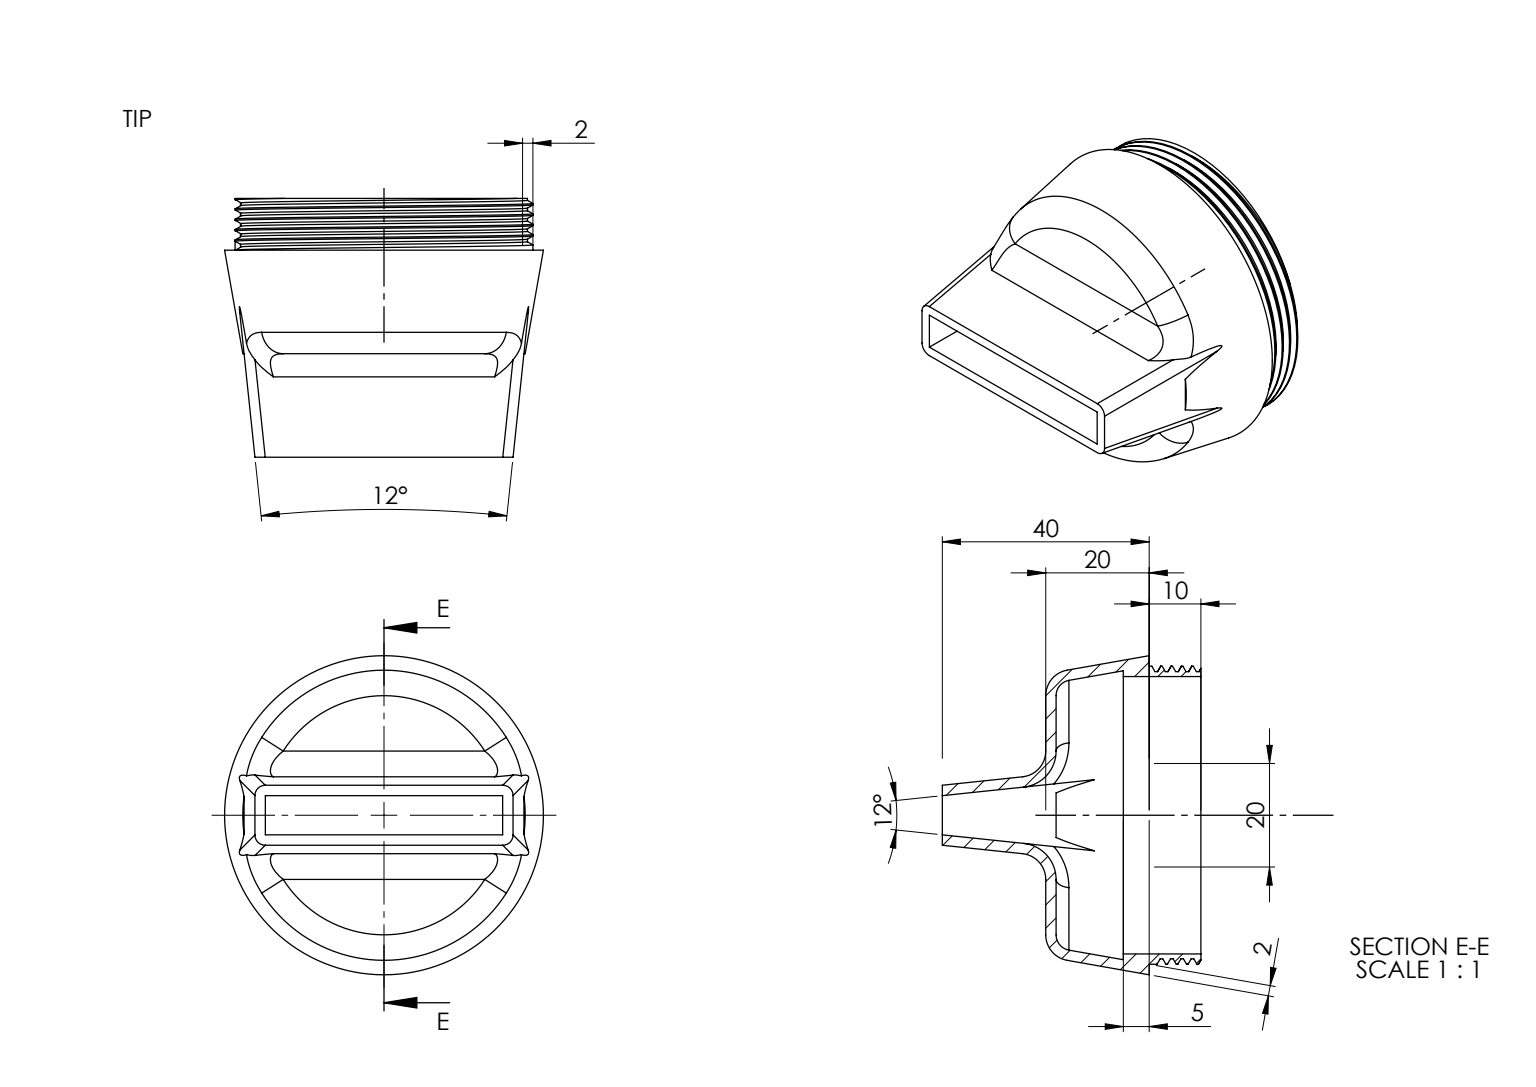
ISO-10303-21;
HEADER;
FILE_DESCRIPTION (('STEP AP214'),
    '1' );
FILE_NAME ('tip.step',
    '2026-10-04T13:31:42',
    ( '' ),
    ( '' ),
    'SwSTEP 2.0',
    'SolidWorks 2026',
    '' );
FILE_SCHEMA (( 'AUTOMOTIVE_DESIGN' ));
ENDSEC;

DATA;
#60=CARTESIAN_POINT ( 'NONE',  ( -8.571926809382608425, 26.38167802310805854, 144.4750000027312069 ) ) ;
#72=( BOUNDED_CURVE ( )  B_SPLINE_CURVE ( 2, ( #135553, #193227, #149715, #197225, #132546, #194235, #55701, #58687, #117374, #179071, #182049 ),
 .UNSPECIFIED., .F., .T. ) 
 B_SPLINE_CURVE_WITH_KNOTS ( ( 3, 2, 2, 2, 2, 3 ),
 ( 0.1000000000000000888, 0.1200000000000001343, 0.1400000000000001799, 0.1600000000000001976, 0.1800000000000002431, 0.2000000000000001776 ),
 .UNSPECIFIED. ) 
 CURVE ( )  GEOMETRIC_REPRESENTATION_ITEM ( )  RATIONAL_B_SPLINE_CURVE ( ( 0.9999999999999997780, 0.9510565162951537532, 1.000000000000000000, 0.9510565162951535312, 1.000000000000000000, 0.9510565162951535312, 1.000000000000000000, 0.9510565162951535312, 1.000000000000000000, 0.9510565162951529761, 1.000000000000000444 ) ) 
 REPRESENTATION_ITEM ( '' )  );
#75=CARTESIAN_POINT ( 'NONE',  ( 27.73933785331498569, 2.768321779492822058E-14, 140.3750000027311842 ) ) ;
#93=CARTESIAN_POINT ( 'NONE',  ( 25.38276140623240096, 4.833717845876353891, 166.7901960806512136 ) ) ;
#101=CARTESIAN_POINT ( 'NONE',  ( 28.79475375365586132, 2.781246896534039337E-14, 145.2656553485623760 ) ) ;
#142=CARTESIAN_POINT ( 'NONE',  ( 1.955436445514509014, -27.87083070116242567, 139.9999999999999716 ) ) ;
#200=CARTESIAN_POINT ( 'NONE',  ( -23.31738231874055245, -16.94106989632524574, 144.1999999999999886 ) ) ;
#216=CARTESIAN_POINT ( 'NONE',  ( 23.29544513554940011, 16.92513159979228021, 143.4656553485623647 ) ) ;
#218=CARTESIAN_POINT ( 'NONE',  ( 19.76513836702801186, -12.18681594171306237, 170.0000000000000000 ) ) ;
#300=ORIENTED_EDGE ( 'NONE', *, *, #146255, .F. ) ;
#338=CARTESIAN_POINT ( 'NONE',  ( -30.82560697742735911, 2.051108057200722688E-14, 150.0000000000000000 ) ) ;
#460=CARTESIAN_POINT ( 'NONE',  ( 27.74036206688027661, 1.797278685356906491, 140.0000000000000000 ) ) ;
#486=CARTESIAN_POINT ( 'NONE',  ( 21.65431292632186100, -8.856125861401146437, 168.9593721673316793 ) ) ;
#544=CARTESIAN_POINT ( 'NONE',  ( -17.14385361876520619, 23.59649016807275856, 143.0750000027311444 ) ) ;
#548=CARTESIAN_POINT ( 'NONE',  ( -17.14385361876520264, -23.59649016807271593, 143.6750000027311671 ) ) ;
#553=DIRECTION ( 'NONE',  ( -0.000000000000000000, -0.000000000000000000, -1.000000000000000000 ) ) ;
#581=CARTESIAN_POINT ( 'NONE',  ( -24.42783677680811749, -12.30119602009749613, 169.8172178118632587 ) ) ;
#601=CARTESIAN_POINT ( 'NONE',  ( -17.79613651744293890, -24.49428055684528260, 140.5656553485623022 ) ) ;
#766=CARTESIAN_POINT ( 'NONE',  ( -24.20533859822809220, -9.236745700548658178, 166.4300890397318540 ) ) ;
#827=CARTESIAN_POINT ( 'NONE',  ( -23.91168844458654164, 8.792376985861425354, 168.9858545422794975 ) ) ;
#852=ORIENTED_EDGE ( 'NONE', *, *, #79706, .T. ) ;
#865=DIRECTION ( 'NONE',  ( -1.000000000000000000, 0.000000000000000000, 0.000000000000000000 ) ) ;
#891=CARTESIAN_POINT ( 'NONE',  ( 1.784210473542230573E-15, -29.16686587814331588, 147.3750000027311842 ) ) ;
#978=CARTESIAN_POINT ( 'NONE',  ( -25.28179187713397269, -11.97099003546684415, 166.1915553108511290 ) ) ;
#1014=CARTESIAN_POINT ( 'NONE',  ( -3.573655867282028392E-15, 2.428612866367529932E-14, 139.9999999999999716 ) ) ;
#1025=( NAMED_UNIT ( * ) PLANE_ANGLE_UNIT ( ) SI_UNIT ( $, .RADIAN. ) );
#1054=CARTESIAN_POINT ( 'NONE',  ( 27.73933785331498214, 9.013057229001095294, 145.9750000027311785 ) ) ;
#1061=CARTESIAN_POINT ( 'NONE',  ( 20.69372460268722236, -10.84650605405300539, 168.1714143675833668 ) ) ;
#1191=CARTESIAN_POINT ( 'NONE',  ( -17.81289503416611808, 24.51734667627700404, 143.7000000000000171 ) ) ;
#1204=CARTESIAN_POINT ( 'NONE',  ( 24.18299921989822820, -12.77492350451709235, 169.7822198539309966 ) ) ;
#1210=CARTESIAN_POINT ( 'NONE',  ( 21.34799762026584702, -10.44447989802409893, 170.3878604776606096 ) ) ;
#1214=CARTESIAN_POINT ( 'NONE',  ( -24.74823625077143774, 6.005039613785521091, 168.8763313249075964 ) ) ;
#1293=ORIENTED_EDGE ( 'NONE', *, *, #171007, .T. ) ;
#1305=CARTESIAN_POINT ( 'NONE',  ( 1.784210473542230573E-15, -29.16686587814331588, 147.8750000027311273 ) ) ;
#1326=CARTESIAN_POINT ( 'NONE',  ( -25.66012929990208136, -7.783344152590475851, 170.2244316400881701 ) ) ;
#1457=CARTESIAN_POINT ( 'NONE',  ( 27.38287604894768634, -4.524378969001820572, 139.9999999999999716 ) ) ;
#1479=AXIS2_PLACEMENT_3D ( 'NONE', #153769, #105284, #28475 ) ;
#1535=EDGE_CURVE ( 'NONE', #136214, #11685, #2227, .T. ) ;
#1547=CARTESIAN_POINT ( 'NONE',  ( 22.44159573604009239, 16.30477369853692693, 148.5750000027312012 ) ) ;
#1657=VECTOR ( 'NONE', #198444, 1000.000000000000000 ) ;
#1779=ADVANCED_FACE ( 'NONE', ( #62900 ), #3223, .T. ) ;
#1806=CARTESIAN_POINT ( 'NONE',  ( -8.898068258721474777, 27.38543819252877043, 145.5843446569000150 ) ) ;
#1831=CARTESIAN_POINT ( 'NONE',  ( -21.70479006154311108, 8.695791278452229989, 169.0563666577074287 ) ) ;
#1897=CARTESIAN_POINT ( 'NONE',  ( 8.571926809382603096, -26.38167802310801235, 139.4750000027311785 ) ) ;
#2037=PLANE ( 'NONE',  #40540 ) ;
#2061=CARTESIAN_POINT ( 'NONE',  ( -27.73933785331498925, 2.428612866367529932E-14, 140.8750000027311842 ) ) ;
#2068=FACE_OUTER_BOUND ( 'NONE', #96703, .T. ) ;
#2128=EDGE_CURVE ( 'NONE', #35378, #51307, #33569, .T. ) ;
#2143=EDGE_CURVE ( 'NONE', #18425, #66087, #76032, .T. ) ;
#2198=CARTESIAN_POINT ( 'NONE',  ( -5.429308488886486681E-15, 30.30510711980690175, 143.4999999999999432 ) ) ;
#2211=CARTESIAN_POINT ( 'NONE',  ( 25.86526910843990379, -7.630673861715740358, 173.3900163844746771 ) ) ;
#2227=LINE ( 'NONE', #170091, #198734 ) ;
#2291=CARTESIAN_POINT ( 'NONE',  ( -5.429308488886486681E-15, 30.30510711980690175, 147.7500000054623683 ) ) ;
#2429=AXIS2_PLACEMENT_3D ( 'NONE', #118960, #58273, #120921 ) ;
#2459=CARTESIAN_POINT ( 'NONE',  ( 18.35237201590196676, -20.87933371662905202, 140.0000000000000284 ) ) ;
#2548=CARTESIAN_POINT ( 'NONE',  ( -28.79475375365586842, 2.428612866367529932E-14, 155.0000000000000000 ) ) ;
#2631=B_SPLINE_CURVE_WITH_KNOTS ( 'NONE', 3,
 ( #184968, #62602, #138458, #91937, #183979, #170795, #107119, #153630 ),
 .UNSPECIFIED., .F., .F.,
 ( 4, 2, 2, 4 ),
 ( 2.244678719545345876E-07, 0.002115167047690978165, 0.004230109627510002419, 0.008459994787147971998 ),
 .UNSPECIFIED. ) ;
#2717=CARTESIAN_POINT ( 'NONE',  ( -24.81835880841865816, 6.052260367207988878, 168.4265213779230521 ) ) ;
#2738=CARTESIAN_POINT ( 'NONE',  ( 3.796749449783271668, 28.08088322626615607, 140.0000000000000000 ) ) ;
#2773=VERTEX_POINT ( 'NONE', #175067 ) ;
#2802=CARTESIAN_POINT ( 'NONE',  ( -28.79475375365603185, 9.355982642739006039, 145.8843446568999980 ) ) ;
#2828=CARTESIAN_POINT ( 'NONE',  ( -23.14613071126281341, 10.96668486446900381, 168.1016194467972014 ) ) ;
#2848=ORIENTED_EDGE ( 'NONE', *, *, #192109, .F. ) ;
#2894=CARTESIAN_POINT ( 'NONE',  ( 22.44159573604009239, 16.30477369853692693, 142.0750000027311728 ) ) ;
#3058=CARTESIAN_POINT ( 'NONE',  ( -27.60098488412532802, 5.861468761074982936, 164.8187539380761564 ) ) ;
#3206=CARTESIAN_POINT ( 'NONE',  ( 21.35462415990438245, -10.43496131973849117, 170.3924512066481043 ) ) ;
#3212=CARTESIAN_POINT ( 'NONE',  ( 21.97181142354051531, -8.379174292515184419, 172.0076905927031419 ) ) ;
#3223=CYLINDRICAL_SURFACE ( 'NONE', #72438, 28.79475375365586487 ) ;
#3266=( BOUNDED_CURVE ( )  B_SPLINE_CURVE ( 2, ( #65961, #49812, #125658, #82104, #110478, #172161, #127632, #112467, #5279, #66961, #128622, #190315, #32661, #3301, #175144, #1305, #62984, #124663, #18490, #64973, #94315, #155993, #17489, #140818, #95307, #156991, #102301, #85114, #83118, #38634, #84113, #176152, #39622, #146798, #178157, #101282, #37622, #115472, #36612, #8291, #192317, #6278, #161969, #7275, #116468, #163990, #162972, #193319, #145792, #25487, #68959, #130621, #147818, #194326, #55794, #179164, #40632, #24477, #99284, #23465, #86127, #117466, #9304, #195326, #70970, #132638, #21457, #53797, #118480, #87129, #148814, #131635, #10304, #71961, #133635, #177161, #100291, #54793, #56806, #69969, #67956, #98268, #191306, #22465, #144795, #129611, #159970, #52782, #114451, #160971, #75, #166972, #13284, #137606, #72980 ),
 .UNSPECIFIED., .F., .F. ) 
 B_SPLINE_CURVE_WITH_KNOTS ( ( 3, 2, 2, 2, 2, 2, 2, 2, 2, 2, 2, 2, 2, 2, 2, 2, 2, 2, 2, 2, 2, 2, 2, 2, 2, 2, 2, 2, 2, 2, 2, 2, 2, 2, 2, 2, 2, 2, 2, 2, 2, 2, 2, 2, 2, 2, 2, 3 ),
 ( 0.000000000000000000, 0.02000000000000000042, 0.04000000000000000083, 0.05999999999999999778, 0.08000000000000000167, 0.1000000000000000056, 0.1199999999999999956, 0.1400000000000000133, 0.1600000000000000033, 0.1799999999999999933, 0.2000000000000000111, 0.2200000000000000011, 0.2399999999999999911, 0.2600000000000000089, 0.2800000000000000266, 0.2999999999999999889, 0.3200000000000000067, 0.3400000000000000244, 0.3599999999999999867, 0.3800000000000000044, 0.4000000000000000222, 0.4199999999999999845, 0.4400000000000000022, 0.4599999999999999645, 0.4799999999999999822, 0.5000000000000000000, 0.5200000000000000178, 0.5400000000000000355, 0.5600000000000000533, 0.5800000000000000711, 0.5999999999999999778, 0.6199999999999999956, 0.6400000000000000133, 0.6600000000000000311, 0.6800000000000000488, 0.6999999999999999556, 0.7199999999999999734, 0.7399999999999999911, 0.7600000000000000089, 0.7800000000000000266, 0.8000000000000000444, 0.8199999999999999512, 0.8399999999999999689, 0.8599999999999999867, 0.8800000000000000044, 0.9000000000000000222, 0.9199999999999999289, 0.9374174419963630100 ),
 .UNSPECIFIED. ) 
 CURVE ( )  GEOMETRIC_REPRESENTATION_ITEM ( )  RATIONAL_B_SPLINE_CURVE ( ( 1.000000000000000000, 0.9510565162951535312, 1.000000000000000000, 0.9510565162951535312, 1.000000000000000000, 0.9510565162951535312, 1.000000000000000000, 0.9510565162951535312, 1.000000000000000000, 0.9510565162951535312, 1.000000000000000000, 0.9510565162951535312, 1.000000000000000000, 0.9510565162951535312, 1.000000000000000000, 0.9510565162951535312, 1.000000000000000000, 0.9510565162951535312, 1.000000000000000000, 0.9510565162951535312, 1.000000000000000000, 0.9510565162951535312, 1.000000000000000000, 0.9510565162951535312, 1.000000000000000000, 0.9510565162951535312, 1.000000000000000000, 0.9510565162951535312, 1.000000000000000000, 0.9510565162951535312, 1.000000000000000000, 0.9510565162951535312, 1.000000000000000000, 0.9510565162951535312, 1.000000000000000000, 0.9510565162951535312, 1.000000000000000000, 0.9510565162951535312, 1.000000000000000000, 0.9510565162951535312, 1.000000000000000000, 0.9510565162951535312, 1.000000000000000000, 0.9510565162951535312, 1.000000000000000000, 0.9510565162951535312, 1.000000000000000000, 0.9510565162951535312, 1.000000000000000000, 0.9510565162951535312, 1.000000000000000000, 0.9510565162951535312, 1.000000000000000000, 0.9510565162951535312, 1.000000000000000000, 0.9510565162951535312, 1.000000000000000000, 0.9510565162951535312, 1.000000000000000000, 0.9510565162951535312, 1.000000000000000000, 0.9510565162951535312, 1.000000000000000000, 0.9510565162951535312, 1.000000000000000000, 0.9510565162951535312, 1.000000000000000000, 0.9510565162951535312, 1.000000000000000000, 0.9510565162951535312, 1.000000000000000000, 0.9510565162951535312, 1.000000000000000000, 0.9510565162951535312, 1.000000000000000000, 0.9510565162951535312, 1.000000000000000000, 0.9510565162951535312, 1.000000000000000000, 0.9510565162951535312, 1.000000000000000000, 0.9510565162951535312, 1.000000000000000000, 0.9510565162951535312, 1.000000000000000000, 0.9510565162951535312, 1.000000000000000000, 0.9510565162951535312, 1.000000000000000000, 0.9510565162951535312, 1.000000000000000000, 0.9510565162951535312, 1.000000000000000000, 0.9573764855735448220, 0.9889922301674822780 ) ) 
 REPRESENTATION_ITEM ( '' )  );
#3280=AXIS2_PLACEMENT_3D ( 'NONE', #188040, #19180, #186051 ) ;
#3301=CARTESIAN_POINT ( 'NONE',  ( 17.14385361876520264, -23.59649016807270883, 148.0750000027312012 ) ) ;
#3499=ORIENTED_EDGE ( 'NONE', *, *, #136656, .T. ) ;
#3562=DIRECTION ( 'NONE',  ( 0.000000000000000000, 0.000000000000000000, 1.000000000000000000 ) ) ;
#3644=ORIENTED_EDGE ( 'NONE', *, *, #152669, .F. ) ;
#3723=CARTESIAN_POINT ( 'NONE',  ( 27.89898386898346772, 7.496946767014385671, 160.9847407629968359 ) ) ;
#3810=CARTESIAN_POINT ( 'NONE',  ( -21.92083080610932910, 6.374575339255513562, 171.4095429173270020 ) ) ;
#3876=CARTESIAN_POINT ( 'NONE',  ( -22.44159573604010305, 16.30477369853692338, 149.1750000027311671 ) ) ;
#3915=FACE_OUTER_BOUND ( 'NONE', #114573, .T. ) ;
#4005=CARTESIAN_POINT ( 'NONE',  ( -5.427562675786936573E-15, 30.27659582821221207, 149.4843446568999923 ) ) ;
#4018=ORIENTED_EDGE ( 'NONE', *, *, #130470, .T. ) ;
#4039=EDGE_CURVE ( 'NONE', #135144, #122542, #15177, .T. ) ;
#4040=CARTESIAN_POINT ( 'NONE',  ( -27.18966431762778058, 4.276553394869404556, 168.7322077152510928 ) ) ;
#4069=EDGE_CURVE ( 'NONE', #163981, #33758, #46734, .T. ) ;
#4102=CARTESIAN_POINT ( 'NONE',  ( 24.06756124613832171, 8.142616467494580235, 169.4332804344653312 ) ) ;
#4186=CARTESIAN_POINT ( 'NONE',  ( 24.05407591190871130, -13.01182159662947413, 169.7785964492052244 ) ) ;
#4193=CARTESIAN_POINT ( 'NONE',  ( 21.96405779611664855, -8.831116573701658368, 171.4809137887048962 ) ) ;
#4268=CARTESIAN_POINT ( 'NONE',  ( -28.82186960331499392, 9.364793116373565596, 148.1500000054624024 ) ) ;
#4511=FACE_OUTER_BOUND ( 'NONE', #127744, .T. ) ;
#4514=CARTESIAN_POINT ( 'NONE',  ( -24.43796699203916845, 7.704306453272268485, 171.8420650787743966 ) ) ;
#4536=CARTESIAN_POINT ( 'NONE',  ( 25.90244409532897762, -6.509810826857640897, 161.8457455760359949 ) ) ;
#4658=FACE_OUTER_BOUND ( 'NONE', #43791, .T. ) ;
#4707=CARTESIAN_POINT ( 'NONE',  ( 27.96890437653522099, 7.184031643483238305, 161.0522725792803556 ) ) ;
#4734=CARTESIAN_POINT ( 'NONE',  ( -22.77340942535178314, 12.66915129224426906, 165.5704402759699008 ) ) ;
#4840=AXIS2_PLACEMENT_3D ( 'NONE', #167237, #77188, #47861 ) ;
#4847=VECTOR ( 'NONE', #61893, 1000.000000000000000 ) ;
#4861=CARTESIAN_POINT ( 'NONE',  ( 21.96329795405619834, 8.386426352705248277, 172.0132153625898468 ) ) ;
#4881=CARTESIAN_POINT ( 'NONE',  ( 27.77694149905228471, -7.633451960439483486, 161.4496143021105183 ) ) ;
#4950=CARTESIAN_POINT ( 'NONE',  ( -26.58496454516998853, -7.626754437231455519, 167.9682100371138915 ) ) ;
#4962=CARTESIAN_POINT ( 'NONE',  ( -3.573655867282028392E-15, 2.428612866367529932E-14, 155.0000000000000000 ) ) ;
#5031=CARTESIAN_POINT ( 'NONE',  ( -27.39399371936807270, 5.109217719441145000, 166.7881433183807189 ) ) ;
#5095=CARTESIAN_POINT ( 'NONE',  ( 24.29042230868054020, 8.936166115089967832, 166.5611006352800132 ) ) ;
#5182=CARTESIAN_POINT ( 'NONE',  ( 25.11239783071230747, -12.35465959874983533, 166.1131185557732124 ) ) ;
#5202=CARTESIAN_POINT ( 'NONE',  ( -23.22614267028769319, -5.670187745555518077, 172.0618673401326646 ) ) ;
#5206=CARTESIAN_POINT ( 'NONE',  ( 22.44159573604009239, 16.30477369853692693, 140.0750000027311728 ) ) ;
#5263=CARTESIAN_POINT ( 'NONE',  ( 1.784210473542230573E-15, -29.16686587814331588, 141.8750000027311842 ) ) ;
#5264=CARTESIAN_POINT ( 'NONE',  ( 17.81289503416611453, -24.51734667627695785, 146.9500000054623570 ) ) ;
#5279=CARTESIAN_POINT ( 'NONE',  ( 22.44159573604009239, 16.30477369853692693, 148.5750000027312012 ) ) ;
#5325=CARTESIAN_POINT ( 'NONE',  ( -23.29544513554941076, 16.92513159979227666, 148.0656553485623590 ) ) ;
#5436=DIRECTION ( 'NONE',  ( 1.000000000000000000, 0.000000000000000000, 0.000000000000000000 ) ) ;
#5520=CARTESIAN_POINT ( 'NONE',  ( -23.58955696227030074, 7.613471476246056469, 172.7063021553927911 ) ) ;
#5700=CARTESIAN_POINT ( 'NONE',  ( 28.79475375365586132, 2.781246896534039337E-14, 146.9843446568999923 ) ) ;
#5712=CARTESIAN_POINT ( 'NONE',  ( 22.12969251635687229, 16.97230210225939118, 139.9999999999999432 ) ) ;
#5739=EDGE_CURVE ( 'NONE', #109599, #48040, #198809, .T. ) ;
#5767=SHAPE_DEFINITION_REPRESENTATION ( #167934, #112845 ) ;
#5840=CARTESIAN_POINT ( 'NONE',  ( -21.98685479826777112, -13.98560643873833875, 165.5209445330007441 ) ) ;
#5903=CARTESIAN_POINT ( 'NONE',  ( 8.898068258721473001, -27.38543819252872069, 146.8656553485623704 ) ) ;
#6085=CARTESIAN_POINT ( 'NONE',  ( -27.91252812235343228, -7.473505457753331527, 160.9450913315372986 ) ) ;
#6149=B_SPLINE_CURVE_WITH_KNOTS ( 'NONE', 3,
 ( #55086, #194613, #23762, #131931, #118773, #56085, #85411, #180461, #11605, #71262, #10597, #8588, #165274, #26768 ),
 .UNSPECIFIED., .F., .F.,
 ( 4, 2, 2, 2, 2, 2, 4 ),
 ( 0.000000000000000000, 0.002096066633256107002, 0.003144099949884150962, 0.004192133266512195790, 0.006288199899768283710, 0.007336233216396328971, 0.008384266533024374232 ),
 .UNSPECIFIED. ) ;
#6208=CARTESIAN_POINT ( 'NONE',  ( -22.44159573604009950, -16.30477369853688430, 141.0750000027311728 ) ) ;
#6264=CARTESIAN_POINT ( 'NONE',  ( -28.82186960331499392, -9.364793116373526516, 146.3500000054623627 ) ) ;
#6278=CARTESIAN_POINT ( 'NONE',  ( -27.73933785331498925, 9.013057229001088189, 145.2750000027311899 ) ) ;
#6348=CARTESIAN_POINT ( 'NONE',  ( -25.55222625260934066, 11.31436996698904629, 166.3494238031456405 ) ) ;
#6389=CARTESIAN_POINT ( 'NONE',  ( 23.64874990377914799, 15.04272038711346049, 165.8682408883346397 ) ) ;
#6412=VECTOR ( 'NONE', #39028, 1000.000000000000114 ) ;
#6426=CARTESIAN_POINT ( 'NONE',  ( -17.79613651744293890, -24.49428055684527550, 144.2843446568999752 ) ) ;
#6431=CARTESIAN_POINT ( 'NONE',  ( -5.427562675786936573E-15, 30.27659582821221207, 145.7656553485623192 ) ) ;
#6543=CARTESIAN_POINT ( 'NONE',  ( -3.573655867282028392E-15, 2.428612866367529932E-14, 150.0000000000000000 ) ) ;
#6732=CARTESIAN_POINT ( 'NONE',  ( -24.66673051387562410, 7.254129419879411955, 167.4978569920363611 ) ) ;
#6753=CARTESIAN_POINT ( 'NONE',  ( -19.49401214000074489, -12.39993551617566325, 167.9999999999999716 ) ) ;
#6792=CARTESIAN_POINT ( 'NONE',  ( 21.73861122199297569, -5.803778330637474170, 172.6157762304496828 ) ) ;
#6995=DIRECTION ( 'NONE',  ( 0.000000000000000000, 0.000000000000000000, -1.000000000000000000 ) ) ;
#7093=CARTESIAN_POINT ( 'NONE',  ( 23.84827716990778512, 9.022217638662837658, 168.8513102586128127 ) ) ;
#7206=CARTESIAN_POINT ( 'NONE',  ( 17.14385361876520264, -23.59649016807270883, 141.5750000027311728 ) ) ;
#7240=ORIENTED_EDGE ( 'NONE', *, *, #34091, .F. ) ;
#7259=CARTESIAN_POINT ( 'NONE',  ( 17.14385361876520264, 23.59649016807275856, 140.6750000027311387 ) ) ;
#7260=CARTESIAN_POINT ( 'NONE',  ( 17.81289503416610742, 24.51734667627700404, 141.5500000054623797 ) ) ;
#7265=B_SPLINE_CURVE_WITH_KNOTS ( 'NONE', 3,
 ( #180380, #153727, #148025, #9514, #87340, #15223, #57015, #76882 ),
 .UNSPECIFIED., .F., .F.,
 ( 4, 2, 2, 4 ),
 ( 0.01263483034531142669, 0.01686471550494896693, 0.01897965808476773791, 0.02109460066458650543 ),
 .UNSPECIFIED. ) ;
#7275=CARTESIAN_POINT ( 'NONE',  ( -17.14385361876520975, 23.59649016807275856, 145.0750000027311444 ) ) ;
#7344=CARTESIAN_POINT ( 'NONE',  ( -25.75939503182791768, 8.559839547494505041, 171.7912139782359588 ) ) ;
#7388=CARTESIAN_POINT ( 'NONE',  ( 25.66129429279843066, 9.008087060820804126, 171.3163768196993431 ) ) ;
#7423=CARTESIAN_POINT ( 'NONE',  ( -29.15849868437705439, -10.00000000000000000, 150.0000000000000000 ) ) ;
#7486=CARTESIAN_POINT ( 'NONE',  ( -24.02706313830240603, 14.44797190822832711, 165.8682408883346113 ) ) ;
#7543=DIRECTION ( 'NONE',  ( 1.000000000000000000, 0.000000000000000000, 0.000000000000000000 ) ) ;
#7551=VECTOR ( 'NONE', #58066, 1000.000000000000114 ) ;
#7692=EDGE_CURVE ( 'NONE', #11205, #144964, #15531, .T. ) ;
#7705=CARTESIAN_POINT ( 'NONE',  ( 26.82869043059737635, 7.693057566823323867, 166.5358880480721098 ) ) ;
#7746=CARTESIAN_POINT ( 'NONE',  ( 17.14385361876520264, -23.59649016807271238, 148.0750000027311728 ) ) ;
#7754=CARTESIAN_POINT ( 'NONE',  ( -23.19706360625325559, -11.80427776162532538, 165.7059442611694067 ) ) ;
#7758=EDGE_CURVE ( 'NONE', #162084, #62156, #27421, .T. ) ;
#7935=CARTESIAN_POINT ( 'NONE',  ( -19.49401214000077331, 12.39993551617566681, 167.9999999999999716 ) ) ;
#7951=DIRECTION ( 'NONE',  ( -0.000000000000000000, -0.000000000000000000, -1.000000000000000000 ) ) ;
#8045=COLOUR_RGB ( '', 0.72549020, 0.75294118, 0.79215686) ;
#8089=CARTESIAN_POINT ( 'NONE',  ( -27.96890437653549455, -7.184031643498222763, 161.0522725792576182 ) ) ;
#8109=CARTESIAN_POINT ( 'NONE',  ( -3.573655867282028392E-15, 2.428612866367529932E-14, 164.9999999999999716 ) ) ;
#8220=CARTESIAN_POINT ( 'NONE',  ( 17.14385361876520264, 23.59649016807275856, 140.1750000027311671 ) ) ;
#8271=ORIENTED_EDGE ( 'NONE', *, *, #74210, .F. ) ;
#8277=CARTESIAN_POINT ( 'NONE',  ( -27.73933785331498925, 2.428612866367529932E-14, 141.3750000027311842 ) ) ;
#8278=CARTESIAN_POINT ( 'NONE',  ( -17.14385361876520619, 23.59649016807275856, 148.5750000027311444 ) ) ;
#8291=CARTESIAN_POINT ( 'NONE',  ( -27.73933785331498925, -9.013057229001049109, 145.4750000027311785 ) ) ;
#8360=CARTESIAN_POINT ( 'NONE',  ( 24.81835718235489807, 6.052279806424484931, 168.4265042179603142 ) ) ;
#8364=CARTESIAN_POINT ( 'NONE',  ( -19.49401214000077687, 12.39993551617566681, 169.9999999999999716 ) ) ;
#8408=CARTESIAN_POINT ( 'NONE',  ( 24.18299921989880730, 12.77492350451764125, 169.7822198539310250 ) ) ;
#8421=CARTESIAN_POINT ( 'NONE',  ( 8.906447517083050158, 27.41122689804195645, 147.4000000000000057 ) ) ;
#8444=PLANE ( 'NONE',  #103538 ) ;
#8447=CARTESIAN_POINT ( 'NONE',  ( 17.79613651744294245, -24.49428055684527195, 144.6843446569000093 ) ) ;
#8452=CARTESIAN_POINT ( 'NONE',  ( 17.79613651744293534, 24.49428055684532524, 145.5656553485623590 ) ) ;
#8485=CYLINDRICAL_SURFACE ( 'NONE', #27165, 28.79475375365586487 ) ;
#8497=ORIENTED_EDGE ( 'NONE', *, *, #57626, .F. ) ;
#8565=CARTESIAN_POINT ( 'NONE',  ( -21.93208748025632460, -6.437649280788580342, 171.3046185016227412 ) ) ;
#8588=CARTESIAN_POINT ( 'NONE',  ( 26.47570757000580954, 8.223507928023316538, 167.6031463996532409 ) ) ;
#8589=FACE_BOUND ( 'NONE', #92313, .T. ) ;
#8770=FACE_OUTER_BOUND ( 'NONE', #32591, .T. ) ;
#8776=CARTESIAN_POINT ( 'NONE',  ( -24.29042230868021690, -8.936166115090793838, 166.5611006352801553 ) ) ;
#8858=DIRECTION ( 'NONE',  ( -1.000000000000000000, 0.000000000000000000, 0.000000000000000000 ) ) ;
#8860=CARTESIAN_POINT ( 'NONE',  ( -26.03370437638687918, 6.875205692009823011, 160.5968874236874910 ) ) ;
#9066=CARTESIAN_POINT ( 'NONE',  ( 30.82560697742735201, 2.428612866367529932E-14, 150.0000000000000000 ) ) ;
#9106=CARTESIAN_POINT ( 'NONE',  ( -27.46944729266723328, -7.746537029273099506, 162.9576794167586797 ) ) ;
#9120=CARTESIAN_POINT ( 'NONE',  ( 21.56952297831559662, 5.557039098534931831, 173.4609804364286276 ) ) ;
#9229=CARTESIAN_POINT ( 'NONE',  ( -24.71161622716357087, -5.993525217005509553, 168.9855167950506427 ) ) ;
#9233=CARTESIAN_POINT ( 'NONE',  ( -27.73933785331498925, 2.428612866367529932E-14, 142.8750000027311842 ) ) ;
#9289=CARTESIAN_POINT ( 'NONE',  ( -8.571926809382608425, 26.38167802310805854, 140.9750000027312069 ) ) ;
#9290=CARTESIAN_POINT ( 'NONE',  ( -28.82186960331499392, 9.364793116373565596, 140.1500000054623740 ) ) ;
#9294=VERTEX_POINT ( 'NONE', #179708 ) ;
#9304=CARTESIAN_POINT ( 'NONE',  ( -22.44159573604010305, 16.30477369853692338, 143.1750000027311671 ) ) ;
#9375=CARTESIAN_POINT ( 'NONE',  ( -21.51693143705273670, 10.15780255052816550, 170.5200780514257133 ) ) ;
#9426=CARTESIAN_POINT ( 'NONE',  ( -8.906447517083060816, 27.41122689804195645, 145.5999999999999943 ) ) ;
#9514=CARTESIAN_POINT ( 'NONE',  ( 27.39399371936806560, -5.109217719441128125, 166.7881433183806905 ) ) ;
#9585=CARTESIAN_POINT ( 'NONE',  ( 1.784210473542230573E-15, -29.16686587814331588, 145.3750000027311842 ) ) ;
#9710=ORIENTED_EDGE ( 'NONE', *, *, #103264, .F. ) ;
#9775=CARTESIAN_POINT ( 'NONE',  ( -8.571926809382608425, 26.38167802310805854, 146.9750000027311785 ) ) ;
#9818=CARTESIAN_POINT ( 'NONE',  ( 21.95653654802608301, -6.613221094984325532, 171.0358100525039902 ) ) ;
#9826=B_SPLINE_CURVE_WITH_KNOTS ( 'NONE', 3,
 ( #156724, #141542, #84833, #116192 ),
 .UNSPECIFIED., .F., .F.,
 ( 4, 4 ),
 ( 0.000000000000000000, 0.007966019813519142206 ),
 .UNSPECIFIED. ) ;
#9833=EDGE_CURVE ( 'NONE', #181866, #51216, #142632, .T. ) ;
#9922=CARTESIAN_POINT ( 'NONE',  ( 20.85011945226400698, 10.59319688750118083, 168.2343749380337954 ) ) ;
#9953=ORIENTED_EDGE ( 'NONE', *, *, #58299, .T. ) ;
#9956=CARTESIAN_POINT ( 'NONE',  ( -21.27520710526540526, 9.818903669220862440, 168.4804316999487241 ) ) ;
#9999=CARTESIAN_POINT ( 'NONE',  ( 24.95432927374997689, 4.974562764236792667, 190.0000000000000000 ) ) ;
#10034=EDGE_LOOP ( 'NONE', ( #88413, #29183, #24215, #173664, #173536, #22454 ) ) ;
#10107=CARTESIAN_POINT ( 'NONE',  ( -27.96784714409843886, -7.240004476342272177, 160.9788157999716702 ) ) ;
#10121=CARTESIAN_POINT ( 'NONE',  ( 24.10884208241212079, 5.471882726980997980, 173.8287385965645058 ) ) ;
#10230=DIRECTION ( 'NONE',  ( 0.000000000000000000, 0.000000000000000000, 1.000000000000000000 ) ) ;
#10291=CARTESIAN_POINT ( 'NONE',  ( 27.73933785331498569, 2.768321779492822058E-14, 147.8750000027311842 ) ) ;
#10294=DIRECTION ( 'NONE',  ( 0.000000000000000000, 0.000000000000000000, 1.000000000000000000 ) ) ;
#10304=CARTESIAN_POINT ( 'NONE',  ( 22.44159573604009594, -16.30477369853687364, 142.1750000027311671 ) ) ;
#10375=CARTESIAN_POINT ( 'NONE',  ( -25.34721418589319342, 10.09305078451843940, 170.5222919391071912 ) ) ;
#10429=CARTESIAN_POINT ( 'NONE',  ( -17.81289503416611808, 24.51734667627700404, 149.6999999999999602 ) ) ;
#10453=CARTESIAN_POINT ( 'NONE',  ( -21.38418241377624085, 5.438282248597754887, 174.2683007571264113 ) ) ;
#10508=EDGE_LOOP ( 'NONE', ( #119645, #128968, #130150, #120844, #135238 ) ) ;
#10586=CARTESIAN_POINT ( 'NONE',  ( 1.784210473542230573E-15, -29.16686587814331588, 147.3750000027311842 ) ) ;
#10597=CARTESIAN_POINT ( 'NONE',  ( 26.33867313280597600, 8.832717389288090359, 167.2809140985657450 ) ) ;
#10783=DIRECTION ( 'NONE',  ( -0.9945218953682734009, 0.000000000000000000, 0.1045284632676537068 ) ) ;
#10816=CARTESIAN_POINT ( 'NONE',  ( 24.85114155361846144, -5.582993631601040896, 168.8590791472286412 ) ) ;
#10845=VERTEX_POINT ( 'NONE', #35693 ) ;
#10990=VECTOR ( 'NONE', #185421, 1000.000000000000000 ) ;
#10997=CARTESIAN_POINT ( 'NONE',  ( 22.96528548301342809, 5.795830589372932273, 190.0000000000000000 ) ) ;
#11077=VECTOR ( 'NONE', #116212, 1000.000000000000000 ) ;
#11122=CARTESIAN_POINT ( 'NONE',  ( 21.96844466259091533, 7.174710485416647465, 170.3366942299255413 ) ) ;
#11203=AXIS2_PLACEMENT_3D ( 'NONE', #132403, #129381, #147580 ) ;
#11205=VERTEX_POINT ( 'NONE', #147882 ) ;
#11296=CARTESIAN_POINT ( 'NONE',  ( 1.993301997531345292E-15, -30.30510711980685912, 142.7500000054623683 ) ) ;
#11300=EDGE_LOOP ( 'NONE', ( #151816, #141478, #142273, #185841, #12704, #153179, #88489, #18190, #109187, #89708, #190461, #153880 ) ) ;
#11378=CARTESIAN_POINT ( 'NONE',  ( -25.80209238092448842, 7.370998251475262997, 174.5109820657625619 ) ) ;
#11435=CARTESIAN_POINT ( 'NONE',  ( 23.31738231874054890, -16.94106989632523508, 146.7999999999999829 ) ) ;
#11524=CARTESIAN_POINT ( 'NONE',  ( -3.573655867282028392E-15, 2.428612866367529932E-14, 150.0000000000000000 ) ) ;
#11581=PLANE ( 'NONE',  #81712 ) ;
#11594=CARTESIAN_POINT ( 'NONE',  ( 17.14385361876520264, -23.59649016807270883, 147.5750000027311728 ) ) ;
#11605=CARTESIAN_POINT ( 'NONE',  ( 26.00062938246248478, 10.06977165081871384, 166.7331697587469250 ) ) ;
#11685=VERTEX_POINT ( 'NONE', #105343 ) ;
#11764=AXIS2_PLACEMENT_3D ( 'NONE', #8109, #143619, #190143 ) ;
#11827=CARTESIAN_POINT ( 'NONE',  ( -19.83801684532646803, -12.12952959760830041, 169.9999999999999716 ) ) ;
#11963=CARTESIAN_POINT ( 'NONE',  ( -21.71408805923171315, 8.664832797227232319, 169.0754946983649916 ) ) ;
#11993=CARTESIAN_POINT ( 'NONE',  ( 1.988064558232696151E-15, -30.27659582821216588, 144.7656553485623476 ) ) ;
#12003=AXIS2_PLACEMENT_3D ( 'NONE', #72281, #70284, #134966 ) ;
#12018=AXIS2_PLACEMENT_3D ( 'NONE', #158362, #47218, #108876 ) ;
#12053=EDGE_LOOP ( 'NONE', ( #119024, #139035, #83954, #140369 ) ) ;
#12133=CARTESIAN_POINT ( 'NONE',  ( -17.14385361876520264, -23.59649016807271593, 145.1750000027311387 ) ) ;
#12145=AXIS2_PLACEMENT_3D ( 'NONE', #194799, #10783, #73458 ) ;
#12194=CARTESIAN_POINT ( 'NONE',  ( -17.79613651744294600, 24.49428055684532524, 141.9656553485623647 ) ) ;
#12211=ORIENTED_EDGE ( 'NONE', *, *, #124720, .T. ) ;
#12222=CARTESIAN_POINT ( 'NONE',  ( -27.95290315088902133, 7.353483241874900322, 160.8982923760598851 ) ) ;
#12295=CARTESIAN_POINT ( 'NONE',  ( -22.44159573604010305, 16.30477369853692338, 142.6750000027311671 ) ) ;
#12297=FACE_OUTER_BOUND ( 'NONE', #26675, .T. ) ;
#12349=ADVANCED_FACE ( 'NONE', ( #26301 ), #135008, .T. ) ;
#12377=CARTESIAN_POINT ( 'NONE',  ( -7.018946318601956058, -27.29839631544761502, 139.9999999999999716 ) ) ;
#12419=CARTESIAN_POINT ( 'NONE',  ( 21.56952297831559662, 7.512152360717371913, 173.9007003117368981 ) ) ;
#12433=CARTESIAN_POINT ( 'NONE',  ( -28.82186960331499392, -9.364793116373526516, 146.1000000000000227 ) ) ;
#12448=CARTESIAN_POINT ( 'NONE',  ( 24.44405923433062355, -13.71792739260136607, 165.9118100595188707 ) ) ;
#12530=CARTESIAN_POINT ( 'NONE',  ( -24.10884208241212079, -5.471882726981282197, 173.8287385965643637 ) ) ;
#12567=CARTESIAN_POINT ( 'NONE',  ( -20.61165082012731986, -10.97245752705834043, 168.1443239908791440 ) ) ;
#12581=CARTESIAN_POINT ( 'NONE',  ( 8.571926809382597767, 26.38167802310806209, 146.2750000027311899 ) ) ;
#12704=ORIENTED_EDGE ( 'NONE', *, *, #122987, .T. ) ;
#12716=CARTESIAN_POINT ( 'NONE',  ( 19.80295450558173442, -12.05995242899444619, 167.9999999999999716 ) ) ;
#12770=CARTESIAN_POINT ( 'NONE',  ( -5.359611314223446995E-15, 29.16686587814335496, 142.8750000027311842 ) ) ;
#12810=CARTESIAN_POINT ( 'NONE',  ( -21.96844466259036111, -8.667631922774113207, 171.6690673070920354 ) ) ;
#12945=CARTESIAN_POINT ( 'NONE',  ( -21.96434091948370337, 6.687777057363587296, 170.9277123045939106 ) ) ;
#12998=EDGE_CURVE ( 'NONE', #189536, #105726, #146730, .T. ) ;
#13032=CARTESIAN_POINT ( 'NONE',  ( -8.898068258721467672, -27.38543819252872069, 146.3843446568999980 ) ) ;
#13079=B_SPLINE_CURVE_WITH_KNOTS ( 'NONE', 3,
 ( #147619, #193121, #162772, #86933, #116269, #176967, #9106, #191119, #133437, #39427, #70773, #192116, #24281, #118282, #6085, #178964, #99088, #132442, #148616, #164787, #10107, #8089, #103106, #179973, #114253, #194133, #55596, #68760 ),
 .UNSPECIFIED., .F., .F.,
 ( 4, 2, 2, 2, 2, 2, 2, 2, 2, 2, 2, 2, 2, 4 ),
 ( 0.000000000000000000, 0.002181393419090842979, 0.004362786838181685958, 0.005453483547727107014, 0.006544180257272528070, 0.006816854434658824353, 0.007089528612045118902, 0.007225865700738303039, 0.007294034245084918960, 0.007362202789431534881, 0.007498539878124766724, 0.007634876966818000300, 0.008180225321591003129, 0.008725573676364006825 ),
 .UNSPECIFIED. ) ;
#13090=CARTESIAN_POINT ( 'NONE',  ( -28.79475375365586842, 2.428612866367529932E-14, 141.9843446568999923 ) ) ;
#13109=CARTESIAN_POINT ( 'NONE',  ( 19.49401214000076621, 12.39993551617566681, 169.9999999999999716 ) ) ;
#13115=CARTESIAN_POINT ( 'NONE',  ( -5.359611314223446995E-15, 29.16686587814335496, 146.3750000027311842 ) ) ;
#13155=PLANE ( 'NONE',  #56380 ) ;
#13158=DIRECTION ( 'NONE',  ( 1.000000000000000000, 0.000000000000000000, 0.000000000000000000 ) ) ;
#13191=EDGE_CURVE ( 'NONE', #131044, #61621, #118465, .T. ) ;
#13216=FACE_OUTER_BOUND ( 'NONE', #165968, .T. ) ;
#13273=CARTESIAN_POINT ( 'NONE',  ( 17.14385361876520264, 23.59649016807275856, 142.1750000027311671 ) ) ;
#13284=CARTESIAN_POINT ( 'NONE',  ( 22.44159573604009594, -16.30477369853687364, 140.1750000027311955 ) ) ;
#13306=CARTESIAN_POINT ( 'NONE',  ( 8.898068258721473001, -27.38543819252872069, 140.5843446569000150 ) ) ;
#13350=CARTESIAN_POINT ( 'NONE',  ( -21.56952297831560372, 7.512152360717371913, 173.9007003117368981 ) ) ;
#13405=CARTESIAN_POINT ( 'NONE',  ( -28.82186960331499037, 2.428612866367529932E-14, 142.0000000000000000 ) ) ;
#13418=FACE_OUTER_BOUND ( 'NONE', #195223, .T. ) ;
#13501=CARTESIAN_POINT ( 'NONE',  ( -24.27995301597599465, -6.552671593955007978, 171.1165850637241874 ) ) ;
#13502=ORIENTED_EDGE ( 'NONE', *, *, #84475, .T. ) ;
#13689=DIRECTION ( 'NONE',  ( -0.1039620511844979306, 0.1039620511844979306, 0.9891328443778538704 ) ) ;
#13744=CARTESIAN_POINT ( 'NONE',  ( 17.14385361876520264, 23.59649016807275856, 142.6750000027311103 ) ) ;
#13748=CARTESIAN_POINT ( 'NONE',  ( 27.73933785331498214, 9.013057229001095294, 146.4750000027311501 ) ) ;
#13777=ADVANCED_FACE ( 'NONE', ( #136598 ), #73959, .T. ) ;
#13784=CARTESIAN_POINT ( 'NONE',  ( -25.82893184621037364, -8.167111171438232731, 172.3011985515803701 ) ) ;
#13909=CARTESIAN_POINT ( 'NONE',  ( -30.82560697742735911, 2.051108057200722688E-14, 150.0000000000000000 ) ) ;
#13959=DIRECTION ( 'NONE',  ( -0.9945218953682734009, 0.000000000000000000, -0.1045284632676528741 ) ) ;
#14005=CARTESIAN_POINT ( 'NONE',  ( 24.20534277172198756, -9.236732224056902751, 166.4300944521385190 ) ) ;
#14020=CARTESIAN_POINT ( 'NONE',  ( 26.03370437638686852, 6.875205692009825675, 160.5968874236875195 ) ) ;
#14086=CARTESIAN_POINT ( 'NONE',  ( -5.359611314223446995E-15, 29.16686587814335496, 148.3750000027311842 ) ) ;
#14143=CARTESIAN_POINT ( 'NONE',  ( 28.79475375365685963, 9.355982642737862065, 141.3656553485623704 ) ) ;
#14246=CARTESIAN_POINT ( 'NONE',  ( -22.44159573604009950, -16.30477369853688430, 147.0750000027312012 ) ) ;
#14309=EDGE_CURVE ( 'NONE', #114568, #105306, #48259, .T. ) ;
#14375=CARTESIAN_POINT ( 'NONE',  ( 25.85231681326528985, 7.957828899753591756, 172.6576833274792762 ) ) ;
#14391=AXIS2_PLACEMENT_3D ( 'NONE', #152755, #167938, #196321 ) ;
#14412=LINE ( 'NONE', #123561, #1657 ) ;
#14434=ORIENTED_EDGE ( 'NONE', *, *, #137956, .F. ) ;
#14491=ORIENTED_EDGE ( 'NONE', *, *, #192849, .T. ) ;
#14510=AXIS2_PLACEMENT_3D ( 'NONE', #119522, #166026, #27526 ) ;
#14530=CARTESIAN_POINT ( 'NONE',  ( -26.11842041226232780, -7.699311778675193452, 169.4341694154020956 ) ) ;
#14659=CARTESIAN_POINT ( 'NONE',  ( 26.85241745982147421, -7.190459374138095328, 139.9999999999999716 ) ) ;
#14743=CARTESIAN_POINT ( 'NONE',  ( 22.44159573604009239, 16.30477369853692693, 144.5750000027311728 ) ) ;
#14747=CARTESIAN_POINT ( 'NONE',  ( -8.571926809382608425, 26.38167802310805854, 148.9750000027311785 ) ) ;
#14784=CARTESIAN_POINT ( 'NONE',  ( -21.35462415990328822, -10.43496131973800090, 170.3924512066482748 ) ) ;
#14909=VECTOR ( 'NONE', #140815, 1000.000000000000000 ) ;
#14936=CARTESIAN_POINT ( 'NONE',  ( -15.67939035206521936, 24.07275550605739767, 140.0000000000000000 ) ) ;
#14951=CARTESIAN_POINT ( 'NONE',  ( 8.898068258721473001, -27.38543819252872069, 144.8656553485623704 ) ) ;
#14963=CARTESIAN_POINT ( 'NONE',  ( -21.98685479826777112, -13.98560643873833875, 165.5209445330007441 ) ) ;
#14984=CARTESIAN_POINT ( 'NONE',  ( -21.92716348790883529, -9.076607822308508489, 171.2490935175190998 ) ) ;
#15010=AXIS2_PLACEMENT_3D ( 'NONE', #82346, #158217, #160210 ) ;
#15047=ORIENTED_EDGE ( 'NONE', *, *, #92009, .T. ) ;
#15061=FACE_OUTER_BOUND ( 'NONE', #145996, .T. ) ;
#15087=CARTESIAN_POINT ( 'NONE',  ( 17.14385361876520264, -23.59649016807271238, 147.5750000027311444 ) ) ;
#15125=CARTESIAN_POINT ( 'NONE',  ( -3.573655867282028392E-15, 2.428612866367529932E-14, 139.9999999999999716 ) ) ;
#15164=CIRCLE ( 'NONE', #31328, 26.79475375365586487 ) ;
#15177=LINE ( 'NONE', #154678, #56405 ) ;
#15178=CARTESIAN_POINT ( 'NONE',  ( -26.00062938246246702, -10.06977165081872094, 166.7331697587468682 ) ) ;
#15223=CARTESIAN_POINT ( 'NONE',  ( 27.18966431762777702, -4.276553394869359259, 168.7322077152510928 ) ) ;
#15251=CARTESIAN_POINT ( 'NONE',  ( 8.571926809382597767, 26.38167802310806209, 146.2750000027311899 ) ) ;
#15286=DIRECTION ( 'NONE',  ( -1.000000000000000000, 0.000000000000000000, 0.000000000000000000 ) ) ;
#15332=CARTESIAN_POINT ( 'NONE',  ( -25.85231681326420272, 7.957828899755264196, 172.6576833274792762 ) ) ;
#15336=VECTOR ( 'NONE', #128029, 1000.000000000000000 ) ;
#15391=CARTESIAN_POINT ( 'NONE',  ( 17.81289503416610742, 24.51734667627700404, 143.2999999999999829 ) ) ;
#15429=AXIS2_PLACEMENT_3D ( 'NONE', #41357, #6995, #160693 ) ;
#15498=VERTEX_POINT ( 'NONE', #157145 ) ;
#15525=CARTESIAN_POINT ( 'NONE',  ( -28.79475375365586842, 2.428612866367529932E-14, 146.2656553485623760 ) ) ;
#15531=LINE ( 'NONE', #338, #92020 ) ;
#15655=CARTESIAN_POINT ( 'NONE',  ( 26.32373036410889355, -8.933993968303854061, 140.0000000000000000 ) ) ;
#15679=CARTESIAN_POINT ( 'NONE',  ( 20.84945647820395109, -10.59429869652066891, 168.2340845703681964 ) ) ;
#15702=EDGE_CURVE ( 'NONE', #140232, #144449, #79767, .T. ) ;
#15724=DIRECTION ( 'NONE',  ( 0.000000000000000000, 0.000000000000000000, -1.000000000000000000 ) ) ;
#15737=CARTESIAN_POINT ( 'NONE',  ( 27.73933785331498925, -9.013057229001033122, 146.2750000027311899 ) ) ;
#15741=CARTESIAN_POINT ( 'NONE',  ( 8.571926809382597767, 26.38167802310806209, 148.7750000027311899 ) ) ;
#15776=CARTESIAN_POINT ( 'NONE',  ( -25.34721418589374764, -10.09305078451760274, 170.5222919391028142 ) ) ;
#15828=ADVANCED_BREP_SHAPE_REPRESENTATION ( '', ( #73950, #82054 ), #166266 ) ;
#15832=AXIS2_PLACEMENT_3D ( 'NONE', #62650, #168836, #123322 ) ;
#15959=CARTESIAN_POINT ( 'NONE',  ( -23.42531391676912378, -11.30614932247368287, 165.8025715494068777 ) ) ;
#16022=CARTESIAN_POINT ( 'NONE',  ( -23.03120525563286947, 11.22467059994864336, 168.0473679553712429 ) ) ;
#16059=CARTESIAN_POINT ( 'NONE',  ( -3.573655867282028392E-15, 2.428612866367529932E-14, 155.0000000000000000 ) ) ;
#16085=CARTESIAN_POINT ( 'NONE',  ( -22.44159573604009950, -16.30477369853688430, 145.0750000027311728 ) ) ;
#16090=ORIENTED_EDGE ( 'NONE', *, *, #19851, .F. ) ;
#16161=CARTESIAN_POINT ( 'NONE',  ( 17.79613651744293534, 24.49428055684532524, 143.2843446568999468 ) ) ;
#16196=PLANE ( 'NONE',  #3280 ) ;
#16214=CARTESIAN_POINT ( 'NONE',  ( 28.79475375365586132, 2.781246896534039337E-14, 148.9843446568999923 ) ) ;
#16216=EDGE_CURVE ( 'NONE', #83996, #61621, #196998, .T. ) ;
#16229=VERTEX_POINT ( 'NONE', #146959 ) ;
#16250=CARTESIAN_POINT ( 'NONE',  ( 8.571926809382597767, 26.38167802310806209, 142.2750000027311899 ) ) ;
#16258=CARTESIAN_POINT ( 'NONE',  ( 23.34492853952200520, -11.48509598731610737, 165.7658222004385777 ) ) ;
#16284=CARTESIAN_POINT ( 'NONE',  ( 28.79475375365586132, 2.781246896534039337E-14, 140.9843446568999923 ) ) ;
#16388=CARTESIAN_POINT ( 'NONE',  ( 23.31738231874054534, 16.94106989632529192, 145.1999999999999886 ) ) ;
#16394=EDGE_CURVE ( 'NONE', #63582, #33758, #63021, .T. ) ;
#16401=CARTESIAN_POINT ( 'NONE',  ( 26.36463166569300043, -3.076743934664109226, 174.2851114983688490 ) ) ;
#16405=CARTESIAN_POINT ( 'NONE',  ( 28.79475375365679923, 9.355982642737952659, 143.3656553485623704 ) ) ;
#16482=CARTESIAN_POINT ( 'NONE',  ( -24.68411608548712266, -7.148172978119915477, 167.5704058020797902 ) ) ;
#16483=ORIENTED_EDGE ( 'NONE', *, *, #193676, .F. ) ;
#16521=CARTESIAN_POINT ( 'NONE',  ( -26.24776304279841455, -7.664901067105981625, 169.1545021717929842 ) ) ;
#16542=CARTESIAN_POINT ( 'NONE',  ( -29.15849868437705439, 10.00000000000000000, 150.0000000000000000 ) ) ;
#16670=CARTESIAN_POINT ( 'NONE',  ( 21.27520710526538394, -9.818903669220862440, 168.4804316999487526 ) ) ;
#16698=ORIENTED_EDGE ( 'NONE', *, *, #175528, .F. ) ;
#16733=CARTESIAN_POINT ( 'NONE',  ( -27.73933785331498925, -9.013057229001049109, 145.4750000027311501 ) ) ;
#16757=CARTESIAN_POINT ( 'NONE',  ( 25.31894786019267229, -4.571304203950320222, 167.3973414147893379 ) ) ;
#16922=CARTESIAN_POINT ( 'NONE',  ( -0.1587466045633683653, 28.39722349821926528, 140.0000000000000000 ) ) ;
#16957=ORIENTED_EDGE ( 'NONE', *, *, #116692, .T. ) ;
#16973=CARTESIAN_POINT ( 'NONE',  ( -21.38418241377624085, 7.427326039334300134, 174.4773576836617224 ) ) ;
#17014=CARTESIAN_POINT ( 'NONE',  ( -21.75836449082843060, 8.509082329563685931, 169.1767350484841472 ) ) ;
#17073=CARTESIAN_POINT ( 'NONE',  ( 21.76481224609945997, 7.725237430229302760, 173.1951747752679296 ) ) ;
#17078=CARTESIAN_POINT ( 'NONE',  ( -17.14385361876520264, -23.59649016807271593, 141.1750000027311671 ) ) ;
#17092=CARTESIAN_POINT ( 'NONE',  ( -24.81835718235489097, -6.052279806424480491, 168.4265042179603427 ) ) ;
#17150=ORIENTED_EDGE ( 'NONE', *, *, #173096, .T. ) ;
#17241=CARTESIAN_POINT ( 'NONE',  ( -17.14385361876520264, -23.59649016807271593, 139.1750000027311955 ) ) ;
#17391=CARTESIAN_POINT ( 'NONE',  ( 21.88033147701266046, -9.239123595177041182, 171.1226046679831825 ) ) ;
#17404=CARTESIAN_POINT ( 'NONE',  ( 24.77450267193474787, 6.022707119490100069, 168.7078695393446424 ) ) ;
#17489=CARTESIAN_POINT ( 'NONE',  ( -22.44159573604010305, 16.30477369853692338, 147.1750000027311671 ) ) ;
#17511=CARTESIAN_POINT ( 'NONE',  ( -26.53315420742543651, -7.611574518544844459, 168.2743882774363726 ) ) ;
#17555=CARTESIAN_POINT ( 'NONE',  ( -29.15849868437705439, 7.427326039334300134, 174.4773576836617224 ) ) ;
#17581=AXIS2_PLACEMENT_3D ( 'NONE', #169847, #44528, #28389 ) ;
#17592=EDGE_CURVE ( 'NONE', #10845, #135262, #45752, .T. ) ;
#17600=EDGE_LOOP ( 'NONE', ( #161936, #80105, #14491, #79742 ) ) ;
#17642=CARTESIAN_POINT ( 'NONE',  ( 12.31437665787661295, -24.87262748924413813, 139.9999999999999716 ) ) ;
#17691=CIRCLE ( 'NONE', #88710, 4.999999999999998224 ) ;
#17787=CARTESIAN_POINT ( 'NONE',  ( 28.79475375365487366, -9.355982642740542587, 141.1656553485623817 ) ) ;
#17917=LINE ( 'NONE', #79572, #120634 ) ;
#17964=CARTESIAN_POINT ( 'NONE',  ( 26.58496454516999563, 7.626754437231445749, 167.9682100371138915 ) ) ;
#17976=CARTESIAN_POINT ( 'NONE',  ( -21.83922654085339587, 7.858455564366264134, 172.8813051029758299 ) ) ;
#17982=EDGE_CURVE ( 'NONE', #18152, #173841, #96073, .T. ) ;
#18017=CARTESIAN_POINT ( 'NONE',  ( -23.46037622756033869, 10.21219847193944474, 168.3031241911537279 ) ) ;
#18037=ORIENTED_EDGE ( 'NONE', *, *, #137185, .T. ) ;
#18060=DIRECTION ( 'NONE',  ( -1.000000000000000000, 0.000000000000000000, -0.000000000000000000 ) ) ;
#18082=CARTESIAN_POINT ( 'NONE',  ( -8.571926809382608425, 26.38167802310805854, 142.4750000027312069 ) ) ;
#18152=VERTEX_POINT ( 'NONE', #99201 ) ;
#18165=CARTESIAN_POINT ( 'NONE',  ( -24.95432927374998044, -3.806786798636382585, 190.0000000000000000 ) ) ;
#18190=ORIENTED_EDGE ( 'NONE', *, *, #93397, .F. ) ;
#18222=FACE_OUTER_BOUND ( 'NONE', #106812, .T. ) ;
#18246=CARTESIAN_POINT ( 'NONE',  ( -17.14385361876520619, 23.59649016807275856, 140.5750000027311728 ) ) ;
#18310=CARTESIAN_POINT ( 'NONE',  ( 20.93662873023604121, 10.44628751056226612, 168.2749732860604865 ) ) ;
#18374=CARTESIAN_POINT ( 'NONE',  ( -25.82634036940375921, 7.758313425001081676, 169.9660385289634519 ) ) ;
#18396=CARTESIAN_POINT ( 'NONE',  ( 25.93326183087870973, -10.28624940747355510, 166.6531433017868835 ) ) ;
#18403=SURFACE_STYLE_FILL_AREA ( #31572 ) ;
#18425=VERTEX_POINT ( 'NONE', #132554 ) ;
#18475=CARTESIAN_POINT ( 'NONE',  ( 8.906447517083050158, 27.41122689804195645, 145.6500000054623740 ) ) ;
#18490=CARTESIAN_POINT ( 'NONE',  ( -22.44159573604009950, -16.30477369853688430, 147.5750000027312012 ) ) ;
#18510=AXIS2_PLACEMENT_3D ( 'NONE', #16542, #33689, #46880 ) ;
#18727=CARTESIAN_POINT ( 'NONE',  ( -24.69864643647405344, 7.736333414721471513, 171.5373488951853460 ) ) ;
#18762=FACE_OUTER_BOUND ( 'NONE', #179582, .T. ) ;
#18918=CARTESIAN_POINT ( 'NONE',  ( 27.94727380668107131, 6.976214527048578695, 161.4607934399207920 ) ) ;
#18956=CARTESIAN_POINT ( 'NONE',  ( 25.12471020271277666, 7.795852113654127002, 170.9710663016988974 ) ) ;
#19008=CARTESIAN_POINT ( 'NONE',  ( -24.83221077041876512, 4.296110748028908688, 170.3917201292316577 ) ) ;
#19072=CARTESIAN_POINT ( 'NONE',  ( -27.73933785331498925, -9.013057229001049109, 138.9750000027311785 ) ) ;
#19155=CARTESIAN_POINT ( 'NONE',  ( -24.81835718235489097, -6.052279806424480491, 168.4265042179603427 ) ) ;
#19178=ORIENTED_EDGE ( 'NONE', *, *, #66645, .T. ) ;
#19180=DIRECTION ( 'NONE',  ( 0.000000000000000000, 0.000000000000000000, 1.000000000000000000 ) ) ;
#19201=CARTESIAN_POINT ( 'NONE',  ( 8.898068258721464119, 27.38543819252877398, 149.3843446568999980 ) ) ;
#19236=CARTESIAN_POINT ( 'NONE',  ( 1.784210473542230573E-15, -29.16686587814331588, 139.3750000027311842 ) ) ;
#19284=AXIS2_PLACEMENT_3D ( 'NONE', #173440, #34909, #51076 ) ;
#19300=CARTESIAN_POINT ( 'NONE',  ( 24.68411608548795044, 7.148172978119885279, 167.5704058020753848 ) ) ;
#19336=EDGE_CURVE ( 'NONE', #18425, #70413, #187788, .T. ) ;
#19382=CARTESIAN_POINT ( 'NONE',  ( 25.82893184620924742, -8.167111171437140271, 172.3011985515803417 ) ) ;
#19410=EDGE_LOOP ( 'NONE', ( #154661, #151131, #54818, #72338, #46622 ) ) ;
#19462=CARTESIAN_POINT ( 'NONE',  ( -17.81289503416611097, -24.51734667627696496, 144.5500000054623513 ) ) ;
#19482=EDGE_CURVE ( 'NONE', #66692, #186058, #128298, .T. ) ;
#19732=CARTESIAN_POINT ( 'NONE',  ( 26.03370437638690049, -6.875205692009868308, 160.5968874236871784 ) ) ;
#19743=CARTESIAN_POINT ( 'NONE',  ( -21.36928693577339189, -7.422813773936192128, 174.5222352431090087 ) ) ;
#19762=CARTESIAN_POINT ( 'NONE',  ( -24.95432927374998044, 0.000000000000000000, 190.0000000000000000 ) ) ;
#19851=EDGE_CURVE ( 'NONE', #45770, #75663, #191977, .T. ) ;
#19922=CARTESIAN_POINT ( 'NONE',  ( -23.84690145917539894, 10.26550538186637596, 166.0764395470883983 ) ) ;
#20062=CARTESIAN_POINT ( 'NONE',  ( 27.46925885783806720, -7.746560145625162264, 162.9586723222894875 ) ) ;
#20353=ORIENTED_EDGE ( 'NONE', *, *, #14309, .F. ) ;
#20358=CARTESIAN_POINT ( 'NONE',  ( 21.51693143705161404, -10.15780255052775161, 170.5200780514259691 ) ) ;
#20362=LINE ( 'NONE', #34549, #44992 ) ;
#20369=CARTESIAN_POINT ( 'NONE',  ( 22.03588254365928378, -7.477584490968436803, 173.9991804579097163 ) ) ;
#20379=CARTESIAN_POINT ( 'NONE',  ( -21.38418241377623374, -5.438282248597753110, 174.2683007571264113 ) ) ;
#20383=CARTESIAN_POINT ( 'NONE',  ( -27.73933785331498925, 9.013057229001088189, 142.7750000027311899 ) ) ;
#20437=CARTESIAN_POINT ( 'NONE',  ( 17.14385361876520264, 23.59649016807275856, 142.6750000027311103 ) ) ;
#20438=CARTESIAN_POINT ( 'NONE',  ( -5.429308488886486681E-15, 30.30510711980690175, 143.7500000054623399 ) ) ;
#20665=CARTESIAN_POINT ( 'NONE',  ( -26.00011078373267637, 10.07146799416499938, 166.7325096689061183 ) ) ;
#20848=CARTESIAN_POINT ( 'NONE',  ( 26.26083487095746349, -9.141127703660906434, 167.1337248662267712 ) ) ;
#20888=CARTESIAN_POINT ( 'NONE',  ( 27.07824611089273148, 7.738748529345179428, 165.1039267699882771 ) ) ;
#20942=ORIENTED_EDGE ( 'NONE', *, *, #92116, .F. ) ;
#20971=CARTESIAN_POINT ( 'NONE',  ( 21.98685479826776046, -13.98560643873834763, 165.5209445330007725 ) ) ;
#20997=ORIENTED_EDGE ( 'NONE', *, *, #134205, .T. ) ;
#21058=EDGE_CURVE ( 'NONE', #31781, #51307, #153732, .T. ) ;
#21144=DIRECTION ( 'NONE',  ( 0.000000000000000000, 0.000000000000000000, -1.000000000000000000 ) ) ;
#21167=CARTESIAN_POINT ( 'NONE',  ( 27.32543223595550330, 4.845308524271299433, 167.4404622590899407 ) ) ;
#21182=( NAMED_UNIT ( * ) SI_UNIT ( $, .STERADIAN. ) SOLID_ANGLE_UNIT ( ) );
#21279=CARTESIAN_POINT ( 'NONE',  ( 24.10180676228321062, 9.559744493757255768, 166.3058469464613154 ) ) ;
#21366=CARTESIAN_POINT ( 'NONE',  ( -25.51209292918185056, 5.276535733812623974, 165.5596888358906540 ) ) ;
#21389=CARTESIAN_POINT ( 'NONE',  ( 22.44159573604009594, -16.30477369853687364, 143.6750000027311671 ) ) ;
#21437=ORIENTED_EDGE ( 'NONE', *, *, #117196, .F. ) ;
#21443=CARTESIAN_POINT ( 'NONE',  ( 27.73933785331498214, 9.013057229001095294, 140.4750000027311785 ) ) ;
#21444=CARTESIAN_POINT ( 'NONE',  ( -23.31738231874055600, 16.94106989632528837, 146.0500000054623797 ) ) ;
#21457=CARTESIAN_POINT ( 'NONE',  ( 8.571926809382597767, 26.38167802310806209, 142.7750000027311899 ) ) ;
#21477=VECTOR ( 'NONE', #81918, 1000.000000000000000 ) ;
#21497=CARTESIAN_POINT ( 'NONE',  ( 21.98685479826775335, -13.98560643873835652, 165.5209445330007441 ) ) ;
#21532=CARTESIAN_POINT ( 'NONE',  ( 1.988064558232696151E-15, -30.27659582821216588, 142.7656553485623760 ) ) ;
#21634=ADVANCED_FACE ( 'NONE', ( #18222 ), #2037, .T. ) ;
#21732=FACE_OUTER_BOUND ( 'NONE', #93524, .T. ) ;
#21942=CARTESIAN_POINT ( 'NONE',  ( -23.75112013235312602, -10.51683317207933044, 166.0021274478077942 ) ) ;
#21980=CARTESIAN_POINT ( 'NONE',  ( 24.57691432906898044, -7.727872488963283715, 167.2019946024468595 ) ) ;
#22183=PRESENTATION_STYLE_ASSIGNMENT (( #192028 ) ) ;
#22207=ADVANCED_FACE ( 'NONE', ( #120163 ), #33228, .F. ) ;
#22282=CARTESIAN_POINT ( 'NONE',  ( 19.49401214000076976, 12.39993551617566681, 167.9999999999999716 ) ) ;
#22451=CARTESIAN_POINT ( 'NONE',  ( 8.906447517083057264, -27.41122689804191026, 138.8500000054623911 ) ) ;
#22454=ORIENTED_EDGE ( 'NONE', *, *, #193877, .F. ) ;
#22465=CARTESIAN_POINT ( 'NONE',  ( -17.14385361876520975, 23.59649016807275856, 141.0750000027311728 ) ) ;
#22578=CARTESIAN_POINT ( 'NONE',  ( 26.57611637973579732, 7.696099174151423306, 167.9177021574031983 ) ) ;
#22857=CARTESIAN_POINT ( 'NONE',  ( 26.47577687012304182, -8.223210953690971436, 167.6032987643051513 ) ) ;
#22894=CARTESIAN_POINT ( 'NONE',  ( 27.91695578976620951, 6.846979738060676723, 161.8037495850574032 ) ) ;
#22942=CARTESIAN_POINT ( 'NONE',  ( -23.14613071126279209, -10.96668486446954560, 168.1016194467971445 ) ) ;
#22979=CARTESIAN_POINT ( 'NONE',  ( 21.93180397000137205, -7.641141194974085948, 169.8616410530775909 ) ) ;
#23173=CARTESIAN_POINT ( 'NONE',  ( 27.74069374691240242, 6.311165852663350506, 163.4895129000348390 ) ) ;
#23285=CARTESIAN_POINT ( 'NONE',  ( 24.79447686064953871, 6.332871904612077607, 168.1804317516251501 ) ) ;
#23342=ORIENTED_EDGE ( 'NONE', *, *, #21058, .T. ) ;
#23451=CARTESIAN_POINT ( 'NONE',  ( 17.14385361876520264, -23.59649016807271238, 142.0750000027311444 ) ) ;
#23452=CARTESIAN_POINT ( 'NONE',  ( -23.31738231874055245, -16.94106989632524574, 138.4500000054623570 ) ) ;
#23465=CARTESIAN_POINT ( 'NONE',  ( -27.73933785331498925, -9.013057229001049109, 143.4750000027312069 ) ) ;
#23523=CARTESIAN_POINT ( 'NONE',  ( -25.51181203389340268, -5.285008086477787081, 165.5623613760384387 ) ) ;
#23580=CARTESIAN_POINT ( 'NONE',  ( 24.54404792736140095, 12.06373989673628877, 169.8487138613017180 ) ) ;
#23593=CARTESIAN_POINT ( 'NONE',  ( 8.571926809382603096, -26.38167802310801235, 139.9750000027311785 ) ) ;
#23762=CARTESIAN_POINT ( 'NONE',  ( 24.37439536253439343, 13.84063584238319322, 165.9041067986157998 ) ) ;
#23945=CARTESIAN_POINT ( 'NONE',  ( -23.63516320021014749, -9.722623904421999086, 168.4908852323012241 ) ) ;
#23960=ORIENTED_EDGE ( 'NONE', *, *, #159956, .T. ) ;
#23982=CARTESIAN_POINT ( 'NONE',  ( 21.56952297831669441, -5.557039098534934496, 173.4609804364286276 ) ) ;
#24085=LINE ( 'NONE', #114066, #138666 ) ;
#24178=EDGE_CURVE ( 'NONE', #105726, #189536, #182557, .T. ) ;
#24215=ORIENTED_EDGE ( 'NONE', *, *, #28979, .F. ) ;
#24221=CARTESIAN_POINT ( 'NONE',  ( 27.05641397906351386, 2.428612866367529932E-14, 169.9999999999999716 ) ) ;
#24281=CARTESIAN_POINT ( 'NONE',  ( -27.86188877290821964, -7.554847477551930091, 161.1024127393599201 ) ) ;
#24408=CARTESIAN_POINT ( 'NONE',  ( -17.14385361876520975, 23.59649016807275856, 142.5750000027311728 ) ) ;
#24463=CARTESIAN_POINT ( 'NONE',  ( -5.359611314223446995E-15, 29.16686587814335496, 140.8750000027311842 ) ) ;
#24464=CARTESIAN_POINT ( 'NONE',  ( -28.82186960331499037, 2.428612866367529932E-14, 138.2500000054623683 ) ) ;
#24477=CARTESIAN_POINT ( 'NONE',  ( -17.14385361876520264, -23.59649016807271238, 143.6750000027311671 ) ) ;
#24534=CARTESIAN_POINT ( 'NONE',  ( -26.03370437638690049, -6.875205692009850544, 160.5968874236872637 ) ) ;
#24549=CARTESIAN_POINT ( 'NONE',  ( -24.95262708931866769, 12.69764001896744432, 166.0532406165024497 ) ) ;
#24582=B_SPLINE_CURVE_WITH_KNOTS ( 'NONE', 3,
 ( #73885, #74864, #89032, #136526, #152682, #87040, #102213, #163902, #148725, #150723, #12222, #133542, #195233, #198207, #135555, #180082, #59678, #121350, #164896, #56716, #183043, #41551, #118388, #197227, #26390, #58689, #44526, #106182 ),
 .UNSPECIFIED., .F., .F.,
 ( 4, 2, 2, 2, 2, 2, 2, 2, 2, 2, 2, 2, 2, 4 ),
 ( 1.734723475976807094E-18, 0.0005512667261461052853, 0.001102533452292208836, 0.001240350133828699080, 0.001378166815365189542, 0.001447075156133453963, 0.001515983496901718384, 0.001653800178438247226, 0.001929433541511376684, 0.002205066904584506143, 0.003307600356876775477, 0.004410133809169045245, 0.006615200713753665446, 0.008820267618338286514 ),
 .UNSPECIFIED. ) ;
#24591=CARTESIAN_POINT ( 'NONE',  ( 25.52568752982265110, 9.519068727185217682, 170.8917780290381927 ) ) ;
#24603=CARTESIAN_POINT ( 'NONE',  ( -28.82186960331499392, 9.364793116373565596, 145.8999999999999773 ) ) ;
#24620=ORIENTED_EDGE ( 'NONE', *, *, #59575, .F. ) ;
#24657=CARTESIAN_POINT ( 'NONE',  ( 24.95432927374998400, -4.974562764236790002, 189.9999999999999716 ) ) ;
#24747=EDGE_CURVE ( 'NONE', #105726, #186058, #62031, .T. ) ;
#24749=CARTESIAN_POINT ( 'NONE',  ( -3.573655867282028392E-15, 2.428612866367529932E-14, 169.9999999999999716 ) ) ;
#24762=CARTESIAN_POINT ( 'NONE',  ( 8.571926809382603096, -26.38167802310801235, 147.4750000027311785 ) ) ;
#24864=EDGE_CURVE ( 'NONE', #86852, #56947, #90523, .T. ) ;
#24876=CARTESIAN_POINT ( 'NONE',  ( -19.49401214000077331, 12.39993551617566681, 167.9999999999999716 ) ) ;
#24918=EDGE_CURVE ( 'NONE', #135939, #11685, #137026, .T. ) ;
#24984=CIRCLE ( 'NONE', #2429, 27.29906736325805028 ) ;
#24996=CARTESIAN_POINT ( 'NONE',  ( 24.14511064691487263, -7.743397529684092007, 169.7652520481140073 ) ) ;
#25153=CARTESIAN_POINT ( 'NONE',  ( 26.12113310390727250, -7.698689789033765329, 169.4288210027979460 ) ) ;
#25231=LINE ( 'NONE', #24221, #11077 ) ;
#25238=PLANE ( 'NONE',  #78925 ) ;
#25285=CARTESIAN_POINT ( 'NONE',  ( 28.79475375365512946, -9.355982642740189092, 142.8843446568999980 ) ) ;
#25364=VERTEX_POINT ( 'NONE', #159959 ) ;
#25475=CARTESIAN_POINT ( 'NONE',  ( 17.14385361876520264, 23.59649016807275856, 148.1750000027311955 ) ) ;
#25487=CARTESIAN_POINT ( 'NONE',  ( 27.73933785331498569, 9.013057229001093518, 144.4750000027311785 ) ) ;
#25517=CARTESIAN_POINT ( 'NONE',  ( -3.573655867282028392E-15, 2.428612866367529932E-14, 167.9999999999999716 ) ) ;
#25559=CARTESIAN_POINT ( 'NONE',  ( -21.88033147701377601, 9.239123595177357373, 171.1226046679828983 ) ) ;
#25610=CARTESIAN_POINT ( 'NONE',  ( 27.73933785331498569, 2.768321779492822058E-14, 140.3750000027311842 ) ) ;
#25657=ORIENTED_EDGE ( 'NONE', *, *, #24864, .F. ) ;
#25665=CARTESIAN_POINT ( 'NONE',  ( 22.96528548301342809, -5.795830589372932273, 190.0000000000000000 ) ) ;
#25747=CARTESIAN_POINT ( 'NONE',  ( -21.47377332591982224, 5.474134792251751591, 173.8918256800988900 ) ) ;
#25765=CARTESIAN_POINT ( 'NONE',  ( 8.571926809382597767, 26.38167802310806209, 148.2750000027311899 ) ) ;
#25953=CARTESIAN_POINT ( 'NONE',  ( 17.14385361876520264, 23.59649016807275856, 146.6750000027311671 ) ) ;
#25993=CARTESIAN_POINT ( 'NONE',  ( 24.17640770809924078, -7.553848413212526758, 169.9412368235734618 ) ) ;
#26127=CARTESIAN_POINT ( 'NONE',  ( -28.09353542562696404, -5.934688857626441383, 140.0000000000000000 ) ) ;
#26137=ADVANCED_FACE ( 'NONE', ( #12297 ), #104287, .T. ) ;
#26146=CARTESIAN_POINT ( 'NONE',  ( 24.93942350307310107, -7.769968609432603479, 171.2173313942149377 ) ) ;
#26158=B_SPLINE_CURVE_WITH_KNOTS ( 'NONE', 3,
 ( #100845, #83678, #145356, #131190, #129179, #37184, #161535, #192880, #68517, #70527, #96855, #130171, #191868, #112045 ),
 .UNSPECIFIED., .F., .F.,
 ( 4, 2, 2, 2, 2, 2, 4 ),
 ( 3.469446951953614189E-18, 0.002289927113134818983, 0.003434890669702226739, 0.004579854226269634496, 0.006869781339404426590, 0.008014744895971800953, 0.009159708452539173582 ),
 .UNSPECIFIED. ) ;
#26181=ORIENTED_EDGE ( 'NONE', *, *, #24918, .T. ) ;
#26195=CARTESIAN_POINT ( 'NONE',  ( -21.96405779611666631, 8.831116573701658368, 171.4809137887048962 ) ) ;
#26276=DIRECTION ( 'NONE',  ( -0.000000000000000000, -1.000000000000000000, -0.000000000000000000 ) ) ;
#26301=FACE_OUTER_BOUND ( 'NONE', #135865, .T. ) ;
#26390=CARTESIAN_POINT ( 'NONE',  ( -27.07812102864229686, 7.738729533396094595, 165.1046384229469766 ) ) ;
#26465=CARTESIAN_POINT ( 'NONE',  ( 8.906447517083050158, 27.41122689804195645, 141.6500000054623740 ) ) ;
#26506=DIRECTION ( 'NONE',  ( 0.8437662581494456138, -0.5367108174878562066, 0.000000000000000000 ) ) ;
#26545=CARTESIAN_POINT ( 'NONE',  ( -25.76143648877210524, 7.343476467573863076, 174.8772314887147843 ) ) ;
#26600=CARTESIAN_POINT ( 'NONE',  ( 1.784210473542230573E-15, -29.16686587814331588, 139.8750000027311842 ) ) ;
#26625=CARTESIAN_POINT ( 'NONE',  ( -22.54345066063601166, 5.578190839439332471, 172.9373910537578638 ) ) ;
#26667=LINE ( 'NONE', #86320, #52948 ) ;
#26675=EDGE_LOOP ( 'NONE', ( #852, #62453, #94412, #14434 ) ) ;
#26688=DIRECTION ( 'NONE',  ( 1.000000000000000000, 0.000000000000000000, 0.000000000000000000 ) ) ;
#26744=FACE_OUTER_BOUND ( 'NONE', #180367, .T. ) ;
#26757=CARTESIAN_POINT ( 'NONE',  ( -5.359611314223446995E-15, 29.16686587814335851, 146.3750000027311842 ) ) ;
#26768=CARTESIAN_POINT ( 'NONE',  ( 26.58496454516999563, 7.626754437231445749, 167.9682100371138915 ) ) ;
#26991=CARTESIAN_POINT ( 'NONE',  ( -23.64729612845568596, -13.72274676820315342, 169.8070494178799663 ) ) ;
#27113=CARTESIAN_POINT ( 'NONE',  ( -3.573655867282028392E-15, 2.428612866367529932E-14, 139.9999999999999716 ) ) ;
#27128=CARTESIAN_POINT ( 'NONE',  ( -21.58577566615619503, 5.573877917343206256, 173.3856758005497340 ) ) ;
#27165=AXIS2_PLACEMENT_3D ( 'NONE', #192508, #117662, #179359 ) ;
#27191=CARTESIAN_POINT ( 'NONE',  ( -21.96329795405619123, -8.386426352705242948, 172.0132153625897899 ) ) ;
#27282=( BOUNDED_CURVE ( )  B_SPLINE_CURVE ( 2, ( #146964, #132792, #190477, #70125, #179325, #6431, #40789, #8452, #51950, #113610, #175304 ),
 .UNSPECIFIED., .F., .F. ) 
 B_SPLINE_CURVE_WITH_KNOTS ( ( 3, 2, 2, 2, 2, 3 ),
 ( 0.2000000000000029532, 0.2200000000000029710, 0.2400000000000029887, 0.2600000000000030065, 0.2800000000000030798, 0.3000000000000030420 ),
 .UNSPECIFIED. ) 
 CURVE ( )  GEOMETRIC_REPRESENTATION_ITEM ( )  RATIONAL_B_SPLINE_CURVE ( ( 0.9999999999999927836, 0.9510565162951607476, 1.000000000000000000, 0.9510565162951535312, 1.000000000000000000, 0.9510565162951535312, 1.000000000000000000, 0.9510565162951535312, 1.000000000000000000, 0.9510565162951460927, 1.000000000000007550 ) ) 
 REPRESENTATION_ITEM ( '' )  );
#27356=ORIENTED_EDGE ( 'NONE', *, *, #79706, .F. ) ;
#27359=CARTESIAN_POINT ( 'NONE',  ( 17.79613651744293534, 24.49428055684532524, 141.5656553485623590 ) ) ;
#27421=CIRCLE ( 'NONE', #4840, 27.29906736325805028 ) ;
#27425=DIRECTION ( 'NONE',  ( 0.000000000000000000, 0.000000000000000000, -1.000000000000000000 ) ) ;
#27445=ORIENTED_EDGE ( 'NONE', *, *, #61925, .F. ) ;
#27466=CARTESIAN_POINT ( 'NONE',  ( 28.79475375365586132, 2.781246896534039337E-14, 155.0000000000000000 ) ) ;
#27467=CARTESIAN_POINT ( 'NONE',  ( -22.44159573604010305, 16.30477369853692338, 146.6750000027311671 ) ) ;
#27503=EDGE_LOOP ( 'NONE', ( #118449, #100255, #111070, #174329, #1293, #112415, #32832, #37106 ) ) ;
#27526=DIRECTION ( 'NONE',  ( 0.000000000000000000, 0.1045284632676537068, 0.9945218953682734009 ) ) ;
#27549=CARTESIAN_POINT ( 'NONE',  ( -25.85392304583292855, 7.514126903508655531, 173.7688241862488212 ) ) ;
#27594=CARTESIAN_POINT ( 'NONE',  ( 26.77293948118378353, 6.014770499723010033, 169.2063755025576199 ) ) ;
#27607=CARTESIAN_POINT ( 'NONE',  ( 28.82186960331498327, 9.364793116373570925, 147.0999999999999943 ) ) ;
#27646=CIRCLE ( 'NONE', #30934, 26.79475375365586487 ) ;
#27705=ADVANCED_FACE ( 'NONE', ( #131387 ), #130367, .T. ) ;
#27716=CARTESIAN_POINT ( 'NONE',  ( 23.64874990377911246, -15.04272038711346937, 165.8682408883346397 ) ) ;
#27745=CARTESIAN_POINT ( 'NONE',  ( -21.58591991293347689, -5.574009794464002354, 173.3850233475172615 ) ) ;
#27758=CARTESIAN_POINT ( 'NONE',  ( -22.44159573604009950, -16.30477369853688430, 147.0750000027312012 ) ) ;
#27782=ORIENTED_EDGE ( 'NONE', *, *, #35307, .F. ) ;
#27827=EDGE_CURVE ( 'NONE', #66087, #104760, #87771, .T. ) ;
#27843=CIRCLE ( 'NONE', #53626, 25.62086810090349331 ) ;
#27898=CARTESIAN_POINT ( 'NONE',  ( 21.97154029300583389, -7.270820338085814072, 170.2141396987978226 ) ) ;
#27953=CARTESIAN_POINT ( 'NONE',  ( 17.14385361876520264, -23.59649016807271238, 142.0750000027311444 ) ) ;
#27994=CARTESIAN_POINT ( 'NONE',  ( -26.13941622279033794, -9.616497135380848604, 166.9083969906205027 ) ) ;
#28128=ORIENTED_EDGE ( 'NONE', *, *, #4069, .T. ) ;
#28149=CARTESIAN_POINT ( 'NONE',  ( 25.66098555633790923, -7.783268508282407794, 170.2231668181882185 ) ) ;
#28196=CARTESIAN_POINT ( 'NONE',  ( -19.49401214000077331, 12.39993551617566681, 169.9999999999999716 ) ) ;
#28237=CARTESIAN_POINT ( 'NONE',  ( -21.61802400803986757, 13.75099706318440340, 167.9999999999999432 ) ) ;
#28301=CARTESIAN_POINT ( 'NONE',  ( 8.571926809382603096, -26.38167802310801235, 143.4750000027312069 ) ) ;
#28389=DIRECTION ( 'NONE',  ( 1.000000000000000000, 0.000000000000000000, 0.000000000000000000 ) ) ;
#28462=CARTESIAN_POINT ( 'NONE',  ( 27.73933785331498214, 9.013057229001095294, 143.9750000027312069 ) ) ;
#28475=DIRECTION ( 'NONE',  ( -1.000000000000000000, 0.000000000000000000, 0.000000000000000000 ) ) ;
#28498=CARTESIAN_POINT ( 'NONE',  ( 1.988064558232696151E-15, -30.27659582821216588, 140.4843446568999923 ) ) ;
#28540=CARTESIAN_POINT ( 'NONE',  ( -20.19161698411414463, -19.96942110459088582, 140.0000000000000000 ) ) ;
#28583=CARTESIAN_POINT ( 'NONE',  ( 25.70602947687971707, 7.354137148287277270, 175.2376750527030538 ) ) ;
#28595=CARTESIAN_POINT ( 'NONE',  ( 8.906447517083050158, 27.41122689804195645, 143.4000000000000057 ) ) ;
#28619=CARTESIAN_POINT ( 'NONE',  ( -21.50819313649950359, 5.452397343345392500, 174.1340046013915241 ) ) ;
#28694=CARTESIAN_POINT ( 'NONE',  ( -24.57691432906831963, -7.727872488968206888, 167.2019946024424257 ) ) ;
#28782=CARTESIAN_POINT ( 'NONE',  ( 26.97479053218977185, 7.816291847812730786, 151.6430507545553894 ) ) ;
#28883=CARTESIAN_POINT ( 'NONE',  ( 21.82762259161258811, -6.010869995788711506, 172.1044450858201742 ) ) ;
#28937=CARTESIAN_POINT ( 'NONE',  ( -8.571926809382608425, 26.38167802310805854, 142.9750000027312069 ) ) ;
#28941=CARTESIAN_POINT ( 'NONE',  ( 22.44159573604009239, 16.30477369853692693, 146.5750000027312012 ) ) ;
#28976=CARTESIAN_POINT ( 'NONE',  ( -25.86526910843991445, -7.630673861715466799, 173.3900163844746203 ) ) ;
#28979=EDGE_CURVE ( 'NONE', #86852, #122599, #199576, .T. ) ;
#29183=ORIENTED_EDGE ( 'NONE', *, *, #92116, .T. ) ;
#29278=CARTESIAN_POINT ( 'NONE',  ( 27.73933785331498569, 2.768321779492822058E-14, 147.8750000027311842 ) ) ;
#29355=CARTESIAN_POINT ( 'NONE',  ( 23.29544513554940011, 16.92513159979228021, 143.1843446569000093 ) ) ;
#29419=ORIENTED_EDGE ( 'NONE', *, *, #160927, .F. ) ;
#29438=CARTESIAN_POINT ( 'NONE',  ( -5.359611314223446995E-15, 29.16686587814335496, 146.3750000027311842 ) ) ;
#29516=CARTESIAN_POINT ( 'NONE',  ( -11.82020350747949955, -25.60187801590574352, 139.9999999999999716 ) ) ;
#29844=ORIENTED_EDGE ( 'NONE', *, *, #125821, .T. ) ;
#29868=DIRECTION ( 'NONE',  ( 0.8437662581494463909, 0.5367108174878553184, 0.000000000000000000 ) ) ;
#29906=ORIENTED_EDGE ( 'NONE', *, *, #99562, .F. ) ;
#29913=CARTESIAN_POINT ( 'NONE',  ( -27.73933785331498925, 2.428612866367529932E-14, 141.3750000027311842 ) ) ;
#29917=CARTESIAN_POINT ( 'NONE',  ( 17.14385361876520264, 23.59649016807275856, 148.6750000027311387 ) ) ;
#29955=CARTESIAN_POINT ( 'NONE',  ( -25.62062145120300372, -9.171473787273981770, 171.1688781158170798 ) ) ;
#30152=CARTESIAN_POINT ( 'NONE',  ( -21.49230439284897543, -7.461675232480832420, 174.1505469413571063 ) ) ;
#30184=EDGE_CURVE ( 'NONE', #31781, #144449, #3266, .T. ) ;
#30255=CARTESIAN_POINT ( 'NONE',  ( -27.73933785331498925, 2.428612866367529932E-14, 142.8750000027311842 ) ) ;
#30330=ADVANCED_FACE ( 'NONE', ( #60756 ), #184121, .T. ) ;
#30419=CARTESIAN_POINT ( 'NONE',  ( -27.73933785331498925, 2.428612866367529932E-14, 142.8750000027311842 ) ) ;
#30455=CARTESIAN_POINT ( 'NONE',  ( -23.29544513554940721, -16.92513159979223403, 140.1843446569000093 ) ) ;
#30498=CARTESIAN_POINT ( 'NONE',  ( -25.70602947687972417, 7.354137148287277270, 175.2376750527030538 ) ) ;
#30558=CARTESIAN_POINT ( 'NONE',  ( -28.82186960331499392, 9.364793116373565596, 143.9000000000000057 ) ) ;
#30560=AXIS2_PLACEMENT_3D ( 'NONE', #197298, #198278, #199274 ) ;
#30571=CARTESIAN_POINT ( 'NONE',  ( 23.64874990377911246, -15.04272038711346937, 165.8682408883346397 ) ) ;
#30629=ORIENTED_EDGE ( 'NONE', *, *, #162141, .T. ) ;
#30658=CARTESIAN_POINT ( 'NONE',  ( -24.30454888808800362, -2.781629622375087152, 174.5654150192188183 ) ) ;
#30844=CIRCLE ( 'NONE', #56696, 5.000000000000001776 ) ;
#30850=ORIENTED_EDGE ( 'NONE', *, *, #99562, .T. ) ;
#30865=DIRECTION ( 'NONE',  ( 1.000000000000000000, 0.000000000000000000, -0.000000000000000000 ) ) ;
#30910=CARTESIAN_POINT ( 'NONE',  ( -17.14385361876520619, 23.59649016807275856, 145.0750000027311728 ) ) ;
#30914=CARTESIAN_POINT ( 'NONE',  ( -17.14385361876520264, -23.59649016807271593, 147.6750000027311671 ) ) ;
#30934=AXIS2_PLACEMENT_3D ( 'NONE', #67312, #82464, #99644 ) ;
#30949=CARTESIAN_POINT ( 'NONE',  ( -26.45594755429640799, -8.318738267476385673, 167.5492909577823752 ) ) ;
#31021=ORIENTED_EDGE ( 'NONE', *, *, #105010, .F. ) ;
#31087=VERTEX_POINT ( 'NONE', #88120 ) ;
#31101=CARTESIAN_POINT ( 'NONE',  ( 17.07321893155272363, 22.25586454244016110, 139.9999999999999432 ) ) ;
#31188=CARTESIAN_POINT ( 'NONE',  ( -21.96844466259092243, 7.174710485416647465, 170.3366942299255413 ) ) ;
#31212=ORIENTED_EDGE ( 'NONE', *, *, #27827, .T. ) ;
#31253=CARTESIAN_POINT ( 'NONE',  ( -22.44159573604010305, 16.30477369853692338, 142.6750000027311671 ) ) ;
#31266=CARTESIAN_POINT ( 'NONE',  ( 27.96892006433830247, -7.184979517970438323, 161.0508495487522680 ) ) ;
#31324=ORIENTED_EDGE ( 'NONE', *, *, #9833, .T. ) ;
#31328=AXIS2_PLACEMENT_3D ( 'NONE', #49205, #110863, #157379 ) ;
#31415=CARTESIAN_POINT ( 'NONE',  ( -17.14385361876520264, -23.59649016807271593, 143.1750000027311671 ) ) ;
#31423=CARTESIAN_POINT ( 'NONE',  ( 22.72581825106559350, -12.75361973299573926, 165.5645137041833550 ) ) ;
#31553=CARTESIAN_POINT ( 'NONE',  ( 8.906447517083050158, 27.41122689804195645, 141.4000000000000057 ) ) ;
#31566=CARTESIAN_POINT ( 'NONE',  ( 21.93180397000137205, -9.000796715316949914, 171.3297436093415058 ) ) ;
#31570=CARTESIAN_POINT ( 'NONE',  ( 8.898068258721465895, 27.38543819252877398, 143.6656553485623817 ) ) ;
#31572=FILL_AREA_STYLE ('',( #81037 ) ) ;
#31576=CARTESIAN_POINT ( 'NONE',  ( -24.81835880841865816, 6.052260367207988878, 168.4265213779230521 ) ) ;
#31605=CYLINDRICAL_SURFACE ( 'NONE', #160230, 5.000000000000004441 ) ;
#31651=CARTESIAN_POINT ( 'NONE',  ( -24.85114155361886290, -5.582993631595906336, 168.8590791472331034 ) ) ;
#31673=EDGE_CURVE ( 'NONE', #122542, #87433, #43521, .T. ) ;
#31781=VERTEX_POINT ( 'NONE', #194096 ) ;
#31842=DIRECTION ( 'NONE',  ( -1.000000000000000000, -0.000000000000000000, 0.000000000000000000 ) ) ;
#31870=ORIENTED_EDGE ( 'NONE', *, *, #16216, .T. ) ;
#31904=CARTESIAN_POINT ( 'NONE',  ( -22.44159573604010305, 16.30477369853692338, 143.1750000027311671 ) ) ;
#31938=CARTESIAN_POINT ( 'NONE',  ( -26.26139018963107929, -3.005588016160666953, 174.9127113745526572 ) ) ;
#31966=VERTEX_POINT ( 'NONE', #51560 ) ;
#32058=EDGE_CURVE ( 'NONE', #162084, #199519, #53553, .T. ) ;
#32094=CARTESIAN_POINT ( 'NONE',  ( -18.87309089550571883, 21.74014469927720228, 140.0000000000000284 ) ) ;
#32183=CARTESIAN_POINT ( 'NONE',  ( -22.24685556490158689, 12.75834802357609910, 167.9013491530738520 ) ) ;
#32247=CARTESIAN_POINT ( 'NONE',  ( -22.44159573604010305, 16.30477369853692338, 146.6750000027311671 ) ) ;
#32287=DIRECTION ( 'NONE',  ( -1.000000000000000000, 0.000000000000000000, -0.000000000000000000 ) ) ;
#32377=CARTESIAN_POINT ( 'NONE',  ( -28.79475375365586842, 9.355982642739222754, 149.8843446568999980 ) ) ;
#32409=CARTESIAN_POINT ( 'NONE',  ( 22.44159573604009239, 16.30477369853692693, 140.0750000027311728 ) ) ;
#32424=EDGE_CURVE ( 'NONE', #172658, #119499, #182368, .T. ) ;
#32538=CARTESIAN_POINT ( 'NONE',  ( -23.58953014017658489, -7.613468834709958166, 172.7063272879299234 ) ) ;
#32547=CARTESIAN_POINT ( 'NONE',  ( 1.993301997531345292E-15, -30.30510711980685912, 140.5000000000000000 ) ) ;
#32560=CARTESIAN_POINT ( 'NONE',  ( 21.36928693577338478, -7.422813773936193016, 174.5222352431090087 ) ) ;
#32564=CARTESIAN_POINT ( 'NONE',  ( -28.79475375365497314, 9.355982642740462651, 144.1656553485623533 ) ) ;
#32591=EDGE_LOOP ( 'NONE', ( #2848, #92953, #23342, #132518, #55758, #177128, #84991, #51494, #34137, #91301, #50189, #138708, #21437 ) ) ;
#32643=CARTESIAN_POINT ( 'NONE',  ( -24.14511064691488329, -7.743397529681040226, 169.7652520481184126 ) ) ;
#32661=CARTESIAN_POINT ( 'NONE',  ( 22.44159573604009594, -16.30477369853687364, 148.1750000027311671 ) ) ;
#32732=FACE_OUTER_BOUND ( 'NONE', #161272, .T. ) ;
#32812=CARTESIAN_POINT ( 'NONE',  ( 27.73881904903412021, -0.9222476559034787913, 140.0000000000000000 ) ) ;
#32832=ORIENTED_EDGE ( 'NONE', *, *, #1535, .T. ) ;
#32884=FACE_OUTER_BOUND ( 'NONE', #143534, .T. ) ;
#33066=CARTESIAN_POINT ( 'NONE',  ( 10.65970682939788716, -25.60940286011448919, 139.9999999999999716 ) ) ;
#33138=CARTESIAN_POINT ( 'NONE',  ( -21.49230329115315996, 7.461674882483885440, 174.1505502713556837 ) ) ;
#33178=CARTESIAN_POINT ( 'NONE',  ( -23.34492853952160019, 11.48509598731696890, 165.7658222004386914 ) ) ;
#33228=CONICAL_SURFACE ( 'NONE', #65539, 28.85599147140294107, 0.1745329251994333364 ) ;
#33245=CARTESIAN_POINT ( 'NONE',  ( -17.14385361876520264, -23.59649016807271593, 139.1750000027311955 ) ) ;
#33280=CARTESIAN_POINT ( 'NONE',  ( 23.29544513554940366, -16.92513159979222337, 147.0656553485623590 ) ) ;
#33329=CARTESIAN_POINT ( 'NONE',  ( -26.33867313280595468, -8.832717389288097465, 167.2809140985657450 ) ) ;
#33365=ORIENTED_EDGE ( 'NONE', *, *, #13191, .F. ) ;
#33382=( BOUNDED_CURVE ( )  B_SPLINE_CURVE ( 2, ( #75955, #61766, #30455, #92103, #184145, #28498, #13306, #93102, #170953, #121462, #16284 ),
 .UNSPECIFIED., .F., .T. ) 
 B_SPLINE_CURVE_WITH_KNOTS ( ( 3, 2, 2, 2, 2, 3 ),
 ( 0.001627243422692786377, 0.02000000000000003858, 0.04000000000000008410, 0.06000000000000012268, 0.08000000000000004330, 0.1000000000000000888 ),
 .UNSPECIFIED. ) 
 CURVE ( )  GEOMETRIC_REPRESENTATION_ITEM ( )  RATIONAL_B_SPLINE_CURVE ( ( 0.9926836962356841987, 0.9550386643922726959, 1.000000000000000000, 0.9510565162951535312, 1.000000000000000000, 0.9510565162951535312, 1.000000000000000000, 0.9510565162951535312, 1.000000000000000000, 0.9510565162951533091, 1.000000000000000222 ) ) 
 REPRESENTATION_ITEM ( '' )  );
#33383=VERTEX_POINT ( 'NONE', #187645 ) ;
#33439=CARTESIAN_POINT ( 'NONE',  ( 23.14225647005876851, -5.657937718899350266, 172.1775255543084882 ) ) ;
#33529=CARTESIAN_POINT ( 'NONE',  ( -24.69864206457980771, -7.736332803992566731, 171.5373547058827626 ) ) ;
#33552=CARTESIAN_POINT ( 'NONE',  ( 25.47140278216198439, -9.703455644538477642, 170.7619267275323409 ) ) ;
#33569=LINE ( 'NONE', #123570, #163225 ) ;
#33689=DIRECTION ( 'NONE',  ( 0.000000000000000000, 0.9945218953682734009, 0.1045284632676537068 ) ) ;
#33712=DIRECTION ( 'NONE',  ( 0.1039620511844979445, -0.1039620511844979445, -0.9891328443778539814 ) ) ;
#33729=EDGE_CURVE ( 'NONE', #31966, #101974, #82363, .T. ) ;
#33758=VERTEX_POINT ( 'NONE', #174448 ) ;
#33772=ORIENTED_EDGE ( 'NONE', *, *, #175018, .T. ) ;
#34080=CARTESIAN_POINT ( 'NONE',  ( -17.07606455188742345, 23.12338299651413820, 140.0000000000000284 ) ) ;
#34091=EDGE_CURVE ( 'NONE', #88085, #139693, #6149, .T. ) ;
#34137=ORIENTED_EDGE ( 'NONE', *, *, #16216, .F. ) ;
#34168=CARTESIAN_POINT ( 'NONE',  ( -24.72709851008508863, 6.869189314505790733, 167.7661538690215650 ) ) ;
#34234=CARTESIAN_POINT ( 'NONE',  ( 22.44159573604009594, -16.30477369853687364, 139.6750000027311955 ) ) ;
#34392=CIRCLE ( 'NONE', #50560, 27.29906736325805028 ) ;
#34462=LINE ( 'NONE', #66778, #21477 ) ;
#34545=CARTESIAN_POINT ( 'NONE',  ( 25.73063820182080264, -8.702599028576591067, 171.6270364942811284 ) ) ;
#34549=CARTESIAN_POINT ( 'NONE',  ( -28.85599147140294463, 2.075228890450760606E-14, 149.6527036446661327 ) ) ;
#34551=PRESENTATION_STYLE_ASSIGNMENT (( #188247 ) ) ;
#34558=CARTESIAN_POINT ( 'NONE',  ( 24.81835718235489807, 6.052279806424484931, 168.4265042179603142 ) ) ;
#34596=CARTESIAN_POINT ( 'NONE',  ( -26.03370437638687918, 6.875205692009823011, 160.5968874236874910 ) ) ;
#34624=CARTESIAN_POINT ( 'NONE',  ( -23.31738231874055245, -16.94106989632524574, 144.4500000054623854 ) ) ;
#34840=VERTEX_POINT ( 'NONE', #184405 ) ;
#34909=DIRECTION ( 'NONE',  ( 0.000000000000000000, 0.000000000000000000, -1.000000000000000000 ) ) ;
#34941=VERTEX_POINT ( 'NONE', #190364 ) ;
#35037=LINE ( 'NONE', #130005, #15336 ) ;
#35155=CARTESIAN_POINT ( 'NONE',  ( -21.93180397000138626, 7.641141194970188621, 169.8616410530809731 ) ) ;
#35161=CIRCLE ( 'NONE', #180547, 25.62086810090349331 ) ;
#35192=EDGE_CURVE ( 'NONE', #35378, #90049, #62896, .T. ) ;
#35222=CARTESIAN_POINT ( 'NONE',  ( 27.73933785331498214, 9.013057229001095294, 139.9750000027311501 ) ) ;
#35236=CARTESIAN_POINT ( 'NONE',  ( 27.96619922901622246, -7.272069078172575196, 160.9422763814157804 ) ) ;
#35301=CIRCLE ( 'NONE', #41821, 2.999999999999999556 ) ;
#35307=EDGE_CURVE ( 'NONE', #119499, #172658, #159009, .T. ) ;
#35330=ORIENTED_EDGE ( 'NONE', *, *, #19482, .F. ) ;
#35332=DIRECTION ( 'NONE',  ( 0.000000000000000000, 0.000000000000000000, -1.000000000000000000 ) ) ;
#35346=DIRECTION ( 'NONE',  ( -0.1045284632676537068, 0.000000000000000000, 0.9945218953682734009 ) ) ;
#35378=VERTEX_POINT ( 'NONE', #84159 ) ;
#35387=CARTESIAN_POINT ( 'NONE',  ( -27.73933785331498925, 9.013057229001089965, 140.7750000027311899 ) ) ;
#35448=CARTESIAN_POINT ( 'NONE',  ( 22.37486833544152631, 13.37560805684319121, 165.5209445320979569 ) ) ;
#35467=B_SPLINE_CURVE_WITH_KNOTS ( 'NONE', 3,
 ( #75598, #32094, #77590, #93751, #34080, #14936, #198959, #155432, #46263, #62409, #186792, #94744, #122100, #124079, #79580, #16922, #78575, #184777, #171600, #2738, #95738, #64415, #187780, #49250, #92749, #183790, #169603, #45277, #31101, #76596, #96720, #146217, #37052, #97702, #5712, #111908, #50252, #83544 ),
 .UNSPECIFIED., .F., .F.,
 ( 4, 2, 2, 2, 2, 2, 2, 2, 2, 2, 2, 2, 2, 2, 2, 2, 2, 2, 4 ),
 ( 0.001405631271041209943, 0.003109748753336292505, 0.004813866235631374633, 0.008222101200221529349, 0.01163033616481168493, 0.01333445364710676533, 0.01503857112940184398, 0.02185504105858216903, 0.02355915854087725289, 0.02526327602317233675, 0.02867151098776249754, 0.03548798091694280871, 0.03719209839923789257, 0.03889621588153296255, 0.04230445084612311640, 0.04571268581071328413, 0.04741680329300836799, 0.04912092077530345186, 0.05593739070448378037 ),
 .UNSPECIFIED. ) ;
#35512=ORIENTED_EDGE ( 'NONE', *, *, #178481, .F. ) ;
#35515=CARTESIAN_POINT ( 'NONE',  ( -26.12113310390730092, 7.698689789033755559, 169.4288210027979460 ) ) ;
#35536=CARTESIAN_POINT ( 'NONE',  ( 26.61723430050320616, -3.645106422947246738, 172.4622069319862590 ) ) ;
#35540=CARTESIAN_POINT ( 'NONE',  ( 28.96383432292632065, 7.816291847812730786, 151.8521076810907005 ) ) ;
#35559=CARTESIAN_POINT ( 'NONE',  ( -27.73933785331498925, 9.013057229001088189, 140.7750000027311899 ) ) ;
#35595=VERTEX_POINT ( 'NONE', #161018 ) ;
#35615=CARTESIAN_POINT ( 'NONE',  ( 17.14385361876520264, -23.59649016807271238, 144.0750000027311444 ) ) ;
#35616=CARTESIAN_POINT ( 'NONE',  ( -8.906447517083060816, 27.41122689804195645, 143.8500000054623911 ) ) ;
#35693=CARTESIAN_POINT ( 'NONE',  ( -22.96528548301343520, -5.795830589372932273, 190.0000000000000000 ) ) ;
#35798=UNCERTAINTY_MEASURE_WITH_UNIT (LENGTH_MEASURE( 1.000000000000000082E-05 ), #127353, 'distance_accuracy_value', 'NONE');
#35838=CARTESIAN_POINT ( 'NONE',  ( -28.79475375365586842, 2.428612866367529932E-14, 140.2656553485623760 ) ) ;
#35859=FACE_OUTER_BOUND ( 'NONE', #168887, .T. ) ;
#35888=CARTESIAN_POINT ( 'NONE',  ( 25.51209292918185412, -5.276535733812600881, 165.5596888358905687 ) ) ;
#35900=CARTESIAN_POINT ( 'NONE',  ( -25.80209238092669821, -7.370998251473047880, 174.5109820657624766 ) ) ;
#36099=CARTESIAN_POINT ( 'NONE',  ( -21.61802400803983559, -13.75099706318440340, 167.9999999999999432 ) ) ;
#36141=CARTESIAN_POINT ( 'NONE',  ( -24.04614410382104595, 5.408324479811685848, 174.2944578187875209 ) ) ;
#36198=CARTESIAN_POINT ( 'NONE',  ( 21.83923006935332012, 7.858462611068595116, 172.8812894384829519 ) ) ;
#36239=CARTESIAN_POINT ( 'NONE',  ( 22.03292204642282925, 7.478118144893481478, 173.9941030799743089 ) ) ;
#36269=ORIENTED_EDGE ( 'NONE', *, *, #24747, .F. ) ;
#36312=DIRECTION ( 'NONE',  ( -1.000000000000000000, 0.000000000000000000, -0.000000000000000000 ) ) ;
#36421=ADVANCED_FACE ( 'NONE', ( #147866 ), #150859, .T. ) ;
#36529=CARTESIAN_POINT ( 'NONE',  ( 24.93942350307310107, -7.769968609432603479, 171.2173313942149377 ) ) ;
#36541=CARTESIAN_POINT ( 'NONE',  ( 8.571926809382603096, -26.38167802310801235, 143.4750000027312069 ) ) ;
#36547=EDGE_CURVE ( 'NONE', #158282, #75891, #59158, .T. ) ;
#36598=CARTESIAN_POINT ( 'NONE',  ( 28.82186960331499392, -9.364793116373510529, 143.1500000054623740 ) ) ;
#36612=CARTESIAN_POINT ( 'NONE',  ( -22.44159573604009950, -16.30477369853688430, 145.5750000027311728 ) ) ;
#36686=CARTESIAN_POINT ( 'NONE',  ( 23.29544513554940366, -16.92513159979222337, 143.0656553485623874 ) ) ;
#36723=ORIENTED_EDGE ( 'NONE', *, *, #123538, .F. ) ;
#36725=CARTESIAN_POINT ( 'NONE',  ( 23.35043118190687750, 14.19381810411953992, 169.8796877288296514 ) ) ;
#36764=CARTESIAN_POINT ( 'NONE',  ( -8.898068258721467672, -27.38543819252872069, 144.3843446568999980 ) ) ;
#36853=CARTESIAN_POINT ( 'NONE',  ( 19.49401214000073779, -12.39993551617566503, 169.9999999999999716 ) ) ;
#36961=EDGE_CURVE ( 'NONE', #34941, #114568, #105011, .T. ) ;
#37011=CARTESIAN_POINT ( 'NONE',  ( 26.58496454516998142, -7.626754437231455519, 167.9682100371138915 ) ) ;
#37044=VECTOR ( 'NONE', #183640, 1000.000000000000000 ) ;
#37052=CARTESIAN_POINT ( 'NONE',  ( 21.08520368033286729, 18.30394477064738012, 139.9999999999999716 ) ) ;
#37099=CARTESIAN_POINT ( 'NONE',  ( -23.34492853952158242, -11.48509598731697068, 165.7658222004386914 ) ) ;
#37106=ORIENTED_EDGE ( 'NONE', *, *, #99048, .T. ) ;
#37136=CARTESIAN_POINT ( 'NONE',  ( 23.19706360625304598, -11.80427776162576592, 165.7059442611692361 ) ) ;
#37184=CARTESIAN_POINT ( 'NONE',  ( 23.71437531004595911, 10.61261859643795091, 165.9743991446059965 ) ) ;
#37244=CARTESIAN_POINT ( 'NONE',  ( -23.29544513554940721, -16.92513159979223758, 146.4656553485623647 ) ) ;
#37318=CARTESIAN_POINT ( 'NONE',  ( 22.94331271462294453, 0.000000000000000000, 190.0000000000000000 ) ) ;
#37352=VERTEX_POINT ( 'NONE', #129214 ) ;
#37403=VECTOR ( 'NONE', #159029, 1000.000000000000000 ) ;
#37442=CARTESIAN_POINT ( 'NONE',  ( 21.61802400803986757, 13.75099706318440340, 167.9999999999999432 ) ) ;
#37548=CARTESIAN_POINT ( 'NONE',  ( -21.77012268027506181, -5.483007391792980911, 173.8427694444997371 ) ) ;
#37552=CARTESIAN_POINT ( 'NONE',  ( -5.359611314223446995E-15, 29.16686587814335851, 144.3750000027311842 ) ) ;
#37607=CARTESIAN_POINT ( 'NONE',  ( 8.571926809382603096, -26.38167802310801235, 139.9750000027311785 ) ) ;
#37609=CARTESIAN_POINT ( 'NONE',  ( -28.82186960331499037, 2.428612866367529932E-14, 140.2500000054623683 ) ) ;
#37622=CARTESIAN_POINT ( 'NONE',  ( -8.571926809382601320, -26.38167802310801591, 145.7750000027311899 ) ) ;
#37694=CARTESIAN_POINT ( 'NONE',  ( -25.73063820182138528, 8.702599028576308626, 171.6270364942766946 ) ) ;
#37696=CARTESIAN_POINT ( 'NONE',  ( -28.79475375365586842, 2.428612866367529932E-14, 142.2656553485623760 ) ) ;
#37739=CARTESIAN_POINT ( 'NONE',  ( 19.49401214000076976, 12.39993551617566681, 169.9999999999999716 ) ) ;
#37743=ORIENTED_EDGE ( 'NONE', *, *, #165138, .F. ) ;
#37826=EDGE_LOOP ( 'NONE', ( #149635, #77149 ) ) ;
#37829=LINE ( 'NONE', #181356, #86448 ) ;
#37840=CARTESIAN_POINT ( 'NONE',  ( -25.41560487745637076, 11.65347601360405605, 166.2639678467665476 ) ) ;
#37861=EDGE_LOOP ( 'NONE', ( #170103, #195316, #173275 ) ) ;
#37863=DIRECTION ( 'NONE',  ( 1.000000000000000000, 0.000000000000000000, 0.000000000000000000 ) ) ;
#37867=DIRECTION ( 'NONE',  ( 0.000000000000000000, 0.000000000000000000, -1.000000000000000000 ) ) ;
#38051=CARTESIAN_POINT ( 'NONE',  ( 8.898068258721464119, 27.38543819252877398, 147.3843446568999980 ) ) ;
#38062=CARTESIAN_POINT ( 'NONE',  ( 27.96784714409925243, 7.240004476324741312, 160.9788157999919918 ) ) ;
#38111=CARTESIAN_POINT ( 'NONE',  ( -19.83802472612924106, -12.02135855756094251, 167.9999999999999716 ) ) ;
#38151=CARTESIAN_POINT ( 'NONE',  ( 24.29042230868020624, -8.936166115090800943, 166.5611006352801553 ) ) ;
#38231=CARTESIAN_POINT ( 'NONE',  ( 27.93385843979449845, -7.419916809875269692, 160.9064084702648643 ) ) ;
#38251=CARTESIAN_POINT ( 'NONE',  ( 21.58591991293347689, 5.574009794464005019, 173.3850233475172615 ) ) ;
#38325=CYLINDRICAL_SURFACE ( 'NONE', #70994, 7.000000000000006217 ) ;
#38336=CARTESIAN_POINT ( 'NONE',  ( 27.39399371936739769, 5.109217719438622574, 166.7881433183870001 ) ) ;
#38387=DIRECTION ( 'NONE',  ( -1.000000000000000000, 0.000000000000000000, 0.000000000000000000 ) ) ;
#38420=EDGE_CURVE ( 'NONE', #87433, #135144, #27843, .T. ) ;
#38559=CARTESIAN_POINT ( 'NONE',  ( -22.87925077421024156, -5.621762139875928099, 172.5226062014847059 ) ) ;
#38564=CARTESIAN_POINT ( 'NONE',  ( 27.73933785331498569, 9.013057229001093518, 141.9750000027311785 ) ) ;
#38620=CARTESIAN_POINT ( 'NONE',  ( 17.81289503416611453, -24.51734667627695785, 138.9500000054623570 ) ) ;
#38634=CARTESIAN_POINT ( 'NONE',  ( 27.73933785331498569, 9.013057229001093518, 146.4750000027311501 ) ) ;
#38662=ADVANCED_FACE ( 'NONE', ( #21732 ), #72997, .T. ) ;
#38705=CARTESIAN_POINT ( 'NONE',  ( -23.03403192006594935, 14.65170476119024201, 169.9999999999999716 ) ) ;
#38787=CARTESIAN_POINT ( 'NONE',  ( 28.79475375365586132, 2.781246896534039337E-14, 144.9843446568999923 ) ) ;
#38801=AXIS2_PLACEMENT_3D ( 'NONE', #127326, #35332, #36312 ) ;
#38866=DIRECTION ( 'NONE',  ( 0.000000000000000000, 0.000000000000000000, 1.000000000000000000 ) ) ;
#39028=DIRECTION ( 'NONE',  ( -0.1039620511844979306, -0.1039620511844979306, -0.9891328443778538704 ) ) ;
#39057=CARTESIAN_POINT ( 'NONE',  ( 27.89963664982190750, 6.788868650204036292, 161.9772721943422482 ) ) ;
#39100=CARTESIAN_POINT ( 'NONE',  ( -27.73933785331498925, 9.013057229001089965, 147.2750000027311614 ) ) ;
#39106=CARTESIAN_POINT ( 'NONE',  ( -21.04946095171256104, -10.24435024061084931, 168.3368280404223754 ) ) ;
#39142=CARTESIAN_POINT ( 'NONE',  ( 24.66578506923904968, -3.377805382905422427, 172.1149105766468210 ) ) ;
#39263=DIRECTION ( 'NONE',  ( -1.000000000000000000, 0.000000000000000000, 0.000000000000000000 ) ) ;
#39278=CARTESIAN_POINT ( 'NONE',  ( -25.89282049031357857, -12.30142083841955269, 140.0000000000000000 ) ) ;
#39280=CARTESIAN_POINT ( 'NONE',  ( -20.48541513753863796, 11.15937153969632156, 168.1083253156164119 ) ) ;
#39348=SHAPE_REPRESENTATION_RELATIONSHIP ( 'NONE' , 'NONE' ,  #112845, #15828 ) ;
#39390=CARTESIAN_POINT ( 'NONE',  ( -3.573655867282028392E-15, 2.428612866367529932E-14, 167.9999999999999716 ) ) ;
#39427=CARTESIAN_POINT ( 'NONE',  ( -27.77709992218201052, -7.633332386735008690, 161.4489275245939268 ) ) ;
#39440=CARTESIAN_POINT ( 'NONE',  ( 24.30454888808800007, 2.781629622375082267, 174.5654150192188183 ) ) ;
#39497=ORIENTED_EDGE ( 'NONE', *, *, #176927, .T. ) ;
#39609=CARTESIAN_POINT ( 'NONE',  ( 28.82186960331498327, 2.781578969918950771E-14, 141.2500000054623683 ) ) ;
#39622=CARTESIAN_POINT ( 'NONE',  ( 22.44159573604009594, -16.30477369853687364, 146.1750000027311671 ) ) ;
#39691=CARTESIAN_POINT ( 'NONE',  ( -25.93326183087854275, 10.28624940747392991, 166.6531433017870540 ) ) ;
#39733=CARTESIAN_POINT ( 'NONE',  ( 25.93326183087853565, 10.28624940747392991, 166.6531433017870540 ) ) ;
#39744=CARTESIAN_POINT ( 'NONE',  ( 28.82186960331499392, -9.364793116373510529, 146.8999999999999773 ) ) ;
#39803=LINE ( 'NONE', #101469, #166765 ) ;
#39809=AXIS2_PLACEMENT_3D ( 'NONE', #50880, #82175, #112538 ) ;
#39824=EDGE_LOOP ( 'NONE', ( #172271, #61109, #183008, #105635, #98400, #82231 ) ) ;
#39888=CARTESIAN_POINT ( 'NONE',  ( -21.94566984220701755, -7.593969325705130835, 169.8906363267648771 ) ) ;
#39900=B_SPLINE_CURVE_WITH_KNOTS ( 'NONE', 3,
 ( #34558, #17404, #116133, #126554, #115133, #192985, #94227, #79061, #160638, #70637, #130276, #186271 ),
 .UNSPECIFIED., .F., .F.,
 ( 4, 2, 2, 2, 2, 4 ),
 ( -0.003994749848159050501, -0.003130422923337882173, -0.002266095998516713846, -0.0005374421488743771902, 0.001191211700767959465, 0.002919865550410296121 ),
 .UNSPECIFIED. ) ;
#39904=CARTESIAN_POINT ( 'NONE',  ( -27.73933785331498925, -9.013057229001049109, 146.9750000027311785 ) ) ;
#40037=CARTESIAN_POINT ( 'NONE',  ( 28.79475375365567302, 9.355982642739496313, 147.0843446568999866 ) ) ;
#40132=CARTESIAN_POINT ( 'NONE',  ( 21.94905633995417915, -7.481063542984161430, 170.0146117665088923 ) ) ;
#40296=CARTESIAN_POINT ( 'NONE',  ( 26.25049742697153832, -7.664248127782749442, 169.1476266185236454 ) ) ;
#40329=EDGE_LOOP ( 'NONE', ( #103946, #161702, #108610, #15047 ) ) ;
#40367=CARTESIAN_POINT ( 'NONE',  ( 23.84690145917535631, -10.26550538186640082, 166.0764395470883983 ) ) ;
#40540=AXIS2_PLACEMENT_3D ( 'NONE', #168891, #125392, #188071 ) ;
#40618=CARTESIAN_POINT ( 'NONE',  ( -27.73933785331498925, 9.013057229001089965, 141.2750000027311614 ) ) ;
#40619=CARTESIAN_POINT ( 'NONE',  ( 8.906447517083057264, -27.41122689804191026, 140.8500000054623911 ) ) ;
#40632=CARTESIAN_POINT ( 'NONE',  ( -8.571926809382601320, -26.38167802310801591, 143.7750000027311899 ) ) ;
#40701=CARTESIAN_POINT ( 'NONE',  ( -25.52568752982265821, 9.519068727184937018, 170.8917780290381927 ) ) ;
#40744=CARTESIAN_POINT ( 'NONE',  ( 19.83801684532418008, 12.12952959760495730, 169.9999999999999716 ) ) ;
#40756=CARTESIAN_POINT ( 'NONE',  ( 23.31738231874054534, 16.94106989632529192, 147.1999999999999886 ) ) ;
#40789=CARTESIAN_POINT ( 'NONE',  ( 8.898068258721465895, 27.38543819252877398, 145.6656553485624102 ) ) ;
#40849=VECTOR ( 'NONE', #101339, 1000.000000000000114 ) ;
#40913=CARTESIAN_POINT ( 'NONE',  ( -27.73933785331498925, 9.013057229001088189, 144.7750000027311614 ) ) ;
#41080=( BOUNDED_CURVE ( )  B_SPLINE_CURVE ( 2, ( #41374, #133370, #88860, #163724, #13032, #89860, #86868, #105032, #137349, #120192, #44357 ),
 .UNSPECIFIED., .F., .T. ) 
 B_SPLINE_CURVE_WITH_KNOTS ( ( 3, 2, 2, 2, 2, 3 ),
 ( 0.6000000000000005329, 0.6200000000000005507, 0.6400000000000005684, 0.6600000000000005862, 0.6800000000000006040, 0.7000000000000006217 ),
 .UNSPECIFIED. ) 
 CURVE ( )  GEOMETRIC_REPRESENTATION_ITEM ( )  RATIONAL_B_SPLINE_CURVE ( ( 0.9999999999999986677, 0.9510565162951548634, 1.000000000000000000, 0.9510565162951535312, 1.000000000000000000, 0.9510565162951535312, 1.000000000000000000, 0.9510565162951535312, 1.000000000000000000, 0.9510565162951518658, 1.000000000000001554 ) ) 
 REPRESENTATION_ITEM ( '' )  );
#41108=CARTESIAN_POINT ( 'NONE',  ( -5.359611314223446995E-15, 29.16686587814335496, 146.8750000027311273 ) ) ;
#41115=PLANE ( 'NONE',  #12145 ) ;
#41152=CARTESIAN_POINT ( 'NONE',  ( 24.10884208241212434, -5.471882726980744849, 173.8287385965643352 ) ) ;
#41189=VECTOR ( 'NONE', #168231, 1000.000000000000000 ) ;
#41286=CARTESIAN_POINT ( 'NONE',  ( -28.21656721799290324, -5.378544878440105315, 140.0000000000000568 ) ) ;
#41310=AXIS2_PLACEMENT_3D ( 'NONE', #158534, #189884, #160531 ) ;
#41332=CARTESIAN_POINT ( 'NONE',  ( -21.38418241377624085, 5.438282248597754887, 174.2683007571264113 ) ) ;
#41352=CARTESIAN_POINT ( 'NONE',  ( -21.65274598442066889, 9.891030456500295998, 170.6639841963363438 ) ) ;
#41357=CARTESIAN_POINT ( 'NONE',  ( -3.573655867282028392E-15, 2.428612866367529932E-14, 155.0000000000000000 ) ) ;
#41374=CARTESIAN_POINT ( 'NONE',  ( -28.79475375365586842, 2.428612866367530248E-14, 145.9843446568999923 ) ) ;
#41434=CARTESIAN_POINT ( 'NONE',  ( -28.79475375365581158, -9.355982642739276045, 142.0843446569000434 ) ) ;
#41455=CARTESIAN_POINT ( 'NONE',  ( 21.92083080610932200, 6.374575339256159268, 171.4095429173257514 ) ) ;
#41524=CARTESIAN_POINT ( 'NONE',  ( -28.79475375365490564, 9.355982642740551469, 142.1656553485624102 ) ) ;
#41532=CARTESIAN_POINT ( 'NONE',  ( -28.79475375365586842, 2.428612866367529932E-14, 155.0000000000000000 ) ) ;
#41551=CARTESIAN_POINT ( 'NONE',  ( -27.46925885783797838, 7.746560145625151605, 162.9586723222901981 ) ) ;
#41627=CARTESIAN_POINT ( 'NONE',  ( 1.784210473542230573E-15, -29.16686587814331588, 147.3750000027311842 ) ) ;
#41669=DIRECTION ( 'NONE',  ( 0.000000000000000000, 0.000000000000000000, 1.000000000000000000 ) ) ;
#41709=CARTESIAN_POINT ( 'NONE',  ( -21.35462415990330953, 10.43496131973800090, 170.3924512066482748 ) ) ;
#41763=CARTESIAN_POINT ( 'NONE',  ( 17.14385361876520264, -23.59649016807271238, 140.0750000027311728 ) ) ;
#41821=AXIS2_PLACEMENT_3D ( 'NONE', #91110, #88149, #26506 ) ;
#41869=EDGE_LOOP ( 'NONE', ( #151698, #146513, #85345, #78076 ) ) ;
#41909=LINE ( 'NONE', #102573, #7551 ) ;
#41922=CARTESIAN_POINT ( 'NONE',  ( -8.571926809382608425, 26.38167802310805854, 146.4750000027311785 ) ) ;
#42114=CARTESIAN_POINT ( 'NONE',  ( -17.14385361876520619, 23.59649016807275856, 149.0750000027311728 ) ) ;
#42155=CARTESIAN_POINT ( 'NONE',  ( 21.88033147701266046, -7.974798826776969385, 169.5716465351769955 ) ) ;
#42332=ADVANCED_FACE ( 'NONE', ( #123796 ), #46985, .F. ) ;
#42375=CARTESIAN_POINT ( 'NONE',  ( 24.81835880841864039, -6.052260367207979996, 168.4265213779230521 ) ) ;
#42424=ADVANCED_FACE ( 'NONE', ( #177313 ), #8444, .T. ) ;
#42451=CARTESIAN_POINT ( 'NONE',  ( 24.83221077041948988, 4.296110748034003279, 170.3917201292229322 ) ) ;
#42619=CARTESIAN_POINT ( 'NONE',  ( -17.14385361876520264, -23.59649016807271593, 145.1750000027311387 ) ) ;
#42704=CARTESIAN_POINT ( 'NONE',  ( 3.071040654511329571, -27.74725471568222801, 139.9999999999999716 ) ) ;
#42750=ORIENTED_EDGE ( 'NONE', *, *, #106636, .T. ) ;
#42759=CARTESIAN_POINT ( 'NONE',  ( 27.73933785331498214, 9.013057229001095294, 140.4750000027311785 ) ) ;
#42860=VERTEX_POINT ( 'NONE', #75092 ) ;
#42863=EDGE_CURVE ( 'NONE', #103252, #144934, #84261, .T. ) ;
#42897=CARTESIAN_POINT ( 'NONE',  ( -21.82220748998223669, -8.288476145941629625, 169.3167957967150983 ) ) ;
#42987=B_SPLINE_CURVE_WITH_KNOTS ( 'NONE', 3,
 ( #97740, #18956, #143260, #157463, #113915, #156464, #112930, #175613, #67426, #17964 ),
 .UNSPECIFIED., .F., .F.,
 ( 4, 2, 2, 2, 4 ),
 ( 3.469446951953614189E-18, 0.0009160790699533124387, 0.001832158139906621408, 0.002748237209859930377, 0.003664316279813239347 ),
 .UNSPECIFIED. ) ;
#43046=CARTESIAN_POINT ( 'NONE',  ( 21.48948823426665911, -5.485118590273156514, 173.8226827327241608 ) ) ;
#43071=ORIENTED_EDGE ( 'NONE', *, *, #155738, .T. ) ;
#43100=CARTESIAN_POINT ( 'NONE',  ( -27.73933785331498925, -9.013057229001049109, 143.4750000027311785 ) ) ;
#43138=CARTESIAN_POINT ( 'NONE',  ( -24.44405923433090067, -13.71792739260092731, 165.9118100595187286 ) ) ;
#43155=EDGE_CURVE ( 'NONE', #131752, #56947, #14412, .T. ) ;
#43339=CARTESIAN_POINT ( 'NONE',  ( -21.93653645885848746, -8.192071713419743162, 172.2938920027118002 ) ) ;
#43344=CARTESIAN_POINT ( 'NONE',  ( -3.573655867282028392E-15, 2.428612866367529932E-14, 139.9999999999999716 ) ) ;
#43361=CARTESIAN_POINT ( 'NONE',  ( 24.39441179196515463, -8.562450407400064023, 166.7298547261019053 ) ) ;
#43383=ORIENTED_EDGE ( 'NONE', *, *, #190970, .T. ) ;
#43445=CARTESIAN_POINT ( 'NONE',  ( 22.44159573604009594, -16.30477369853687364, 145.6750000027311671 ) ) ;
#43490=CARTESIAN_POINT ( 'NONE',  ( -3.573655867282028392E-15, 2.428612866367529932E-14, 164.9999999999999716 ) ) ;
#43521=CIRCLE ( 'NONE', #11203, 25.62086810090349331 ) ;
#43608=CARTESIAN_POINT ( 'NONE',  ( -8.571926809382601320, -26.38167802310801591, 145.2750000027311899 ) ) ;
#43689=CARTESIAN_POINT ( 'NONE',  ( -17.17579732620334454, -22.53935769174907122, 140.0000000000000000 ) ) ;
#43733=CARTESIAN_POINT ( 'NONE',  ( 26.36463166569312477, 3.076743934663749069, 174.2851114983683942 ) ) ;
#43747=CARTESIAN_POINT ( 'NONE',  ( -28.82186960331499392, -9.364793116373526516, 142.0999999999999659 ) ) ;
#43770=CARTESIAN_POINT ( 'NONE',  ( -22.32889156691206622, 5.550768075871975071, 173.1969276168243823 ) ) ;
#43786=DIRECTION ( 'NONE',  ( 0.000000000000000000, 0.000000000000000000, -1.000000000000000000 ) ) ;
#43791=EDGE_LOOP ( 'NONE', ( #62971, #160380, #75656, #168823 ) ) ;
#43845=CARTESIAN_POINT ( 'NONE',  ( -21.75836449082842705, -8.509082329565398339, 169.1767350484829251 ) ) ;
#43885=CARTESIAN_POINT ( 'NONE',  ( -21.75500197730213259, -5.836128546636254910, 172.5265712840238734 ) ) ;
#44036=ORIENTED_EDGE ( 'NONE', *, *, #12998, .F. ) ;
#44040=CARTESIAN_POINT ( 'NONE',  ( 21.58577566615618082, -5.573877917343201815, 173.3856758005497056 ) ) ;
#44096=CARTESIAN_POINT ( 'NONE',  ( -22.44159573604009950, -16.30477369853688430, 141.5750000027311728 ) ) ;
#44100=CARTESIAN_POINT ( 'NONE',  ( 17.14385361876520264, 23.59649016807275856, 144.6750000027311671 ) ) ;
#44136=CARTESIAN_POINT ( 'NONE',  ( -20.93662873023658122, -11.00447265502299210, 170.1964094900432372 ) ) ;
#44284=CARTESIAN_POINT ( 'NONE',  ( 22.94331271462294097, -3.784814030245898575, 190.0000000000000000 ) ) ;
#44335=CARTESIAN_POINT ( 'NONE',  ( -21.64434376887846767, -9.890319055725230513, 170.6724019390509568 ) ) ;
#44357=CARTESIAN_POINT ( 'NONE',  ( 28.79475375365586132, 2.781246896534039337E-14, 146.9843446568999923 ) ) ;
#44440=CARTESIAN_POINT ( 'NONE',  ( 27.73933785331498214, 9.013057229001095294, 145.9750000027311785 ) ) ;
#44479=DIRECTION ( 'NONE',  ( -0.8437662581494470571, 0.5367108174878540972, 0.000000000000000000 ) ) ;
#44516=CARTESIAN_POINT ( 'NONE',  ( -5.427562675786936573E-15, 30.27659582821221207, 143.4843446568999639 ) ) ;
#44526=CARTESIAN_POINT ( 'NONE',  ( -26.70613957415103101, 7.662257527287501979, 167.2521143936661474 ) ) ;
#44528=DIRECTION ( 'NONE',  ( 0.000000000000000000, 0.000000000000000000, 1.000000000000000000 ) ) ;
#44601=CARTESIAN_POINT ( 'NONE',  ( 1.784210473542230573E-15, -29.16686587814331588, 141.3750000027311557 ) ) ;
#44603=DIRECTION ( 'NONE',  ( -1.000000000000000000, 0.000000000000000000, 0.000000000000000000 ) ) ;
#44681=CARTESIAN_POINT ( 'NONE',  ( 6.377275439838900439, -27.11046330701184459, 140.0000000000000000 ) ) ;
#44723=CARTESIAN_POINT ( 'NONE',  ( 26.79623349963134871, 5.044589688426436069, 170.2051123914324080 ) ) ;
#44737=CARTESIAN_POINT ( 'NONE',  ( -8.906447517083053711, -27.41122689804191026, 140.4000000000000057 ) ) ;
#44897=FACE_OUTER_BOUND ( 'NONE', #175080, .T. ) ;
#44920=CARTESIAN_POINT ( 'NONE',  ( -28.79475375365586842, 2.428612866367529932E-14, 150.0000000000000000 ) ) ;
#44930=DIRECTION ( 'NONE',  ( 0.000000000000000000, 0.000000000000000000, -1.000000000000000000 ) ) ;
#44992=VECTOR ( 'NONE', #175058, 1000.000000000000000 ) ;
#45086=CARTESIAN_POINT ( 'NONE',  ( -27.73933785331498925, 9.013057229001089965, 143.2750000027311899 ) ) ;
#45090=CARTESIAN_POINT ( 'NONE',  ( -5.359611314223446995E-15, 29.16686587814335496, 148.8750000027311842 ) ) ;
#45125=CARTESIAN_POINT ( 'NONE',  ( -24.06609220500524415, -14.38661408136937148, 165.8682408874374232 ) ) ;
#45277=CARTESIAN_POINT ( 'NONE',  ( 16.18341559714236055, 22.93862090151660382, 139.9999999999999716 ) ) ;
#45293=CARTESIAN_POINT ( 'NONE',  ( -28.79475375365586842, 2.428612866367529932E-14, 144.2656553485623760 ) ) ;
#45306=DIRECTION ( 'NONE',  ( 0.1039620511844979445, 0.1039620511844979445, -0.9891328443778539814 ) ) ;
#45341=EDGE_LOOP ( 'NONE', ( #152192, #180986, #168348, #117968, #16483 ) ) ;
#45366=CARTESIAN_POINT ( 'NONE',  ( 27.88129983271499768, 6.733757357597986548, 162.1517353552272880 ) ) ;
#45427=CARTESIAN_POINT ( 'NONE',  ( -27.73933785331498925, 9.013057229001089965, 144.7750000027311614 ) ) ;
#45432=ORIENTED_EDGE ( 'NONE', *, *, #125504, .T. ) ;
#45518=EDGE_CURVE ( 'NONE', #68306, #155416, #61071, .T. ) ;
#45589=CARTESIAN_POINT ( 'NONE',  ( -22.44159573604009950, -16.30477369853688430, 143.0750000027311728 ) ) ;
#45643=ADVANCED_FACE ( 'NONE', ( #121753 ), #55350, .T. ) ;
#45752=LINE ( 'NONE', #78058, #4847 ) ;
#45770=VERTEX_POINT ( 'NONE', #199605 ) ;
#45825=CARTESIAN_POINT ( 'NONE',  ( -21.95653654802831412, -6.613221094984323756, 171.0358100525039902 ) ) ;
#45862=CARTESIAN_POINT ( 'NONE',  ( -25.31005825231498818, -7.802036135343648482, 170.7258689498729325 ) ) ;
#45887=DIRECTION ( 'NONE',  ( 1.000000000000000000, 0.000000000000000000, -0.000000000000000000 ) ) ;
#46062=VERTEX_POINT ( 'NONE', #123724 ) ;
#46069=CARTESIAN_POINT ( 'NONE',  ( 8.571926809382603096, -26.38167802310801235, 143.9750000027312069 ) ) ;
#46073=CARTESIAN_POINT ( 'NONE',  ( -27.73933785331498925, 9.013057229001089965, 147.2750000027311614 ) ) ;
#46108=CARTESIAN_POINT ( 'NONE',  ( -25.27727188472087505, -10.29814791481089387, 170.4127952078933106 ) ) ;
#46263=CARTESIAN_POINT ( 'NONE',  ( -11.70006521384596709, 26.14342653898853541, 139.9999999999999716 ) ) ;
#46351=CARTESIAN_POINT ( 'NONE',  ( -24.79447686064998635, 6.332871904607505265, 168.1804317516294134 ) ) ;
#46384=VECTOR ( 'NONE', #120353, 1000.000000000000000 ) ;
#46416=CARTESIAN_POINT ( 'NONE',  ( 17.14385361876520264, -23.59649016807271238, 145.5750000027312012 ) ) ;
#46429=CARTESIAN_POINT ( 'NONE',  ( 27.94727395831375460, -6.976223361892288644, 161.4607800657734344 ) ) ;
#46582=CARTESIAN_POINT ( 'NONE',  ( 17.14385361876520264, -23.59649016807271238, 141.5750000027312012 ) ) ;
#46622=ORIENTED_EDGE ( 'NONE', *, *, #19336, .F. ) ;
#46664=CARTESIAN_POINT ( 'NONE',  ( -26.77313074627685907, 4.631999166354653141, 170.7390164845645870 ) ) ;
#46723=CARTESIAN_POINT ( 'NONE',  ( -28.82186960331499392, 9.364793116373565596, 141.9000000000000057 ) ) ;
#46734=CIRCLE ( 'NONE', #17581, 23.10356920737165254 ) ;
#46745=CARTESIAN_POINT ( 'NONE',  ( 21.92644707618960709, -9.078916001213698905, 171.2473621415418847 ) ) ;
#46821=CARTESIAN_POINT ( 'NONE',  ( -24.24393946302878078, -5.863316274098051117, 172.4343578713344982 ) ) ;
#46880=DIRECTION ( 'NONE',  ( 0.000000000000000000, -0.1045284632676537068, 0.9945218953682734009 ) ) ;
#46900=CARTESIAN_POINT ( 'NONE',  ( 1.988064558232696151E-15, -30.27659582821216588, 148.4843446568999923 ) ) ;
#46910=VECTOR ( 'NONE', #84540, 1000.000000000000000 ) ;
#46985=PLANE ( 'NONE',  #129321 ) ;
#47013=CARTESIAN_POINT ( 'NONE',  ( 21.96434091948367850, -6.687777057363585520, 170.9277123045938822 ) ) ;
#47025=FACE_OUTER_BOUND ( 'NONE', #152969, .T. ) ;
#47032=ADVANCED_FACE ( 'NONE', ( #84305 ), #8485, .T. ) ;
#47075=CARTESIAN_POINT ( 'NONE',  ( -27.73933785331498925, 9.013057229001089965, 143.2750000027311899 ) ) ;
#47103=EDGE_CURVE ( 'NONE', #100170, #16229, #26667, .T. ) ;
#47110=CARTESIAN_POINT ( 'NONE',  ( -21.04946095171256104, -10.86023174791543866, 170.2405914574444239 ) ) ;
#47218=DIRECTION ( 'NONE',  ( 0.000000000000000000, 0.000000000000000000, -1.000000000000000000 ) ) ;
#47334=CARTESIAN_POINT ( 'NONE',  ( 17.79613651744293534, 24.49428055684532524, 145.2843446568999752 ) ) ;
#47360=CARTESIAN_POINT ( 'NONE',  ( -24.24385185424182154, 7.025880200331685366, 170.5073520790474504 ) ) ;
#47423=CARTESIAN_POINT ( 'NONE',  ( 27.73933785331498569, 2.768321779492822058E-14, 145.8750000027311842 ) ) ;
#47460=CARTESIAN_POINT ( 'NONE',  ( -19.49401214000077331, 12.39993551617566858, 164.9999999999999716 ) ) ;
#47553=CARTESIAN_POINT ( 'NONE',  ( 28.79475375365563750, 9.355982642739540722, 149.0843446568999866 ) ) ;
#47565=( BOUNDED_CURVE ( )  B_SPLINE_CURVE ( 2, ( #88803, #150496, #153453, #123107, #14951, #11993, #73656, #152461, #90777, #107934, #45293 ),
 .UNSPECIFIED., .F., .T. ) 
 B_SPLINE_CURVE_WITH_KNOTS ( ( 3, 2, 2, 2, 2, 3 ),
 ( 0.3000000000000030420, 0.3200000000000030598, 0.3400000000000030775, 0.3600000000000030953, 0.3800000000000031131, 0.4000000000000031308 ),
 .UNSPECIFIED. ) 
 CURVE ( )  GEOMETRIC_REPRESENTATION_ITEM ( )  RATIONAL_B_SPLINE_CURVE ( ( 0.9999999999999925615, 0.9510565162951609697, 1.000000000000000000, 0.9510565162951535312, 1.000000000000000000, 0.9510565162951535312, 1.000000000000000000, 0.9510565162951535312, 1.000000000000000000, 0.9510565162951458706, 1.000000000000007550 ) ) 
 REPRESENTATION_ITEM ( '' )  );
#47566=ORIENTED_EDGE ( 'NONE', *, *, #19851, .T. ) ;
#47585=CARTESIAN_POINT ( 'NONE',  ( -27.74069374691375955, 6.311165852667651066, 163.4895129000220209 ) ) ;
#47631=DIRECTION ( 'NONE',  ( 0.000000000000000000, 0.000000000000000000, -1.000000000000000000 ) ) ;
#47724=CARTESIAN_POINT ( 'NONE',  ( -8.906447517083053711, -27.41122689804191026, 142.4000000000000057 ) ) ;
#47737=CARTESIAN_POINT ( 'NONE',  ( 26.62494319856317304, -7.396441074661128212, 168.1134502243652094 ) ) ;
#47743=CARTESIAN_POINT ( 'NONE',  ( 21.83922654085338877, -7.858455564366274793, 172.8813051029758299 ) ) ;
#47767=ORIENTED_EDGE ( 'NONE', *, *, #133168, .T. ) ;
#47785=CIRCLE ( 'NONE', #83263, 26.05799246640827960 ) ;
#47861=DIRECTION ( 'NONE',  ( 1.000000000000000000, 0.000000000000000000, 0.000000000000000000 ) ) ;
#47884=CARTESIAN_POINT ( 'NONE',  ( -3.573655867282028392E-15, -12.39993551617566503, 175.0000000000000000 ) ) ;
#48040=VERTEX_POINT ( 'NONE', #188060 ) ;
#48101=DIRECTION ( 'NONE',  ( 1.000000000000000000, 0.000000000000000000, 0.000000000000000000 ) ) ;
#48106=CARTESIAN_POINT ( 'NONE',  ( -21.47376810973161199, -7.452933495370250405, 174.2084625793504244 ) ) ;
#48174=EDGE_CURVE ( 'NONE', #51216, #51307, #48744, .T. ) ;
#48184=ORIENTED_EDGE ( 'NONE', *, *, #146255, .T. ) ;
#48246=ORIENTED_EDGE ( 'NONE', *, *, #69903, .T. ) ;
#48259=B_SPLINE_CURVE_WITH_KNOTS ( 'NONE', 3,
 ( #37011, #86520, #22857, #189722, #20848, #131020, #53180, #159352, #99682, #115865, #148204, #82506, #70361, #116855 ),
 .UNSPECIFIED., .F., .F.,
 ( 4, 2, 2, 2, 2, 2, 4 ),
 ( -0.0006136969902427243540, 0.0004464899733162487790, 0.001506676936875221912, 0.003627050863993200487, 0.004687237827552194654, 0.005747424791111188820, 0.007867798718229178020 ),
 .UNSPECIFIED. ) ;
#48354=CARTESIAN_POINT ( 'NONE',  ( -21.88033147701267822, 7.974798826780869376, 169.5716465351736133 ) ) ;
#48415=CARTESIAN_POINT ( 'NONE',  ( 21.81018892176227908, 9.477090470496801089, 170.9397748289983099 ) ) ;
#48420=CARTESIAN_POINT ( 'NONE',  ( 27.73933785331498569, 2.768321779492822058E-14, 141.8750000027311842 ) ) ;
#48457=CARTESIAN_POINT ( 'NONE',  ( 24.43795752428853518, 7.704305290315001997, 171.8420761435737631 ) ) ;
#48504=CARTESIAN_POINT ( 'NONE',  ( -27.73933785331498925, 2.428612866367529932E-14, 149.1250000027311842 ) ) ;
#48508=CARTESIAN_POINT ( 'NONE',  ( -24.02723517065431125, -14.44770145514793036, 165.8682408883346397 ) ) ;
#48705=ORIENTED_EDGE ( 'NONE', *, *, #2143, .F. ) ;
#48707=CARTESIAN_POINT ( 'NONE',  ( -21.70980307670620846, -7.452553642297963243, 174.2373330747589932 ) ) ;
#48729=CARTESIAN_POINT ( 'NONE',  ( 20.69372460268611746, -11.29034304323151794, 170.1224388339879567 ) ) ;
#48733=CARTESIAN_POINT ( 'NONE',  ( -5.427562675786936573E-15, 30.27659582821221207, 143.7656553485623476 ) ) ;
#48744=( BOUNDED_CURVE ( )  B_SPLINE_CURVE ( 2, ( #16214, #47553, #64702, #62693, #19201, #4005, #126364, #124375, #49530, #32377, #143509 ),
 .UNSPECIFIED., .F., .F. ) 
 B_SPLINE_CURVE_WITH_KNOTS ( ( 3, 2, 2, 2, 2, 3 ),
 ( 0.9000000000000007994, 0.9200000000000007061, 0.9400000000000003908, 0.9600000000000002975, 0.9800000000000002043, 1.000000000000000000 ),
 .UNSPECIFIED. ) 
 CURVE ( )  GEOMETRIC_REPRESENTATION_ITEM ( )  RATIONAL_B_SPLINE_CURVE ( ( 0.9999999999999981126, 0.9510565162951554186, 1.000000000000000000, 0.9510565162951535312, 1.000000000000000000, 0.9510565162951535312, 1.000000000000000000, 0.9510565162951535312, 1.000000000000000000, 0.9510565162951535312, 1.000000000000000000 ) ) 
 REPRESENTATION_ITEM ( '' )  );
#48811=CARTESIAN_POINT ( 'NONE',  ( 17.81289503416611453, -24.51734667627695785, 144.9500000054623854 ) ) ;
#49116=CARTESIAN_POINT ( 'NONE',  ( 1.988064558232696151E-15, -30.27659582821216588, 140.7656553485623760 ) ) ;
#49205=CARTESIAN_POINT ( 'NONE',  ( -3.573655867282028392E-15, 2.428612866367529932E-14, 139.9999999999999716 ) ) ;
#49250=CARTESIAN_POINT ( 'NONE',  ( 12.83293741674485133, 25.03729200590208848, 139.9999999999999716 ) ) ;
#49336=CARTESIAN_POINT ( 'NONE',  ( -24.57691432906752382, 7.727872488968269948, 167.2019946024466890 ) ) ;
#49397=CARTESIAN_POINT ( 'NONE',  ( 20.74379371951214424, 11.24248911466463774, 170.1280252572803420 ) ) ;
#49402=CARTESIAN_POINT ( 'NONE',  ( 17.14385361876520264, 23.59649016807275856, 142.1750000027311671 ) ) ;
#49486=VECTOR ( 'NONE', #123722, 1000.000000000000114 ) ;
#49530=CARTESIAN_POINT ( 'NONE',  ( -23.29544513554941076, 16.92513159979227666, 149.7843446568999752 ) ) ;
#49565=CARTESIAN_POINT ( 'NONE',  ( -27.32543223595603266, 4.845308524273425732, 167.4404622590849385 ) ) ;
#49618=VECTOR ( 'NONE', #43786, 1000.000000000000000 ) ;
#49632=CARTESIAN_POINT ( 'NONE',  ( 21.94381615377240280, 13.26253372808201902, 167.9278110240112767 ) ) ;
#49707=EDGE_CURVE ( 'NONE', #146141, #66087, #71433, .T. ) ;
#49715=CARTESIAN_POINT ( 'NONE',  ( 25.85392304583073297, -7.514126903509208866, 173.7688241862487644 ) ) ;
#49721=CARTESIAN_POINT ( 'NONE',  ( 20.51334883519569985, -11.49142661404781229, 170.0774692710818101 ) ) ;
#49743=ORIENTED_EDGE ( 'NONE', *, *, #148158, .T. ) ;
#49797=EDGE_CURVE ( 'NONE', #33758, #95658, #107578, .T. ) ;
#49812=CARTESIAN_POINT ( 'NONE',  ( -27.73933785331498925, 9.013057229001088189, 149.2750000027311614 ) ) ;
#49924=( BOUNDED_SURFACE ( )  B_SPLINE_SURFACE ( 3, 2, ( 
 ( #6753, #36099, #146268 ),
 ( #38111, #97751, #68432 ),
 ( #101773, #159439, #190793 ),
 ( #52267, #113925, #7754 ),
 ( #99766, #175625, #37099 ),
 ( #161451, #98758, #160451 ),
 ( #39106, #22942, #21942 ),
 ( #69438, #131106, #100762 ),
 ( #162444, #23945, #8776 ),
 ( #85599, #147286, #70445 ),
 ( #43845, #121660, #28694 ),
 ( #199513, #182369, #16482 ),
 ( #77148, #154986, #197535 ),
 ( #137831, #32643, #92311 ),
 ( #167197, #105511, #91299 ),
 ( #123634, #122655, #31651 ),
 ( #90330, #185330, #76151 ),
 ( #45825, #13501, #152015 ),
 ( #78131, #171156, #75166 ),
 ( #186340, #46821, #109471 ),
 ( #60980, #184343, #136838 ),
 ( #107476, #12530, #198522 ),
 ( #170158, #106493, #169154 ),
 ( #59993, #183355, #30658 ) ),
 .UNSPECIFIED., .F., .F., .T. ) 
 B_SPLINE_SURFACE_WITH_KNOTS ( ( 4, 2, 2, 2, 2, 2, 2, 2, 2, 2, 2, 4 ),
 ( 3, 3 ),
 ( 0.000000000000000000, 0.001899702839891690993, 0.002849554259837536706, 0.003799405679783381985, 0.005699108519675073412, 0.006648959939620918691, 0.007598811359566763970, 0.008548662779512609250, 0.009498514199458456264, 0.01139821703935014682, 0.01329791987924183738, 0.01519762271913352794 ),
 ( 0.000000000000000000, 1.000000000000000000 ),
 .UNSPECIFIED. ) 
 GEOMETRIC_REPRESENTATION_ITEM ( )  RATIONAL_B_SPLINE_SURFACE ( (
 ( 1.000000000000000000, 0.7660444431189795678, 1.000000000000000000),
 ( 1.000000000000000000, 0.7753720600382140171, 1.000000000000000000),
 ( 1.000000000000000000, 0.7832595754286290068, 1.000000000000000000),
 ( 1.000000000000000000, 0.7928595458705313126, 1.000000000000000000),
 ( 1.000000000000000000, 0.7956872332516286006, 1.000000000000000000),
 ( 1.000000000000000000, 0.8005750596157429344, 1.000000000000000000),
 ( 1.000000000000000000, 0.8026302056541707586, 1.000000000000000000),
 ( 1.000000000000000000, 0.8075080643848452366, 1.000000000000000000),
 ( 1.000000000000000000, 0.8091143015810108308, 1.000000000000000000),
 ( 1.000000000000000000, 0.8093067629632920701, 1.000000000000000000),
 ( 1.000000000000000000, 0.8089952915731790650, 1.000000000000000000),
 ( 1.000000000000000000, 0.8076919994862170604, 1.000000000000000000),
 ( 1.000000000000000000, 0.8067078407649250771, 1.000000000000000000),
 ( 1.000000000000000000, 0.8041786842467109064, 1.000000000000000000),
 ( 1.000000000000000000, 0.8026334674877432240, 1.000000000000000000),
 ( 1.000000000000000000, 0.7990747329468971261, 1.000000000000000000),
 ( 1.000000000000000000, 0.7970509760942148247, 1.000000000000000000),
 ( 1.000000000000000000, 0.7904793850862690263, 1.000000000000000000),
 ( 1.000000000000000000, 0.7855040224313801778, 1.000000000000000000),
 ( 1.000000000000000000, 0.7751942650507522847, 1.000000000000000000),
 ( 1.000000000000000000, 0.7698260778212435707, 1.000000000000000000),
 ( 1.000000000000000000, 0.7598259884960076871, 1.000000000000000000),
 ( 1.000000000000000000, 0.7551428682220966415, 1.000000000000000000),
 ( 1.000000000000000000, 0.7510191126010865581, 1.000000000000000000) ) ) 
 REPRESENTATION_ITEM ( '' )  SURFACE ( )  );
#50058=CARTESIAN_POINT ( 'NONE',  ( -22.03588254365376997, 7.477584490969214848, 173.9991804579021277 ) ) ;
#50092=CYLINDRICAL_SURFACE ( 'NONE', #19284, 26.79475375365586487 ) ;
#50170=ORIENTED_EDGE ( 'NONE', *, *, #5739, .T. ) ;
#50189=ORIENTED_EDGE ( 'NONE', *, *, #92009, .F. ) ;
#50236=EDGE_LOOP ( 'NONE', ( #27782, #81088 ) ) ;
#50252=CARTESIAN_POINT ( 'NONE',  ( 24.81492239413702805, 12.70475479534830043, 139.9999999999999716 ) ) ;
#50341=CARTESIAN_POINT ( 'NONE',  ( -24.81886791266634873, 6.075537473402705224, 168.3989613422507432 ) ) ;
#50406=CARTESIAN_POINT ( 'NONE',  ( -27.73933785331498925, 2.428612866367529932E-14, 140.8750000027311842 ) ) ;
#50526=CARTESIAN_POINT ( 'NONE',  ( 27.16945489364049848, -10.00000000000000000, 149.7909430734646890 ) ) ;
#50538=SURFACE_STYLE_FILL_AREA ( #97010 ) ;
#50560=AXIS2_PLACEMENT_3D ( 'NONE', #75878, #105236, #182088 ) ;
#50601=CARTESIAN_POINT ( 'NONE',  ( 21.62954880396029367, -5.465688001471229462, 174.0035134771793253 ) ) ;
#50629=CARTESIAN_POINT ( 'NONE',  ( 21.93180397000027781, 7.641141194973617878, 169.8616410530779604 ) ) ;
#50685=ADVANCED_FACE ( 'NONE', ( #174634 ), #49924, .F. ) ;
#50717=CARTESIAN_POINT ( 'NONE',  ( 26.70292545465252942, -6.820347898103277018, 168.5277281069534752 ) ) ;
#50733=DIRECTION ( 'NONE',  ( 0.000000000000000000, 0.000000000000000000, -1.000000000000000000 ) ) ;
#50795=CARTESIAN_POINT ( 'NONE',  ( -17.14385361876520619, 23.59649016807275856, 149.0750000027311728 ) ) ;
#50796=CARTESIAN_POINT ( 'NONE',  ( 1.993301997531345292E-15, -30.30510711980685912, 144.7500000054623399 ) ) ;
#50880=CARTESIAN_POINT ( 'NONE',  ( -3.573655867282028392E-15, 2.428612866367529932E-14, 155.0000000000000000 ) ) ;
#50959=CARTESIAN_POINT ( 'NONE',  ( 1.988064558232696151E-15, -30.27659582821216588, 144.4843446568999639 ) ) ;
#51076=DIRECTION ( 'NONE',  ( -1.000000000000000000, 0.000000000000000000, 0.000000000000000000 ) ) ;
#51216=VERTEX_POINT ( 'NONE', #64959 ) ;
#51269=ADVANCED_FACE ( 'NONE', ( #79130 ), #84743, .T. ) ;
#51307=VERTEX_POINT ( 'NONE', #127384 ) ;
#51319=EDGE_CURVE ( 'NONE', #16229, #25364, #52071, .T. ) ;
#51382=CARTESIAN_POINT ( 'NONE',  ( 21.76075944043963872, 9.615265036675765487, 170.8440536485302346 ) ) ;
#51392=ORIENTED_EDGE ( 'NONE', *, *, #159956, .F. ) ;
#51400=CARTESIAN_POINT ( 'NONE',  ( 27.07812102864233239, -7.738729533396120353, 165.1046384229466355 ) ) ;
#51494=ORIENTED_EDGE ( 'NONE', *, *, #171107, .F. ) ;
#51520=SURFACE_SIDE_STYLE ('',( #50538 ) ) ;
#51553=CARTESIAN_POINT ( 'NONE',  ( -3.573655867282028392E-15, 2.428612866367529932E-14, 169.9999999999999716 ) ) ;
#51560=CARTESIAN_POINT ( 'NONE',  ( 28.79475375365586132, 2.781246896534039337E-14, 141.2656553485623760 ) ) ;
#51675=ORIENTED_EDGE ( 'NONE', *, *, #79934, .T. ) ;
#51678=CARTESIAN_POINT ( 'NONE',  ( -25.31021317688466254, 7.802057701675677137, 170.7256852586636171 ) ) ;
#51709=CARTESIAN_POINT ( 'NONE',  ( 21.38418241377623019, -7.427326039334300134, 174.4773576836617224 ) ) ;
#51722=CARTESIAN_POINT ( 'NONE',  ( 22.44159573604009239, 16.30477369853692693, 142.0750000027311728 ) ) ;
#51740=AXIS2_PLACEMENT_3D ( 'NONE', #54953, #99447, #5436 ) ;
#51768=AXIS2_PLACEMENT_3D ( 'NONE', #50526, #173876, #35346 ) ;
#51777=CARTESIAN_POINT ( 'NONE',  ( -17.14385361876520264, -23.59649016807271593, 141.6750000027311103 ) ) ;
#51778=CARTESIAN_POINT ( 'NONE',  ( 23.31738231874054534, 16.94106989632529192, 145.4500000054623854 ) ) ;
#51950=CARTESIAN_POINT ( 'NONE',  ( 23.29544513554940011, 16.92513159979228021, 145.4656553485623647 ) ) ;
#51963=UNCERTAINTY_MEASURE_WITH_UNIT (LENGTH_MEASURE( 1.000000000000000082E-05 ), #93038, 'distance_accuracy_value', 'NONE');
#52071=B_SPLINE_CURVE_WITH_KNOTS ( 'NONE', 3,
 ( #143545, #47585, #3058, #5031, #49565, #4040, #124410, #78892 ),
 .UNSPECIFIED., .F., .F.,
 ( 4, 2, 2, 4 ),
 ( 0.01263483034531157588, 0.01686471550494908489, 0.01897965808476779689, 0.02109460066458651237 ),
 .UNSPECIFIED. ) ;
#52210=CARTESIAN_POINT ( 'NONE',  ( -8.898068258721474777, 27.38543819252877043, 147.5843446568999866 ) ) ;
#52221=CARTESIAN_POINT ( 'NONE',  ( 27.94130797166919322, 7.397772140654549133, 160.8977822374800155 ) ) ;
#52267=CARTESIAN_POINT ( 'NONE',  ( -20.56371838171433097, -11.04494471775294961, 168.1294998094270454 ) ) ;
#52306=CARTESIAN_POINT ( 'NONE',  ( 22.37486833544087617, -13.37560805684410070, 165.5209445320981558 ) ) ;
#52371=CARTESIAN_POINT ( 'NONE',  ( 21.38418241377623019, 7.427326039334300134, 174.4773576836617224 ) ) ;
#52411=CARTESIAN_POINT ( 'NONE',  ( 28.79475375365586132, 2.781246896534039337E-14, 147.2656553485624045 ) ) ;
#52484=CARTESIAN_POINT ( 'NONE',  ( 21.38418241377623019, 5.438282248597753110, 174.2683007571264113 ) ) ;
#52516=ORIENTED_EDGE ( 'NONE', *, *, #134775, .F. ) ;
#52575=CARTESIAN_POINT ( 'NONE',  ( 21.98831087263036110, -5.509728484239349022, 173.5901369092267430 ) ) ;
#52761=ADVANCED_FACE ( 'NONE', ( #163738 ), #25238, .F. ) ;
#52768=CARTESIAN_POINT ( 'NONE',  ( 8.571926809382597767, 26.38167802310806209, 140.7750000027311899 ) ) ;
#52782=CARTESIAN_POINT ( 'NONE',  ( 17.14385361876520264, 23.59649016807275856, 140.6750000027311387 ) ) ;
#52853=CARTESIAN_POINT ( 'NONE',  ( -24.44405923433097172, 13.71792739260091132, 165.9118100595185297 ) ) ;
#52895=CARTESIAN_POINT ( 'NONE',  ( 26.38458505201398907, 8.641005086744664609, 167.3773361139123494 ) ) ;
#52924=CIRCLE ( 'NONE', #101280, 27.91311885011353766 ) ;
#52948=VECTOR ( 'NONE', #131830, 1000.000000000000114 ) ;
#53139=CARTESIAN_POINT ( 'NONE',  ( -21.98685479826779954, 13.98560643873834408, 165.5209445330007441 ) ) ;
#53180=CARTESIAN_POINT ( 'NONE',  ( 25.78958964901895712, -10.70071173758533334, 166.5174151181484774 ) ) ;
#53216=CARTESIAN_POINT ( 'NONE',  ( 26.58496454516999563, 7.626754437231445749, 167.9682100371138915 ) ) ;
#53245=CARTESIAN_POINT ( 'NONE',  ( -24.60782464877076237, -7.576768089025921249, 167.2921030401324174 ) ) ;
#53255=FACE_OUTER_BOUND ( 'NONE', #148930, .T. ) ;
#53260=CARTESIAN_POINT ( 'NONE',  ( -28.75808110634262604, -1.452795517301058048, 139.9999999999999716 ) ) ;
#53303=CARTESIAN_POINT ( 'NONE',  ( 21.36928693577338123, -5.431965077040403322, 174.3311293403526179 ) ) ;
#53356=VECTOR ( 'NONE', #115141, 1000.000000000000000 ) ;
#53388=CARTESIAN_POINT ( 'NONE',  ( 26.82864639204112933, -7.693045595922322732, 166.5361468217299148 ) ) ;
#53497=CARTESIAN_POINT ( 'NONE',  ( 27.12243378312293274, 3.972435522077283121, 169.3718635229823235 ) ) ;
#53546=CARTESIAN_POINT ( 'NONE',  ( -3.573655867282028392E-15, 2.428612866367529932E-14, 155.0000000000000000 ) ) ;
#53553=LINE ( 'NONE', #9066, #124170 ) ;
#53612=CARTESIAN_POINT ( 'NONE',  ( 21.95653654802720212, 6.613221094984321091, 171.0358100525039902 ) ) ;
#53626=AXIS2_PLACEMENT_3D ( 'NONE', #93587, #3562, #48101 ) ;
#53724=CARTESIAN_POINT ( 'NONE',  ( -24.77450267193474076, -6.022707119490098293, 168.7078695393447560 ) ) ;
#53783=CARTESIAN_POINT ( 'NONE',  ( -5.429308488886486681E-15, 30.30510711980690175, 141.7500000054623683 ) ) ;
#53797=CARTESIAN_POINT ( 'NONE',  ( 17.14385361876520264, 23.59649016807275856, 142.6750000027311103 ) ) ;
#53819=AXIS2_PLACEMENT_3D ( 'NONE', #114699, #37867, #110716 ) ;
#53871=CARTESIAN_POINT ( 'NONE',  ( -20.93662873023604831, 11.00447265502299388, 170.1964094900432372 ) ) ;
#53913=CARTESIAN_POINT ( 'NONE',  ( 21.84611564451295962, 9.363109600221495299, 171.0247306346272751 ) ) ;
#53951=CARTESIAN_POINT ( 'NONE',  ( 23.29544513554940366, -16.92513159979222337, 144.7843446568999752 ) ) ;
#54040=CARTESIAN_POINT ( 'NONE',  ( -23.88380138457670654, 7.642903512909264840, 172.4262750319490181 ) ) ;
#54091=CARTESIAN_POINT ( 'NONE',  ( -23.29544513554940721, -16.92513159979223758, 140.4656553485623931 ) ) ;
#54252=CIRCLE ( 'NONE', #147795, 30.82560697742735556 ) ;
#54256=CARTESIAN_POINT ( 'NONE',  ( -24.39441179196517240, 8.562450407400056918, 166.7298547261019621 ) ) ;
#54313=CARTESIAN_POINT ( 'NONE',  ( 21.84611564451239119, -8.148379233839406766, 169.4346228884785148 ) ) ;
#54449=CARTESIAN_POINT ( 'NONE',  ( -23.49396498682886403, -16.15366880693413520, 140.0000000000000568 ) ) ;
#54721=CARTESIAN_POINT ( 'NONE',  ( 8.571926809382597767, 26.38167802310806209, 140.2750000027311899 ) ) ;
#54779=CARTESIAN_POINT ( 'NONE',  ( 27.73933785331498925, -9.013057229001033122, 142.2750000027311899 ) ) ;
#54780=CARTESIAN_POINT ( 'NONE',  ( -23.31738231874055600, 16.94106989632528837, 140.0500000054623513 ) ) ;
#54793=CARTESIAN_POINT ( 'NONE',  ( -17.14385361876520264, -23.59649016807271238, 141.6750000027311387 ) ) ;
#54818=ORIENTED_EDGE ( 'NONE', *, *, #159341, .F. ) ;
#54825=FACE_OUTER_BOUND ( 'NONE', #133870, .T. ) ;
#54865=CARTESIAN_POINT ( 'NONE',  ( -19.83801684532418363, 12.12952959760495908, 169.9999999999999716 ) ) ;
#54908=CARTESIAN_POINT ( 'NONE',  ( 23.64729612845681928, 13.72274676820423167, 169.8070494178799663 ) ) ;
#54920=CARTESIAN_POINT ( 'NONE',  ( 28.82186960331498327, 9.364793116373570925, 149.0999999999999943 ) ) ;
#54953=CARTESIAN_POINT ( 'NONE',  ( -3.573655867282028392E-15, 2.428612866367529932E-14, 167.9999999999999716 ) ) ;
#55006=CARTESIAN_POINT ( 'NONE',  ( -19.30190589895974185, 21.36759865781276346, 139.9999999999999716 ) ) ;
#55076=CARTESIAN_POINT ( 'NONE',  ( 27.73933785331498569, 2.768321779492822058E-14, 145.8750000027311842 ) ) ;
#55086=CARTESIAN_POINT ( 'NONE',  ( 23.64874990377914799, 15.04272038711346049, 165.8682408883346397 ) ) ;
#55305=CARTESIAN_POINT ( 'NONE',  ( 24.68411608548642988, -7.148172978124902599, 167.5704058020752996 ) ) ;
#55350=CYLINDRICAL_SURFACE ( 'NONE', #149824, 28.79475375365586487 ) ;
#55387=CARTESIAN_POINT ( 'NONE',  ( 27.40223502306392689, -7.751740014893113262, 163.3164180876353555 ) ) ;
#55596=CARTESIAN_POINT ( 'NONE',  ( -27.89963664982370872, -6.788868650209762379, 161.9772721943246552 ) ) ;
#55701=CARTESIAN_POINT ( 'NONE',  ( -8.898068258721474777, 27.38543819252877043, 141.5843446569000150 ) ) ;
#55723=CARTESIAN_POINT ( 'NONE',  ( 22.44159573604009594, -16.30477369853687364, 141.6750000027311671 ) ) ;
#55758=ORIENTED_EDGE ( 'NONE', *, *, #9833, .F. ) ;
#55778=CARTESIAN_POINT ( 'NONE',  ( -17.14385361876520264, -23.59649016807271593, 139.6750000027311955 ) ) ;
#55780=CARTESIAN_POINT ( 'NONE',  ( -23.31738231874055245, -16.94106989632524574, 140.4500000054623854 ) ) ;
#55785=EDGE_CURVE ( 'NONE', #148762, #101739, #39900, .T. ) ;
#55794=CARTESIAN_POINT ( 'NONE',  ( 8.571926809382603096, -26.38167802310801235, 143.9750000027312069 ) ) ;
#55849=CARTESIAN_POINT ( 'NONE',  ( -25.77159179889071439, -6.124174026812453597, 163.0907220140216509 ) ) ;
#55863=CARTESIAN_POINT ( 'NONE',  ( -26.57611637973580443, 7.696099174151423306, 167.9177021574031983 ) ) ;
#55906=CARTESIAN_POINT ( 'NONE',  ( 21.93180397000027781, 9.000796715316637275, 171.3297436093417900 ) ) ;
#55916=CARTESIAN_POINT ( 'NONE',  ( 28.82186960331498327, 2.781578969918950771E-14, 149.0000000000000000 ) ) ;
#55965=ORIENTED_EDGE ( 'NONE', *, *, #131623, .T. ) ;
#56055=CARTESIAN_POINT ( 'NONE',  ( -21.36928693577339544, 5.431965077040405099, 174.3311293403526179 ) ) ;
#56060=CARTESIAN_POINT ( 'NONE',  ( -21.82787714368444654, -6.011549001344956622, 172.1028946673681332 ) ) ;
#56074=CARTESIAN_POINT ( 'NONE',  ( 22.44159573604009594, -16.30477369853687364, 145.6750000027311671 ) ) ;
#56085=CARTESIAN_POINT ( 'NONE',  ( 25.28179187713399401, 11.97099003546684060, 166.1915553108511290 ) ) ;
#56185=B_SPLINE_CURVE_WITH_KNOTS ( 'NONE', 3,
 ( #171048, #33529, #81985, #186237, #32538, #124540, #175032, #93196, #94191, #48707, #154881, #78026 ),
 .UNSPECIFIED., .F., .F.,
 ( 4, 2, 2, 2, 2, 4 ),
 ( 0.003927129849554285117, 0.005134622258946382710, 0.006342114668338479436, 0.007549607077730577029, 0.008153353282426625825, 0.008757099487122674622 ),
 .UNSPECIFIED. ) ;
#56265=CARTESIAN_POINT ( 'NONE',  ( -8.571926809382608425, 26.38167802310805854, 148.9750000027311785 ) ) ;
#56286=ORIENTED_EDGE ( 'NONE', *, *, #175528, .T. ) ;
#56308=CARTESIAN_POINT ( 'NONE',  ( 24.72709851008550075, -6.869189314501102039, 167.7661538690260556 ) ) ;
#56351=CARTESIAN_POINT ( 'NONE',  ( 26.56065628307859683, -9.391201389438098346, 155.7923318601102380 ) ) ;
#56380=AXIS2_PLACEMENT_3D ( 'NONE', #15125, #185976, #32287 ) ;
#56405=VECTOR ( 'NONE', #106184, 1000.000000000000000 ) ;
#56415=CARTESIAN_POINT ( 'NONE',  ( 21.48956683882227381, 5.485153550827154945, 173.8223501052718518 ) ) ;
#56521=DIRECTION ( 'NONE',  ( 0.000000000000000000, 0.000000000000000000, -1.000000000000000000 ) ) ;
#56530=EDGE_LOOP ( 'NONE', ( #59185, #125324, #91803, #94426, #33772, #86117, #178384, #9953, #145915, #191657, #136965, #73626 ) ) ;
#56603=CARTESIAN_POINT ( 'NONE',  ( -23.29544513554940721, -16.92513159979223403, 142.1843446569000093 ) ) ;
#56622=CARTESIAN_POINT ( 'NONE',  ( 23.97133246043717847, 5.390759101651051211, 174.7603932261090733 ) ) ;
#56696=AXIS2_PLACEMENT_3D ( 'NONE', #166900, #196262, #180097 ) ;
#56704=EDGE_LOOP ( 'NONE', ( #27445, #59215 ) ) ;
#56712=VECTOR ( 'NONE', #186081, 1000.000000000000114 ) ;
#56716=CARTESIAN_POINT ( 'NONE',  ( -27.67867608143706804, 7.698234437107397632, 161.8893175680488525 ) ) ;
#56794=CARTESIAN_POINT ( 'NONE',  ( 22.44159573604009594, -16.30477369853687364, 147.6750000027311671 ) ) ;
#56806=CARTESIAN_POINT ( 'NONE',  ( -22.44159573604009950, -16.30477369853688430, 141.5750000027311728 ) ) ;
#56875=CARTESIAN_POINT ( 'NONE',  ( -25.66129429279789065, 9.008087060820807679, 171.3163768196993715 ) ) ;
#56917=CARTESIAN_POINT ( 'NONE',  ( 21.47376810973061723, 7.452933495370294814, 174.2084625793499981 ) ) ;
#56931=CARTESIAN_POINT ( 'NONE',  ( -5.359611314223446995E-15, 29.16686587814335496, 140.8750000027311842 ) ) ;
#56947=VERTEX_POINT ( 'NONE', #44284 ) ;
#56955=CARTESIAN_POINT ( 'NONE',  ( -21.87067081123533541, 5.494950430485542547, 173.7269556299028750 ) ) ;
#57015=CARTESIAN_POINT ( 'NONE',  ( 27.12243378312305708, -3.972435522077897296, 169.3718635229811014 ) ) ;
#57087=CARTESIAN_POINT ( 'NONE',  ( -22.44159573604010305, 16.30477369853692338, 148.6750000027311671 ) ) ;
#57320=CARTESIAN_POINT ( 'NONE',  ( 23.46037622755923380, -10.21219847193883368, 168.3031241911537847 ) ) ;
#57426=CARTESIAN_POINT ( 'NONE',  ( 20.48593134815244099, 11.15862823513540647, 168.1084560298344570 ) ) ;
#57450=CIRCLE ( 'NONE', #121938, 28.79475375365586487 ) ;
#57524=CARTESIAN_POINT ( 'NONE',  ( -21.96985492114659166, -8.492568044003455441, 171.8755390570805730 ) ) ;
#57626=EDGE_CURVE ( 'NONE', #15498, #140232, #35467, .T. ) ;
#57688=ORIENTED_EDGE ( 'NONE', *, *, #196970, .T. ) ;
#57717=DIRECTION ( 'NONE',  ( 0.1039620511844979306, -0.1039620511844979306, -0.9891328443778538704 ) ) ;
#57791=CARTESIAN_POINT ( 'NONE',  ( 23.31738231874054534, 16.94106989632529192, 139.4500000054623570 ) ) ;
#57861=EDGE_CURVE ( 'NONE', #104760, #66087, #191734, .T. ) ;
#57873=CARTESIAN_POINT ( 'NONE',  ( -26.68407921138448557, 3.932373394472265193, 171.8653659962753295 ) ) ;
#57928=CARTESIAN_POINT ( 'NONE',  ( 1.993301997531345292E-15, -30.30510711980685912, 148.5000000000000000 ) ) ;
#57943=CARTESIAN_POINT ( 'NONE',  ( 23.03403192006591027, -14.65170476119024912, 169.9999999999999716 ) ) ;
#58061=CARTESIAN_POINT ( 'NONE',  ( -23.97133246043719268, 5.390759101651052099, 174.7603932261090733 ) ) ;
#58066=DIRECTION ( 'NONE',  ( 0.1039620511844979306, 0.1039620511844979306, 0.9891328443778538704 ) ) ;
#58162=VECTOR ( 'NONE', #83809, 1000.000000000000000 ) ;
#58273=DIRECTION ( 'NONE',  ( 0.000000000000000000, 0.000000000000000000, 1.000000000000000000 ) ) ;
#58299=EDGE_CURVE ( 'NONE', #139693, #107790, #134342, .T. ) ;
#58495=CYLINDRICAL_SURFACE ( 'NONE', #154032, 28.79475375365586487 ) ;
#58503=CARTESIAN_POINT ( 'NONE',  ( -20.74379371951212647, -11.24248911466463596, 170.1280252572803988 ) ) ;
#58526=CARTESIAN_POINT ( 'NONE',  ( 24.66673051387559568, -7.254129419879413732, 167.4978569920363043 ) ) ;
#58582=FACE_OUTER_BOUND ( 'NONE', #27503, .T. ) ;
#58605=CARTESIAN_POINT ( 'NONE',  ( -5.359611314223446995E-15, 29.16686587814335496, 144.3750000027311842 ) ) ;
#58687=CARTESIAN_POINT ( 'NONE',  ( -17.79613651744294600, 24.49428055684532524, 141.6843446568999809 ) ) ;
#58689=CARTESIAN_POINT ( 'NONE',  ( -26.82864639204112578, 7.693045595922302304, 166.5361468217300569 ) ) ;
#58762=CARTESIAN_POINT ( 'NONE',  ( -8.571926809382601320, -26.38167802310801591, 147.2750000027311899 ) ) ;
#58832=CARTESIAN_POINT ( 'NONE',  ( -25.25560589046783733, -4.310829775027113620, 167.9999999999999716 ) ) ;
#58846=CARTESIAN_POINT ( 'NONE',  ( 0.2665833460779011288, -27.95491218073336270, 139.9999999999999716 ) ) ;
#58889=CARTESIAN_POINT ( 'NONE',  ( 21.95653654802720212, 8.266568072468359674, 172.1684357517875412 ) ) ;
#58902=CARTESIAN_POINT ( 'NONE',  ( -28.82186960331499392, 9.364793116373565596, 149.9000000000000057 ) ) ;
#58927=CARTESIAN_POINT ( 'NONE',  ( -21.62954880396024748, 5.465688001471193047, 174.0035134771795526 ) ) ;
#59129=ORIENTED_EDGE ( 'NONE', *, *, #57861, .T. ) ;
#59158=B_SPLINE_CURVE_WITH_KNOTS ( 'NONE', 3,
 ( #156602, #108088, #110090, #17092 ),
 .UNSPECIFIED., .F., .F.,
 ( 4, 4 ),
 ( 0.000000000000000000, 0.007966001190080937433 ),
 .UNSPECIFIED. ) ;
#59185=ORIENTED_EDGE ( 'NONE', *, *, #7692, .F. ) ;
#59210=EDGE_CURVE ( 'NONE', #79565, #189536, #157069, .T. ) ;
#59215=ORIENTED_EDGE ( 'NONE', *, *, #183623, .F. ) ;
#59243=CARTESIAN_POINT ( 'NONE',  ( 27.73933785331498214, 9.013057229001095294, 142.4750000027311785 ) ) ;
#59247=CARTESIAN_POINT ( 'NONE',  ( 1.784210473542230573E-15, -29.16686587814331588, 145.8750000027311273 ) ) ;
#59283=B_SPLINE_CURVE_WITH_KNOTS ( 'NONE', 3,
 ( #155025, #198563, #45862, #1326, #63006, #14530, #16521, #169191, #17511, #108519 ),
 .UNSPECIFIED., .F., .F.,
 ( 4, 2, 2, 2, 4 ),
 ( 3.469446951953613804E-18, 0.0009160790699533039819, 0.001832158139906604494, 0.002748237209859905224, 0.003664316279813205519 ),
 .UNSPECIFIED. ) ;
#59284=CARTESIAN_POINT ( 'NONE',  ( -25.55222625260941172, -11.31436996698886155, 166.3494238031455268 ) ) ;
#59345=ADVANCED_FACE ( 'NONE', ( #47025 ), #108683, .F. ) ;
#59421=CARTESIAN_POINT ( 'NONE',  ( -21.82762259161260232, 6.010869995788715059, 172.1044450858202026 ) ) ;
#59439=CARTESIAN_POINT ( 'NONE',  ( 26.53317239408746175, -7.611579847057702075, 168.2742808015845526 ) ) ;
#59522=CARTESIAN_POINT ( 'NONE',  ( 24.93942350307308686, 7.769968609432599926, 171.2173313942149946 ) ) ;
#59575=EDGE_CURVE ( 'NONE', #93307, #75663, #39803, .T. ) ;
#59589=CARTESIAN_POINT ( 'NONE',  ( -27.73933785331498925, 9.013057229001089965, 146.7750000027312183 ) ) ;
#59668=CARTESIAN_POINT ( 'NONE',  ( -23.29544513554941076, 16.92513159979227666, 143.7843446568999752 ) ) ;
#59678=CARTESIAN_POINT ( 'NONE',  ( -27.83964505791037425, 7.578386611925740368, 161.1890226338711614 ) ) ;
#59757=CARTESIAN_POINT ( 'NONE',  ( 17.14385361876520264, -23.59649016807271238, 143.5750000027312012 ) ) ;
#59789=CARTESIAN_POINT ( 'NONE',  ( 25.77159179889068596, 6.124174026812450045, 163.0907220140217930 ) ) ;
#59836=CARTESIAN_POINT ( 'NONE',  ( -21.73861122199408058, 7.688394669363296963, 173.2969830217476499 ) ) ;
#59894=CARTESIAN_POINT ( 'NONE',  ( 28.82186960331498327, 2.781578969918950771E-14, 143.0000000000000000 ) ) ;
#59909=CARTESIAN_POINT ( 'NONE',  ( -17.79613651744294600, 24.49428055684532524, 143.9656553485623647 ) ) ;
#59971=ORIENTED_EDGE ( 'NONE', *, *, #79934, .F. ) ;
#59993=CARTESIAN_POINT ( 'NONE',  ( -21.36928693577339189, -5.431965077040402434, 174.3311293403526179 ) ) ;
#60183=DIRECTION ( 'NONE',  ( 0.1039620511844979306, -0.1039620511844979306, 0.9891328443778538704 ) ) ;
#60191=DIRECTION ( 'NONE',  ( 0.000000000000000000, 0.000000000000000000, 1.000000000000000000 ) ) ;
#60238=CARTESIAN_POINT ( 'NONE',  ( -8.571926809382601320, -26.38167802310801591, 143.7750000027311899 ) ) ;
#60242=CARTESIAN_POINT ( 'NONE',  ( -5.359611314223446995E-15, 29.16686587814335496, 142.8750000027311842 ) ) ;
#60274=CARTESIAN_POINT ( 'NONE',  ( -28.79475375365586842, 2.428612866367529932E-14, 155.0000000000000000 ) ) ;
#60277=CARTESIAN_POINT ( 'NONE',  ( -25.11239783071220799, -12.35465959875006092, 166.1131185557732124 ) ) ;
#60415=CARTESIAN_POINT ( 'NONE',  ( -21.94595931813859124, 7.591279830614301893, 169.8931963588657368 ) ) ;
#60488=CARTESIAN_POINT ( 'NONE',  ( -23.29544513554941076, 16.92513159979227666, 145.7843446568999752 ) ) ;
#60576=CARTESIAN_POINT ( 'NONE',  ( 1.784210473542230573E-15, -29.16686587814331588, 143.3750000027311557 ) ) ;
#60743=CARTESIAN_POINT ( 'NONE',  ( -27.73933785331498925, 2.428612866367529932E-14, 144.8750000027311842 ) ) ;
#60756=FACE_OUTER_BOUND ( 'NONE', #17600, .T. ) ;
#60823=CARTESIAN_POINT ( 'NONE',  ( -25.86526910843991800, 7.630673861713272998, 173.3900163844835163 ) ) ;
#60864=CARTESIAN_POINT ( 'NONE',  ( 21.81230582904511550, 7.807068725604178638, 172.9985625539982550 ) ) ;
#60980=CARTESIAN_POINT ( 'NONE',  ( -21.73861122199297924, -5.803778330637474170, 172.6157762304496828 ) ) ;
#60981=VERTEX_POINT ( 'NONE', #64921 ) ;
#61071=LINE ( 'NONE', #154086, #10990 ) ;
#61109=ORIENTED_EDGE ( 'NONE', *, *, #4039, .T. ) ;
#61146=CARTESIAN_POINT ( 'NONE',  ( 14.68807091101007067, -23.54891160506147330, 139.9999999999999716 ) ) ;
#61228=CARTESIAN_POINT ( 'NONE',  ( 22.44159573604009594, -16.30477369853687364, 142.1750000027311671 ) ) ;
#61232=CARTESIAN_POINT ( 'NONE',  ( -22.44159573604009950, -16.30477369853688430, 147.5750000027312012 ) ) ;
#61269=CARTESIAN_POINT ( 'NONE',  ( -25.52568752982044842, -9.519068727187397272, 170.8917780290337873 ) ) ;
#61408=CARTESIAN_POINT ( 'NONE',  ( -19.49401214000074489, -12.39993551617566503, 167.9999999999999716 ) ) ;
#61470=CARTESIAN_POINT ( 'NONE',  ( -21.59135963187072704, 7.527667041516030721, 173.8290201207856285 ) ) ;
#61511=CARTESIAN_POINT ( 'NONE',  ( -23.84827716990724866, 9.022217638662548111, 168.8513102586128412 ) ) ;
#61571=CARTESIAN_POINT ( 'NONE',  ( 8.571926809382597767, 26.38167802310806209, 146.2750000027311899 ) ) ;
#61621=VERTEX_POINT ( 'NONE', #195273 ) ;
#61646=CARTESIAN_POINT ( 'NONE',  ( -28.79475375365596435, 9.355982642739093080, 143.8843446568999980 ) ) ;
#61659=CARTESIAN_POINT ( 'NONE',  ( -26.53515902489024825, -7.921333329385879196, 167.7790254135048826 ) ) ;
#61733=CARTESIAN_POINT ( 'NONE',  ( -5.359611314223446995E-15, 29.16686587814335496, 144.3750000027311842 ) ) ;
#61766=CARTESIAN_POINT ( 'NONE',  ( -28.32625367550113182, -10.00081768005069449, 140.0928639110588279 ) ) ;
#61869=CARTESIAN_POINT ( 'NONE',  ( -8.906447517083060816, 27.41122689804195645, 143.5999999999999943 ) ) ;
#61891=CARTESIAN_POINT ( 'NONE',  ( -24.62642639703178205, 5.957135776930584825, 169.3344962860537635 ) ) ;
#61893=DIRECTION ( 'NONE',  ( 1.000000000000000000, -0.000000000000000000, -0.000000000000000000 ) ) ;
#61909=EDGE_CURVE ( 'NONE', #11205, #31087, #34392, .T. ) ;
#61925=EDGE_CURVE ( 'NONE', #42860, #112207, #189407, .T. ) ;
#62031=B_SPLINE_CURVE_WITH_KNOTS ( 'NONE', 3,
 ( #107667, #12716, #169344, #167387, #181568, #15679, #196747, #16670, #197722, #486, #119883, #77340, #185521, #74382, #27898, #47013, #170350, #28883, #108672, #44040, #43046, #105700 ),
 .UNSPECIFIED., .F., .F.,
 ( 4, 2, 2, 2, 2, 2, 2, 2, 2, 2, 4 ),
 ( 0.000000000000000000, 0.001361773908209224556, 0.002042660862313843990, 0.002723547816418463857, 0.004085321724627701857, 0.004766208678732323893, 0.005447095632836944194, 0.006808869541046241175, 0.008170643449255537288, 0.009532417357464836871, 0.01089419126567413298 ),
 .UNSPECIFIED. ) ;
#62156=VERTEX_POINT ( 'NONE', #136563 ) ;
#62159=CARTESIAN_POINT ( 'NONE',  ( -3.573655867282028392E-15, -12.39993551617566503, 167.9999999999999716 ) ) ;
#62215=CARTESIAN_POINT ( 'NONE',  ( 8.571926809382603096, -26.38167802310801235, 145.9750000027311785 ) ) ;
#62219=CARTESIAN_POINT ( 'NONE',  ( -27.73933785331498925, -9.013057229001049109, 143.4750000027311785 ) ) ;
#62252=CARTESIAN_POINT ( 'NONE',  ( -26.62494319856254066, -7.396441074666470605, 168.1134502243608893 ) ) ;
#62409=CARTESIAN_POINT ( 'NONE',  ( -10.11138388277261946, 26.74549871207304363, 140.0000000000000000 ) ) ;
#62453=ORIENTED_EDGE ( 'NONE', *, *, #189014, .F. ) ;
#62502=CARTESIAN_POINT ( 'NONE',  ( -24.86035471869041302, 4.680034064337904809, 169.8578160361100799 ) ) ;
#62566=CARTESIAN_POINT ( 'NONE',  ( -8.571926809382608425, 26.38167802310805854, 148.4750000027311785 ) ) ;
#62579=CARTESIAN_POINT ( 'NONE',  ( 27.88129983271663903, -6.733757357602863536, 162.1517353552116560 ) ) ;
#62602=CARTESIAN_POINT ( 'NONE',  ( -27.12243378312308195, -3.972435522077939929, 169.3718635229810729 ) ) ;
#62650=CARTESIAN_POINT ( 'NONE',  ( -3.573655867282028392E-15, 2.428612866367529932E-14, 165.8682408883346397 ) ) ;
#62652=CARTESIAN_POINT ( 'NONE',  ( -3.573655867282028392E-15, 2.428612866367529932E-14, 165.8682408883346397 ) ) ;
#62654=CARTESIAN_POINT ( 'NONE',  ( -25.79025989231046623, -10.69883710965550527, 166.5180000355201742 ) ) ;
#62693=CARTESIAN_POINT ( 'NONE',  ( 17.79613651744293534, 24.49428055684532524, 149.2843446569000037 ) ) ;
#62727=CARTESIAN_POINT ( 'NONE',  ( -17.14385361876520264, -23.59649016807271593, 141.1750000027311671 ) ) ;
#62775=LINE ( 'NONE', #121474, #200166 ) ;
#62867=CARTESIAN_POINT ( 'NONE',  ( 28.82186960331499392, -9.364793116373510529, 142.9000000000000057 ) ) ;
#62881=CARTESIAN_POINT ( 'NONE',  ( 26.79623349963120660, -5.044589688426930785, 170.2051123914326070 ) ) ;
#62888=CARTESIAN_POINT ( 'NONE',  ( 21.65274598442062626, -9.891030456500306656, 170.6639841963363438 ) ) ;
#62896=( BOUNDED_CURVE ( )  B_SPLINE_CURVE ( 2, ( #99335, #69005, #5325, #80184, #141856, #65022, #98318, #126678, #128668, #174207, #188382 ),
 .UNSPECIFIED., .F., .F. ) 
 B_SPLINE_CURVE_WITH_KNOTS ( ( 3, 2, 2, 2, 2, 3 ),
 ( 0.000000000000000000, 0.02000000000000001776, 0.04000000000000003553, 0.06000000000000005329, 0.08000000000000007105, 0.1000000000000000888 ),
 .UNSPECIFIED. ) 
 CURVE ( )  GEOMETRIC_REPRESENTATION_ITEM ( )  RATIONAL_B_SPLINE_CURVE ( ( 1.000000000000000000, 0.9510565162951535312, 1.000000000000000000, 0.9510565162951535312, 1.000000000000000000, 0.9510565162951535312, 1.000000000000000000, 0.9510565162951535312, 1.000000000000000000, 0.9510565162951533091, 1.000000000000000222 ) ) 
 REPRESENTATION_ITEM ( '' )  );
#62900=FACE_OUTER_BOUND ( 'NONE', #146917, .T. ) ;
#62971=ORIENTED_EDGE ( 'NONE', *, *, #116692, .F. ) ;
#62984=CARTESIAN_POINT ( 'NONE',  ( -8.571926809382601320, -26.38167802310801591, 147.7750000027311899 ) ) ;
#63006=CARTESIAN_POINT ( 'NONE',  ( -25.82491430096448681, -7.758527484246124040, 169.9682266581730232 ) ) ;
#63021=CIRCLE ( 'NONE', #172735, 4.999999999999998224 ) ;
#63049=LINE ( 'NONE', #17555, #37403 ) ;
#63156=ORIENTED_EDGE ( 'NONE', *, *, #125997, .F. ) ;
#63223=CARTESIAN_POINT ( 'NONE',  ( 27.73933785331498569, 2.768321779492822058E-14, 148.3750000027311842 ) ) ;
#63403=EDGE_LOOP ( 'NONE', ( #100641, #65175, #20997, #81111 ) ) ;
#63459=CARTESIAN_POINT ( 'NONE',  ( -28.79475375365586842, 2.428612866367529932E-14, 143.9843446568999923 ) ) ;
#63513=CARTESIAN_POINT ( 'NONE',  ( -24.17640770809925854, 7.553848413212390867, 169.9412368235690565 ) ) ;
#63577=CARTESIAN_POINT ( 'NONE',  ( 1.784210473542230573E-15, -29.16686587814331588, 139.3750000027311842 ) ) ;
#63582=VERTEX_POINT ( 'NONE', #87825 ) ;
#63614=CARTESIAN_POINT ( 'NONE',  ( 24.69864206457978639, 7.736332803992567619, 171.5373547058828763 ) ) ;
#63663=DIRECTION ( 'NONE',  ( 0.000000000000000000, 0.000000000000000000, -1.000000000000000000 ) ) ;
#63740=CARTESIAN_POINT ( 'NONE',  ( -27.73933785331498925, -9.013057229001049109, 138.9750000027311785 ) ) ;
#63879=CARTESIAN_POINT ( 'NONE',  ( 23.31738231874054890, -16.94106989632523508, 140.7999999999999829 ) ) ;
#63898=( LENGTH_UNIT ( ) NAMED_UNIT ( * ) SI_UNIT ( .MILLI., .METRE. ) );
#63973=CARTESIAN_POINT ( 'NONE',  ( 23.31738231874054890, -16.94106989632523508, 147.0500000054623797 ) ) ;
#63978=ORIENTED_EDGE ( 'NONE', *, *, #55785, .F. ) ;
#64051=CARTESIAN_POINT ( 'NONE',  ( -17.79613651744293890, -24.49428055684527550, 148.2843446568999752 ) ) ;
#64141=CARTESIAN_POINT ( 'NONE',  ( 11.49674612099286719, -25.26099202438251723, 140.0000000000000000 ) ) ;
#64370=ADVANCED_FACE ( 'NONE', ( #32884 ), #58495, .T. ) ;
#64407=DIRECTION ( 'NONE',  ( 0.1039620511844979306, 0.1039620511844979306, -0.9891328443778538704 ) ) ;
#64415=CARTESIAN_POINT ( 'NONE',  ( 8.211251140130430670, 27.09903948220703995, 139.9999999999999147 ) ) ;
#64506=CARTESIAN_POINT ( 'NONE',  ( -24.51266705573315718, 8.027923408435372110, 167.0300397585818928 ) ) ;
#64545=CARTESIAN_POINT ( 'NONE',  ( -29.15849868437705439, 5.438282248597753110, 174.2683007571264113 ) ) ;
#64568=CARTESIAN_POINT ( 'NONE',  ( 19.49401214000076621, 12.39993551617566681, 169.9999999999999716 ) ) ;
#64573=CARTESIAN_POINT ( 'NONE',  ( -17.14385361876520619, 23.59649016807275856, 140.5750000027311728 ) ) ;
#64589=PRODUCT_DEFINITION_CONTEXT ( 'detailed design', #164372, 'design' ) ;
#64702=CARTESIAN_POINT ( 'NONE',  ( 23.29544513554940011, 16.92513159979228021, 149.1843446569000093 ) ) ;
#64800=CARTESIAN_POINT ( 'NONE',  ( 21.98685479826779599, 13.98560643873834231, 165.5209445330007725 ) ) ;
#64880=CARTESIAN_POINT ( 'NONE',  ( 26.77313074627600287, -4.631999166350020403, 170.7390164845734546 ) ) ;
#64897=CARTESIAN_POINT ( 'NONE',  ( -3.573655867282028392E-15, 2.428612866367529932E-14, 155.0000000000000000 ) ) ;
#64921=CARTESIAN_POINT ( 'NONE',  ( 21.38418241377623019, 7.427326039334300134, 174.4773576836617224 ) ) ;
#64959=CARTESIAN_POINT ( 'NONE',  ( 28.79475375365586132, 2.781246896534039337E-14, 148.9843446568999923 ) ) ;
#64973=CARTESIAN_POINT ( 'NONE',  ( -27.73933785331498925, -9.013057229001049109, 147.4750000027311785 ) ) ;
#65022=CARTESIAN_POINT ( 'NONE',  ( -5.427562675786936573E-15, 30.27659582821221207, 147.7656553485623760 ) ) ;
#65175=ORIENTED_EDGE ( 'NONE', *, *, #155178, .T. ) ;
#65245=CARTESIAN_POINT ( 'NONE',  ( -25.70602947687971351, -7.354137148287275494, 175.2376750527030822 ) ) ;
#65488=CARTESIAN_POINT ( 'NONE',  ( -24.24393946303101544, 5.863316274098875347, 172.4343578713345266 ) ) ;
#65539=AXIS2_PLACEMENT_3D ( 'NONE', #153481, #75642, #181854 ) ;
#65555=CARTESIAN_POINT ( 'NONE',  ( 27.73933785331498925, -9.013057229001033122, 139.7750000027311899 ) ) ;
#65717=CARTESIAN_POINT ( 'NONE',  ( 22.44159573604009594, -16.30477369853687364, 139.6750000027311955 ) ) ;
#65865=CARTESIAN_POINT ( 'NONE',  ( 21.97054992548899222, -8.562709642470922589, 171.7904333278019351 ) ) ;
#65907=ORIENTED_EDGE ( 'NONE', *, *, #24178, .F. ) ;
#65947=CARTESIAN_POINT ( 'NONE',  ( -28.82186960331499392, 9.364793116373565596, 144.1500000054623740 ) ) ;
#65961=CARTESIAN_POINT ( 'NONE',  ( -27.73933785331498925, 2.428612866367529932E-14, 149.3750000027311842 ) ) ;
#66087=VERTEX_POINT ( 'NONE', #82857 ) ;
#66207=( BOUNDED_CURVE ( )  B_SPLINE_CURVE ( 2, ( #89005, #41524, #75810, #12194, #152653, #181043, #150696, #27359, #183014, #14143, #73859 ),
 .UNSPECIFIED., .F., .T. ) 
 B_SPLINE_CURVE_WITH_KNOTS ( ( 3, 2, 2, 2, 2, 3 ),
 ( 0.6000000000000033085, 0.6200000000000033262, 0.6400000000000033440, 0.6600000000000034728, 0.6800000000000034905, 0.7000000000000033973 ),
 .UNSPECIFIED. ) 
 CURVE ( )  GEOMETRIC_REPRESENTATION_ITEM ( )  RATIONAL_B_SPLINE_CURVE ( ( 0.9999999999999918954, 0.9510565162951616358, 1.000000000000000000, 0.9510565162951535312, 1.000000000000000000, 0.9510565162951535312, 1.000000000000000000, 0.9510565162951535312, 1.000000000000000000, 0.9510565162951450935, 1.000000000000008438 ) ) 
 REPRESENTATION_ITEM ( '' )  );
#66229=CARTESIAN_POINT ( 'NONE',  ( 25.57682740168941748, -5.495034664247685718, 164.9437814717016408 ) ) ;
#66383=EDGE_LOOP ( 'NONE', ( #174642, #97767, #69447, #117609 ) ) ;
#66397=CARTESIAN_POINT ( 'NONE',  ( 27.95742675678724609, 7.330130391636824783, 160.9071069586348415 ) ) ;
#66415=TOROIDAL_SURFACE ( 'NONE', #11764, 23.10356920737165254, 3.000000000000000000 ) ;
#66504=EDGE_CURVE ( 'NONE', #110081, #100463, #177287, .T. ) ;
#66583=B_SPLINE_CURVE_WITH_KNOTS ( 'NONE', 3,
 ( #14963, #76623, #184804, #154467, #15959, #77619, #139289, #766, #124110, #53245, #144253, #145251, #131083, #67416 ),
 .UNSPECIFIED., .F., .F.,
 ( 4, 2, 2, 2, 2, 2, 4 ),
 ( 3.469446951953614189E-18, 0.002289927113134828090, 0.003434890669702238015, 0.004579854226269648373, 0.006869781339404439600, 0.008014744895971813096, 0.009159708452539187459 ),
 .UNSPECIFIED. ) ;
#66645=EDGE_CURVE ( 'NONE', #48040, #177604, #41080, .T. ) ;
#66692=VERTEX_POINT ( 'NONE', #117207 ) ;
#66750=CARTESIAN_POINT ( 'NONE',  ( 23.48258780958830982, -5.709364865862134764, 171.6892424014283733 ) ) ;
#66778=CARTESIAN_POINT ( 'NONE',  ( 28.79475375365586132, 2.781246896534039337E-14, 155.0000000000000000 ) ) ;
#66792=VECTOR ( 'NONE', #105181, 1000.000000000000000 ) ;
#66863=CARTESIAN_POINT ( 'NONE',  ( 24.86475712555791873, -11.37215039201027089, 169.9824823118007657 ) ) ;
#66874=CARTESIAN_POINT ( 'NONE',  ( 23.58955696227031140, -7.613471476246058245, 172.7063021553927058 ) ) ;
#66887=CARTESIAN_POINT ( 'NONE',  ( -27.73933785331498925, -9.013057229001049109, 142.9750000027312069 ) ) ;
#66945=CARTESIAN_POINT ( 'NONE',  ( 22.44159573604009594, -16.30477369853687364, 140.1750000027311955 ) ) ;
#66946=CARTESIAN_POINT ( 'NONE',  ( 17.81289503416610742, 24.51734667627700404, 143.5500000054623513 ) ) ;
#66961=CARTESIAN_POINT ( 'NONE',  ( 27.73933785331498569, 9.013057229001093518, 148.4750000027311785 ) ) ;
#66985=DIRECTION ( 'NONE',  ( 0.000000000000000000, 0.000000000000000000, 1.000000000000000000 ) ) ;
#67009=DIRECTION ( 'NONE',  ( 1.000000000000000000, 0.000000000000000000, -0.000000000000000000 ) ) ;
#67107=VECTOR ( 'NONE', #80692, 1000.000000000000000 ) ;
#67114=CARTESIAN_POINT ( 'NONE',  ( -28.79475375365577250, -9.355982642739318678, 144.0843446569000150 ) ) ;
#67200=CARTESIAN_POINT ( 'NONE',  ( -24.93942350307309752, 7.769968609432599926, 171.2173313942149946 ) ) ;
#67312=CARTESIAN_POINT ( 'NONE',  ( -3.573655867282028392E-15, 2.428612866367529932E-14, 155.0000000000000000 ) ) ;
#67377=CARTESIAN_POINT ( 'NONE',  ( -28.79475375365586842, 2.428612866367529932E-14, 147.9843446568999923 ) ) ;
#67416=CARTESIAN_POINT ( 'NONE',  ( -24.81835718235489097, -6.052279806424480491, 168.4265042179603427 ) ) ;
#67426=CARTESIAN_POINT ( 'NONE',  ( 26.53315420742544717, 7.611574518544833801, 168.2743882774363726 ) ) ;
#67491=ADVANCED_FACE ( 'NONE', ( #98920 ), #115105, .T. ) ;
#67539=CARTESIAN_POINT ( 'NONE',  ( 21.59136165864583390, 7.527668378163610896, 173.8290135686407893 ) ) ;
#67557=CARTESIAN_POINT ( 'NONE',  ( 27.60788766665615768, -7.718175339870845697, 162.2452582881560943 ) ) ;
#67580=CARTESIAN_POINT ( 'NONE',  ( 22.67087683854552083, 7.530304285672279718, 173.4975851171454622 ) ) ;
#67778=CARTESIAN_POINT ( 'NONE',  ( 21.51693143705272959, 9.260949364272169859, 168.7281092719942990 ) ) ;
#67859=VERTEX_POINT ( 'NONE', #96931 ) ;
#67888=CARTESIAN_POINT ( 'NONE',  ( -17.14385361876520975, 23.59649016807275856, 140.5750000027311444 ) ) ;
#67922=ORIENTED_EDGE ( 'NONE', *, *, #114385, .F. ) ;
#67944=CARTESIAN_POINT ( 'NONE',  ( -28.82186960331499392, 9.364793116373565596, 146.1500000054623456 ) ) ;
#67956=CARTESIAN_POINT ( 'NONE',  ( -27.73933785331498925, 2.428612866367529932E-14, 141.3750000027311842 ) ) ;
#68125=UNCERTAINTY_MEASURE_WITH_UNIT (LENGTH_MEASURE( 1.000000000000000082E-05 ), #63898, 'distance_accuracy_value', 'NONE');
#68165=CARTESIAN_POINT ( 'NONE',  ( -25.78958964901898554, 10.70071173758531557, 166.5174151181484490 ) ) ;
#68275=EDGE_CURVE ( 'NONE', #67859, #15498, #134872, .T. ) ;
#68306=VERTEX_POINT ( 'NONE', #136259 ) ;
#68383=CARTESIAN_POINT ( 'NONE',  ( 27.83962847748220781, 7.578403945688395815, 161.1890875223823514 ) ) ;
#68410=CARTESIAN_POINT ( 'NONE',  ( -22.40075113267185714, 13.33491755757043506, 165.5209445330008009 ) ) ;
#68432=CARTESIAN_POINT ( 'NONE',  ( -22.37486833544133091, -13.37560805684351450, 165.5209445320977864 ) ) ;
#68471=CARTESIAN_POINT ( 'NONE',  ( 21.47377332592399668, -5.474134792251643233, 173.8918256800999984 ) ) ;
#68495=ORIENTED_EDGE ( 'NONE', *, *, #178481, .T. ) ;
#68517=CARTESIAN_POINT ( 'NONE',  ( 24.39440776506090103, 8.562465606919662520, 166.7298475161184683 ) ) ;
#68575=( BOUNDED_SURFACE ( )  B_SPLINE_SURFACE ( 3, 2, ( 
 ( #37739, #130739, #6389 ),
 ( #40744, #36725, #191419 ),
 ( #116581, #54908, #100405 ),
 ( #176267, #192431, #132747 ),
 ( #190430, #8408, #129722 ),
 ( #69072, #193432, #178270 ),
 ( #83231, #23580, #144906 ),
 ( #179279, #70082, #39733 ),
 ( #101394, #162086, #131750 ),
 ( #194435, #128734, #52895 ),
 ( #99400, #163087, #161083 ),
 ( #53913, #85228, #22578 ),
 ( #146919, #24591, #86239 ),
 ( #55906, #117579, #84225 ),
 ( #145904, #7388, #115588 ),
 ( #180282, #152880, #27594 ),
 ( #183242, #195442, #73092 ),
 ( #58889, #75056, #44723 ),
 ( #106379, #14375, #120555 ),
 ( #60864, #76041, #137716 ),
 ( #119587, #165094, #197423 ),
 ( #12419, #182248, #148927 ),
 ( #56917, #199400, #43733 ),
 ( #72074, #28583, #89232 ) ),
 .UNSPECIFIED., .F., .F., .T. ) 
 B_SPLINE_SURFACE_WITH_KNOTS ( ( 4, 2, 2, 2, 2, 2, 2, 2, 2, 2, 2, 4 ),
 ( 3, 3 ),
 ( -8.673617379884035472E-19, 0.001899702839891689908, 0.002849554259837535405, 0.003799405679783380684, 0.005699108519675071677, 0.006648959939620916956, 0.007598811359566762236, 0.008548662779512607515, 0.009498514199458452795, 0.01139821703935014335, 0.01329791987924183391, 0.01519762271913352447 ),
 ( 0.000000000000000000, 1.000000000000000000 ),
 .UNSPECIFIED. ) 
 GEOMETRIC_REPRESENTATION_ITEM ( )  RATIONAL_B_SPLINE_SURFACE ( (
 ( 1.000000000000000000, 0.7660444431189777914, 1.000000000000000000),
 ( 1.000000000000000000, 0.7753720600381861505, 1.000000000000000000),
 ( 1.000000000000000000, 0.7832595754286625356, 1.000000000000000000),
 ( 1.000000000000000000, 0.7928595458705119947, 1.000000000000000000),
 ( 1.000000000000000000, 0.7956872332516092827, 1.000000000000000000),
 ( 1.000000000000000000, 0.8005750596157589216, 1.000000000000000000),
 ( 1.000000000000000000, 0.8026302056541690932, 1.000000000000000000),
 ( 1.000000000000000000, 0.8075080643848435713, 1.000000000000000000),
 ( 1.000000000000000000, 0.8091143015809740824, 1.000000000000000000),
 ( 1.000000000000000000, 0.8093067629633081683, 1.000000000000000000),
 ( 1.000000000000000000, 0.8089952915731970506, 1.000000000000000000),
 ( 1.000000000000000000, 0.8076919994861997409, 1.000000000000000000),
 ( 1.000000000000000000, 0.8067078407648531346, 1.000000000000000000),
 ( 1.000000000000000000, 0.8041786842467797403, 1.000000000000000000),
 ( 1.000000000000000000, 0.8026334674877259046, 1.000000000000000000),
 ( 1.000000000000000000, 0.7990747329469148896, 1.000000000000000000),
 ( 1.000000000000000000, 0.7970509760942132704, 1.000000000000000000),
 ( 1.000000000000000000, 0.7904793850862674720, 1.000000000000000000),
 ( 1.000000000000000000, 0.7855040224314492336, 1.000000000000000000),
 ( 1.000000000000000000, 0.7751942650506803423, 1.000000000000000000),
 ( 1.000000000000000000, 0.7698260778211011290, 1.000000000000000000),
 ( 1.000000000000000000, 0.7598259884961470201, 1.000000000000000000),
 ( 1.000000000000000000, 0.7551428682219897270, 1.000000000000000000),
 ( 1.000000000000000000, 0.7510191126010854479, 1.000000000000000000) ) ) 
 REPRESENTATION_ITEM ( '' )  SURFACE ( )  );
#68669=APPLICATION_CONTEXT ( 'automotive_design' ) ;
#68760=CARTESIAN_POINT ( 'NONE',  ( -27.88129983271673851, -6.733757357603135318, 162.1517353552107750 ) ) ;
#68890=CARTESIAN_POINT ( 'NONE',  ( 27.73933785331498569, 9.013057229001093518, 143.9750000027312069 ) ) ;
#68945=CARTESIAN_POINT ( 'NONE',  ( -27.73933785331498925, 9.013057229001089965, 148.7750000027311899 ) ) ;
#68959=CARTESIAN_POINT ( 'NONE',  ( 27.73933785331498569, 2.768321779492822058E-14, 144.3750000027311842 ) ) ;
#69005=CARTESIAN_POINT ( 'NONE',  ( -28.79475375365586842, 9.355982642739222754, 148.1656553485623533 ) ) ;
#69029=CARTESIAN_POINT ( 'NONE',  ( -21.94905633995364269, 8.886455535323596777, 171.4390084046502523 ) ) ;
#69072=CARTESIAN_POINT ( 'NONE',  ( 20.93662873023604121, 11.00447265502299388, 170.1964094900432372 ) ) ;
#69112=LINE ( 'NONE', #88026, #46384 ) ;
#69116=CARTESIAN_POINT ( 'NONE',  ( 28.79475375365586132, 2.781246896534039337E-14, 140.9843446568999923 ) ) ;
#69189=VERTEX_POINT ( 'NONE', #91714 ) ;
#69312=ORIENTED_EDGE ( 'NONE', *, *, #93066, .T. ) ;
#69438=CARTESIAN_POINT ( 'NONE',  ( -21.35462415990328822, -9.648971641163925028, 168.5494316893072835 ) ) ;
#69447=ORIENTED_EDGE ( 'NONE', *, *, #55785, .T. ) ;
#69478=CARTESIAN_POINT ( 'NONE',  ( 23.75112013235311892, -10.51683317207933399, 166.0021274478077942 ) ) ;
#69618=CARTESIAN_POINT ( 'NONE',  ( -19.80295450558176640, 12.05995242899444797, 167.9999999999999716 ) ) ;
#69634=DIRECTION ( 'NONE',  ( -1.000000000000000000, 0.000000000000000000, 0.000000000000000000 ) ) ;
#69766=CARTESIAN_POINT ( 'NONE',  ( -3.573655867282028392E-15, 2.428612866367529932E-14, 167.9999999999999716 ) ) ;
#69870=CARTESIAN_POINT ( 'NONE',  ( -25.25560589046783733, 4.310829775027161581, 167.9999999999999716 ) ) ;
#69896=CARTESIAN_POINT ( 'NONE',  ( -27.73933785331498925, 2.428612866367529932E-14, 140.8750000027311842 ) ) ;
#69903=EDGE_CURVE ( 'NONE', #146141, #18152, #35037, .T. ) ;
#69955=CARTESIAN_POINT ( 'NONE',  ( 27.73933785331498569, 2.768321779492822058E-14, 140.3750000027311842 ) ) ;
#69956=CARTESIAN_POINT ( 'NONE',  ( -5.359611314223446995E-15, 29.16686587814335496, 148.3750000027311842 ) ) ;
#69969=CARTESIAN_POINT ( 'NONE',  ( -27.73933785331498925, -9.013057229001049109, 141.4750000027312069 ) ) ;
#70025=CARTESIAN_POINT ( 'NONE',  ( -28.28060372831499336, 2.428612866367529932E-14, 148.5625000040967620 ) ) ;
#70082=CARTESIAN_POINT ( 'NONE',  ( 24.86475712555687423, 11.37215039201022293, 169.9824823118007657 ) ) ;
#70093=CARTESIAN_POINT ( 'NONE',  ( 8.571926809382597767, 26.38167802310806209, 140.7750000027311899 ) ) ;
#70125=CARTESIAN_POINT ( 'NONE',  ( -17.79613651744294600, 24.49428055684532524, 145.9656553485623647 ) ) ;
#70181=CARTESIAN_POINT ( 'NONE',  ( -28.79475375365484524, 9.355982642740638511, 140.1656553485623533 ) ) ;
#70240=CARTESIAN_POINT ( 'NONE',  ( -21.96449396329681392, -6.689387493872139601, 170.9254202302468855 ) ) ;
#70267=ORIENTED_EDGE ( 'NONE', *, *, #151508, .F. ) ;
#70284=DIRECTION ( 'NONE',  ( 0.000000000000000000, 0.000000000000000000, 1.000000000000000000 ) ) ;
#70361=CARTESIAN_POINT ( 'NONE',  ( 24.02706313830236695, -14.44797190822832889, 165.8682408883346397 ) ) ;
#70413=VERTEX_POINT ( 'NONE', #154054 ) ;
#70422=AXIS2_PLACEMENT_3D ( 'NONE', #43490, #183983, #13158 ) ;
#70445=CARTESIAN_POINT ( 'NONE',  ( -24.51266705573320692, -8.027923408435210462, 167.0300397585817791 ) ) ;
#70482=FACE_OUTER_BOUND ( 'NONE', #19410, .T. ) ;
#70527=CARTESIAN_POINT ( 'NONE',  ( 24.60782464877076947, 7.576768089025934572, 167.2921030401324742 ) ) ;
#70540=EDGE_CURVE ( 'NONE', #34840, #42860, #80181, .T. ) ;
#70622=CARTESIAN_POINT ( 'NONE',  ( -27.81654016797119766, -7.031644252044944920, 140.0000000000000284 ) ) ;
#70637=CARTESIAN_POINT ( 'NONE',  ( 22.15208335914313409, 5.528296758471276107, 173.4118699040215006 ) ) ;
#70694=DIRECTION ( 'NONE',  ( 1.000000000000000000, -0.000000000000000000, -0.000000000000000000 ) ) ;
#70773=CARTESIAN_POINT ( 'NONE',  ( -27.79720911487485324, -7.618197028333625553, 161.3616953378478343 ) ) ;
#70787=CARTESIAN_POINT ( 'NONE',  ( 24.40828949532285819, 2.848420800298366196, 173.9378174459544937 ) ) ;
#70806=ADVANCED_FACE ( 'NONE', ( #44897 ), #172204, .T. ) ;
#70826=VECTOR ( 'NONE', #141720, 1000.000000000000114 ) ;
#70875=CARTESIAN_POINT ( 'NONE',  ( -25.31894786019269361, 4.571304203950368183, 167.3973414147895085 ) ) ;
#70900=CARTESIAN_POINT ( 'NONE',  ( 8.571926809382597767, 26.38167802310806209, 142.2750000027311899 ) ) ;
#70954=CARTESIAN_POINT ( 'NONE',  ( 17.14385361876520264, -23.59649016807271238, 140.0750000027311728 ) ) ;
#70956=CARTESIAN_POINT ( 'NONE',  ( 8.906447517083050158, 27.41122689804195645, 139.6500000054623740 ) ) ;
#70970=CARTESIAN_POINT ( 'NONE',  ( -8.571926809382608425, 26.38167802310805854, 142.9750000027312069 ) ) ;
#70994=AXIS2_PLACEMENT_3D ( 'NONE', #130305, #85822, #147510 ) ;
#71040=CARTESIAN_POINT ( 'NONE',  ( -26.38458505201399618, 8.641005086744664609, 167.3773361139123494 ) ) ;
#71091=CARTESIAN_POINT ( 'NONE',  ( -27.73933785331498925, -9.013057229001049109, 139.4750000027311785 ) ) ;
#71251=CARTESIAN_POINT ( 'NONE',  ( 17.14385361876520264, -23.59649016807270883, 145.5750000027311728 ) ) ;
#71262=CARTESIAN_POINT ( 'NONE',  ( 26.26106931734003425, 9.140213825779245127, 167.1341548181404164 ) ) ;
#71325=ORIENTED_EDGE ( 'NONE', *, *, #104490, .T. ) ;
#71374=ORIENTED_EDGE ( 'NONE', *, *, #121851, .F. ) ;
#71433=B_SPLINE_CURVE_WITH_KNOTS ( 'NONE', 3,
 ( #196049, #30152, #149520, #91794, #136341, #181860, #43339, #27191, #57524, #121159, #14984, #135365, #166693, #44335, #197036, #118193, #89838, #58503, #105007, #137326, #105992, #88838 ),
 .UNSPECIFIED., .F., .F.,
 ( 4, 2, 2, 2, 2, 2, 2, 2, 2, 2, 4 ),
 ( 0.000000000000000000, 0.001027542925581684209, 0.002055085851163368418, 0.002568857313954213666, 0.003082628776745058915, 0.004110171702326815765, 0.004623943165117716525, 0.005137714627908618152, 0.006165257553490454366, 0.007192800479072292315, 0.008220343404654129396 ),
 .UNSPECIFIED. ) ;
#71479=CARTESIAN_POINT ( 'NONE',  ( 23.63516320021125594, -9.722623904421409335, 168.4908852323012809 ) ) ;
#71581=CARTESIAN_POINT ( 'NONE',  ( 19.80313217313587870, 12.05975691044382181, 167.9999999999999147 ) ) ;
#71714=DIRECTION ( 'NONE',  ( 0.000000000000000000, -0.000000000000000000, -1.000000000000000000 ) ) ;
#71781=CARTESIAN_POINT ( 'NONE',  ( 24.04614410382215084, 5.408324479805897589, 174.2944578187874072 ) ) ;
#71949=CARTESIAN_POINT ( 'NONE',  ( 27.73933785331498925, -9.013057229001033122, 147.7750000027311899 ) ) ;
#71961=CARTESIAN_POINT ( 'NONE',  ( 17.14385361876520264, -23.59649016807270883, 142.0750000027311444 ) ) ;
#72032=CARTESIAN_POINT ( 'NONE',  ( -20.14845677604832375, 11.85354687992394496, 170.0217845860066745 ) ) ;
#72064=VECTOR ( 'NONE', #13689, 1000.000000000000114 ) ;
#72074=CARTESIAN_POINT ( 'NONE',  ( 21.36928693577338834, 7.422813773936193016, 174.5222352431090087 ) ) ;
#72087=CARTESIAN_POINT ( 'NONE',  ( 23.31738231874054890, -16.94106989632523508, 148.7999999999999829 ) ) ;
#72105=ORIENTED_EDGE ( 'NONE', *, *, #141591, .T. ) ;
#72247=CARTESIAN_POINT ( 'NONE',  ( -27.73933785331498925, -9.013057229001049109, 144.9750000027312069 ) ) ;
#72281=CARTESIAN_POINT ( 'NONE',  ( -3.573655867282028392E-15, 2.428612866367529932E-14, 169.9999999999999716 ) ) ;
#72338=ORIENTED_EDGE ( 'NONE', *, *, #114385, .T. ) ;
#72438=AXIS2_PLACEMENT_3D ( 'NONE', #64897, #50733, #186276 ) ;
#72450=FACE_OUTER_BOUND ( 'NONE', #39824, .T. ) ;
#72486=CARTESIAN_POINT ( 'NONE',  ( 21.92083080610821355, -6.374575339255582840, 171.4095429173268599 ) ) ;
#72592=CARTESIAN_POINT ( 'NONE',  ( 21.97143472835163891, 7.273127645264538366, 170.2116391040482313 ) ) ;
#72623=ORIENTED_EDGE ( 'NONE', *, *, #43155, .T. ) ;
#72626=CARTESIAN_POINT ( 'NONE',  ( -21.38418241377624085, 5.438282248597754887, 174.2683007571264113 ) ) ;
#72690=CARTESIAN_POINT ( 'NONE',  ( -20.02432819973542877, 11.96332215053014636, 170.0134113894037000 ) ) ;
#72797=CARTESIAN_POINT ( 'NONE',  ( 24.66578506923905323, 3.377805382905409104, 172.1149105766468494 ) ) ;
#72892=LINE ( 'NONE', #196248, #108979 ) ;
#72968=CARTESIAN_POINT ( 'NONE',  ( -23.31738231874055245, -16.94106989632524574, 142.4500000054623854 ) ) ;
#72980=CARTESIAN_POINT ( 'NONE',  ( 10.65970682939788716, -25.60940286011448919, 139.9999999999999716 ) ) ;
#72997=CONICAL_SURFACE ( 'NONE', #131132, 30.82560697742735556, 0.1745329251994333364 ) ;
#73009=PLANE ( 'NONE',  #145128 ) ;
#73048=CARTESIAN_POINT ( 'NONE',  ( -21.36928693577339544, 7.422813773936193016, 174.5222352431090087 ) ) ;
#73092=CARTESIAN_POINT ( 'NONE',  ( 26.78465914369782297, 5.761000505272440897, 169.4491075441771670 ) ) ;
#73104=AXIS2_PLACEMENT_3D ( 'NONE', #94498, #155192, #29868 ) ;
#73106=CARTESIAN_POINT ( 'NONE',  ( 8.906447517083057264, -27.41122689804191026, 146.5999999999999943 ) ) ;
#73262=CARTESIAN_POINT ( 'NONE',  ( 17.14385361876520264, 23.59649016807275856, 146.1750000027311387 ) ) ;
#73274=PLANE ( 'NONE',  #151956 ) ;
#73397=ORIENTED_EDGE ( 'NONE', *, *, #136828, .F. ) ;
#73458=DIRECTION ( 'NONE',  ( 0.1045284632676537068, 0.000000000000000000, 0.9945218953682734009 ) ) ;
#73492=CARTESIAN_POINT ( 'NONE',  ( -24.95262708931866058, -12.69764001896745143, 166.0532406165023360 ) ) ;
#73626=ORIENTED_EDGE ( 'NONE', *, *, #104106, .T. ) ;
#73628=CARTESIAN_POINT ( 'NONE',  ( -21.81399809961444802, 8.291606000631404072, 169.3279294801716617 ) ) ;
#73656=CARTESIAN_POINT ( 'NONE',  ( -8.898068258721469448, -27.38543819252872069, 144.6656553485624102 ) ) ;
#73716=CARTESIAN_POINT ( 'NONE',  ( 23.71437922609630178, -10.61260870832703773, 165.9744018657352456 ) ) ;
#73773=CARTESIAN_POINT ( 'NONE',  ( 17.79613651744294245, -24.49428055684527195, 142.6843446568999809 ) ) ;
#73797=CARTESIAN_POINT ( 'NONE',  ( -27.73933785331498925, -9.013057229001049109, 144.9750000027312069 ) ) ;
#73856=ORIENTED_EDGE ( 'NONE', *, *, #160998, .T. ) ;
#73859=CARTESIAN_POINT ( 'NONE',  ( 28.79475375365586132, 2.781246896534039337E-14, 141.2656553485623760 ) ) ;
#73885=CARTESIAN_POINT ( 'NONE',  ( -27.88129983271662837, 6.733757357602863536, 162.1517353552117982 ) ) ;
#73950=MANIFOLD_SOLID_BREP ( 'Cavity1', #117602 ) ;
#73959=CYLINDRICAL_SURFACE ( 'NONE', #30560, 28.79475375365586487 ) ;
#73960=CARTESIAN_POINT ( 'NONE',  ( 17.14385361876520264, -23.59649016807271238, 145.5750000027312012 ) ) ;
#74025=CARTESIAN_POINT ( 'NONE',  ( -3.573655867282028392E-15, 2.428612866367529932E-14, 149.6527036446661327 ) ) ;
#74039=CARTESIAN_POINT ( 'NONE',  ( -9.708182408413708941, -26.42831169063299157, 139.9999999999999716 ) ) ;
#74095=CARTESIAN_POINT ( 'NONE',  ( 28.82186960331498327, 2.781578969918950771E-14, 147.0000000000000000 ) ) ;
#74110=CARTESIAN_POINT ( 'NONE',  ( 23.64729612845458817, -13.72274676820368633, 169.8070494178799663 ) ) ;
#74126=CARTESIAN_POINT ( 'NONE',  ( 25.25560589046783022, -4.310829775027113620, 167.9999999999999716 ) ) ;
#74210=EDGE_CURVE ( 'NONE', #104760, #18152, #173885, .T. ) ;
#74246=CARTESIAN_POINT ( 'NONE',  ( 22.44159573604009239, 16.30477369853692693, 146.0750000027311728 ) ) ;
#74382=CARTESIAN_POINT ( 'NONE',  ( 21.94595931813856637, -7.591279830614304558, 169.8931963588656231 ) ) ;
#74390=DIRECTION ( 'NONE',  ( 1.000000000000000000, 0.000000000000000000, 0.000000000000000000 ) ) ;
#74434=CARTESIAN_POINT ( 'NONE',  ( 17.14385361876520264, -23.59649016807271238, 146.0750000027311728 ) ) ;
#74438=CARTESIAN_POINT ( 'NONE',  ( 22.44159573604009594, -16.30477369853687364, 148.1750000027311671 ) ) ;
#74477=CARTESIAN_POINT ( 'NONE',  ( -25.85231681326418851, -7.957828899753048191, 172.6576833274880869 ) ) ;
#74779=CARTESIAN_POINT ( 'NONE',  ( -17.14385361876520264, -23.59649016807271593, 143.1750000027311671 ) ) ;
#74862=LINE ( 'NONE', #125336, #157975 ) ;
#74864=CARTESIAN_POINT ( 'NONE',  ( -27.89965394715913760, 6.788920637341050224, 161.9771076211713137 ) ) ;
#74936=CARTESIAN_POINT ( 'NONE',  ( -27.73933785331498925, -9.013057229001049109, 146.9750000027311785 ) ) ;
#74976=FACE_OUTER_BOUND ( 'NONE', #128348, .T. ) ;
#75014=CARTESIAN_POINT ( 'NONE',  ( -21.95653654802720922, 8.266568072468359674, 172.1684357517875412 ) ) ;
#75056=CARTESIAN_POINT ( 'NONE',  ( 25.82893184620815319, 8.167111171437667849, 172.3011985515803701 ) ) ;
#75069=CARTESIAN_POINT ( 'NONE',  ( 28.82186960331499392, -9.364793116373510529, 144.9000000000000057 ) ) ;
#75092=CARTESIAN_POINT ( 'NONE',  ( -26.79475375365586842, 2.428612866367529932E-14, 139.9999999999999716 ) ) ;
#75107=CARTESIAN_POINT ( 'NONE',  ( 28.79475375365586132, 2.781246896534039337E-14, 155.0000000000000000 ) ) ;
#75166=CARTESIAN_POINT ( 'NONE',  ( -24.83221077041872960, -4.296110748029300375, 170.3917201292314303 ) ) ;
#75246=CARTESIAN_POINT ( 'NONE',  ( 28.79475375365609935, -9.355982642738862154, 148.8843446569000264 ) ) ;
#75405=AXIS2_PLACEMENT_3D ( 'NONE', #99311, #66985, #127655 ) ;
#75412=CARTESIAN_POINT ( 'NONE',  ( -27.73933785331498925, -9.013057229001049109, 141.4750000027311785 ) ) ;
#75416=CARTESIAN_POINT ( 'NONE',  ( 8.571926809382603096, -26.38167802310801235, 145.9750000027311785 ) ) ;
#75451=CARTESIAN_POINT ( 'NONE',  ( -21.73861122199297924, -7.688394669363364464, 173.2969830217473941 ) ) ;
#75553=EDGE_CURVE ( 'NONE', #16229, #2773, #24582, .T. ) ;
#75598=CARTESIAN_POINT ( 'NONE',  ( -19.30190589895974185, 21.36759865781276346, 139.9999999999999716 ) ) ;
#75626=FACE_OUTER_BOUND ( 'NONE', #45341, .T. ) ;
#75642=DIRECTION ( 'NONE',  ( -0.000000000000000000, -0.000000000000000000, -1.000000000000000000 ) ) ;
#75656=ORIENTED_EDGE ( 'NONE', *, *, #183623, .T. ) ;
#75662=CARTESIAN_POINT ( 'NONE',  ( 23.29544513554940011, 16.92513159979228021, 145.1843446569000093 ) ) ;
#75663=VERTEX_POINT ( 'NONE', #75839 ) ;
#75729=CARTESIAN_POINT ( 'NONE',  ( 1.988064558232696151E-15, -30.27659582821216588, 142.4843446568999923 ) ) ;
#75752=CARTESIAN_POINT ( 'NONE',  ( 17.14385361876520264, -23.59649016807271238, 143.5750000027312012 ) ) ;
#75810=CARTESIAN_POINT ( 'NONE',  ( -23.29544513554941076, 16.92513159979227666, 142.0656553485623590 ) ) ;
#75822=EDGE_CURVE ( 'NONE', #9294, #34941, #72892, .T. ) ;
#75839=CARTESIAN_POINT ( 'NONE',  ( -22.94331271462294808, 3.784814030245898575, 190.0000000000000000 ) ) ;
#75878=CARTESIAN_POINT ( 'NONE',  ( -3.573655867282028392E-15, 2.428612866367529932E-14, 169.9999999999999716 ) ) ;
#75881=PRODUCT_DEFINITION_FORMATION_WITH_SPECIFIED_SOURCE ( 'ANY', '', #95384, .NOT_KNOWN. ) ;
#75891=VERTEX_POINT ( 'NONE', #19155 ) ;
#75918=CARTESIAN_POINT ( 'NONE',  ( 27.73933785331498925, -9.013057229001033122, 145.7750000027311899 ) ) ;
#75954=ORIENTED_EDGE ( 'NONE', *, *, #74210, .T. ) ;
#75955=CARTESIAN_POINT ( 'NONE',  ( -28.75808110634262604, -1.452795517301058048, 139.9999999999999716 ) ) ;
#76032=CIRCLE ( 'NONE', #189064, 5.000000000000001776 ) ;
#76041=CARTESIAN_POINT ( 'NONE',  ( 25.86526910843881311, 7.630673861714906359, 173.3900163844835731 ) ) ;
#76055=CARTESIAN_POINT ( 'NONE',  ( 28.82186960331498327, 2.781578969918950771E-14, 145.0000000000000000 ) ) ;
#76057=EDGE_CURVE ( 'NONE', #105306, #18425, #163852, .T. ) ;
#76151=CARTESIAN_POINT ( 'NONE',  ( -24.85901545656360767, -5.346793810781480083, 169.1018111888377291 ) ) ;
#76153=ORIENTED_EDGE ( 'NONE', *, *, #193676, .T. ) ;
#76230=CARTESIAN_POINT ( 'NONE',  ( 8.898068258721473001, -27.38543819252872069, 148.5843446568999866 ) ) ;
#76266=( BOUNDED_CURVE ( )  B_SPLINE_CURVE ( 3, ( #88409, #132927, #149108, #178449 ),
 .UNSPECIFIED., .F., .F. ) 
 B_SPLINE_CURVE_WITH_KNOTS ( ( 4, 4 ),
 ( 5.503250352303675541, 7.063120262055496923 ),
 .UNSPECIFIED. ) 
 CURVE ( )  GEOMETRIC_REPRESENTATION_ITEM ( )  RATIONAL_B_SPLINE_CURVE ( ( 1.000000000000000000, 0.8073061876036304874, 0.8073061876036304874, 1.000000000000000000 ) ) 
 REPRESENTATION_ITEM ( '' )  );
#76404=CARTESIAN_POINT ( 'NONE',  ( 8.571926809382597767, 26.38167802310806209, 144.7750000027311899 ) ) ;
#76408=CARTESIAN_POINT ( 'NONE',  ( 8.571926809382603096, -26.38167802310801235, 147.9750000027311785 ) ) ;
#76444=CARTESIAN_POINT ( 'NONE',  ( -23.64874990377911601, -15.04272038711346582, 165.8682408883346397 ) ) ;
#76596=CARTESIAN_POINT ( 'NONE',  ( 18.76835711872175594, 20.78600286866540969, 140.0000000000000000 ) ) ;
#76623=CARTESIAN_POINT ( 'NONE',  ( -22.40074995931641055, -13.33491940220945793, 165.5209445330007725 ) ) ;
#76685=CARTESIAN_POINT ( 'NONE',  ( -21.94381615377086447, 13.26253372808103848, 167.9278110240108788 ) ) ;
#76748=CARTESIAN_POINT ( 'NONE',  ( -17.14385361876520619, 23.59649016807275856, 146.5750000027311444 ) ) ;
#76834=DIRECTION ( 'NONE',  ( -1.000000000000000000, 0.000000000000000000, 0.000000000000000000 ) ) ;
#76837=CARTESIAN_POINT ( 'NONE',  ( -26.26106931734002004, -9.140213825779254009, 167.1341548181403596 ) ) ;
#76882=CARTESIAN_POINT ( 'NONE',  ( 27.05641397906351386, -3.631740835637518927, 169.9999999999999716 ) ) ;
#76909=CARTESIAN_POINT ( 'NONE',  ( -22.44159573604009950, -16.30477369853688430, 145.0750000027311728 ) ) ;
#77048=CARTESIAN_POINT ( 'NONE',  ( 8.906447517083050158, 27.41122689804195645, 145.4000000000000057 ) ) ;
#77066=CARTESIAN_POINT ( 'NONE',  ( 21.76480897080536181, -7.725232727579773417, 173.1951875983967852 ) ) ;
#77093=EDGE_CURVE ( 'NONE', #100463, #79565, #47785, .T. ) ;
#77148=CARTESIAN_POINT ( 'NONE',  ( -21.88033147701211689, -7.974798826780787664, 169.5716465351736986 ) ) ;
#77149=ORIENTED_EDGE ( 'NONE', *, *, #176999, .F. ) ;
#77188=DIRECTION ( 'NONE',  ( 0.000000000000000000, 0.000000000000000000, 1.000000000000000000 ) ) ;
#77207=CARTESIAN_POINT ( 'NONE',  ( -26.79475375365586842, 2.428612866367529932E-14, 155.0000000000000000 ) ) ;
#77275=ORIENTED_EDGE ( 'NONE', *, *, #167369, .T. ) ;
#77314=CARTESIAN_POINT ( 'NONE',  ( 16.94467121224478134, -22.03697309902838697, 139.9999999999999432 ) ) ;
#77330=CIRCLE ( 'NONE', #90181, 26.05799246640827960 ) ;
#77340=CARTESIAN_POINT ( 'NONE',  ( 21.81399809961443381, -8.291606000631404072, 169.3279294801716048 ) ) ;
#77396=CARTESIAN_POINT ( 'NONE',  ( -8.571926809382608425, 26.38167802310805854, 144.9750000027312069 ) ) ;
#77400=CARTESIAN_POINT ( 'NONE',  ( -8.571926809382601320, -26.38167802310801591, 145.7750000027311899 ) ) ;
#77435=CARTESIAN_POINT ( 'NONE',  ( -21.51693143705271893, -10.15780255052857406, 170.5200780514254859 ) ) ;
#77453=CARTESIAN_POINT ( 'NONE',  ( 8.898068258721473001, -27.38543819252872069, 140.8656553485623704 ) ) ;
#77590=CARTESIAN_POINT ( 'NONE',  ( -18.43223033536927957, 22.10073931973474970, 139.9999999999999716 ) ) ;
#77619=CARTESIAN_POINT ( 'NONE',  ( -23.71437531004594135, -10.61261859643794558, 165.9743991446059113 ) ) ;
#77626=ORIENTED_EDGE ( 'NONE', *, *, #175018, .F. ) ;
#77680=CARTESIAN_POINT ( 'NONE',  ( -20.93662873023660254, 10.44628751056252725, 168.2749732860604013 ) ) ;
#77698=EDGE_CURVE ( 'NONE', #114568, #173841, #147383, .T. ) ;
#77717=CYLINDRICAL_SURFACE ( 'NONE', #130537, 28.79475375365586487 ) ;
#77743=CARTESIAN_POINT ( 'NONE',  ( -17.14385361876520619, 23.59649016807275856, 142.5750000027312012 ) ) ;
#77902=CARTESIAN_POINT ( 'NONE',  ( 27.73933785331498569, 2.768321779492822058E-14, 141.8750000027311842 ) ) ;
#77974=FACE_OUTER_BOUND ( 'NONE', #128601, .T. ) ;
#78026=CARTESIAN_POINT ( 'NONE',  ( -21.38418241377623374, -7.427326039334300134, 174.4773576836617224 ) ) ;
#78035=CARTESIAN_POINT ( 'NONE',  ( 23.31738231874054890, -16.94106989632523508, 144.7999999999999829 ) ) ;
#78047=CARTESIAN_POINT ( 'NONE',  ( 21.47376810972761163, -7.452933495370365868, 174.2084625793492307 ) ) ;
#78058=CARTESIAN_POINT ( 'NONE',  ( 0.000000000000000000, -5.795830589372932273, 190.0000000000000000 ) ) ;
#78076=ORIENTED_EDGE ( 'NONE', *, *, #49797, .T. ) ;
#78131=CARTESIAN_POINT ( 'NONE',  ( -21.92083080610932200, -6.374575339255695638, 171.4095429173266325 ) ) ;
#78132=ORIENTED_EDGE ( 'NONE', *, *, #77093, .F. ) ;
#78291=DIRECTION ( 'NONE',  ( 0.000000000000000000, 0.000000000000000000, 1.000000000000000000 ) ) ;
#78381=CARTESIAN_POINT ( 'NONE',  ( 27.73933785331498569, 2.768321779492822058E-14, 146.3750000027311842 ) ) ;
#78405=CARTESIAN_POINT ( 'NONE',  ( 25.77168321198462664, -6.124454116751252286, 163.0898522765300811 ) ) ;
#78575=CARTESIAN_POINT ( 'NONE',  ( 0.4100696261202915749, 28.38346208463798348, 140.0000000000000853 ) ) ;
#78666=CARTESIAN_POINT ( 'NONE',  ( -23.63516320021239636, 9.722623904421405783, 168.4908852323012809 ) ) ;
#78709=DIRECTION ( 'NONE',  ( 0.000000000000000000, 0.000000000000000000, -1.000000000000000000 ) ) ;
#78727=CARTESIAN_POINT ( 'NONE',  ( 20.02446474427094003, 11.96320450740734032, 170.0134183209139849 ) ) ;
#78732=CARTESIAN_POINT ( 'NONE',  ( 17.14385361876520264, -23.59649016807271238, 139.5750000027311444 ) ) ;
#78892=CARTESIAN_POINT ( 'NONE',  ( -27.05641397906351742, 3.631740835637567333, 169.9999999999999716 ) ) ;
#78925=AXIS2_PLACEMENT_3D ( 'NONE', #86879, #148564, #71714 ) ;
#79033=CARTESIAN_POINT ( 'NONE',  ( -23.31738231874055245, -16.94106989632524574, 140.1999999999999886 ) ) ;
#79061=CARTESIAN_POINT ( 'NONE',  ( 23.22614267028769675, 5.670187745555516301, 172.0618673401326646 ) ) ;
#79130=FACE_OUTER_BOUND ( 'NONE', #86431, .T. ) ;
#79212=CARTESIAN_POINT ( 'NONE',  ( -23.29544513554940721, -16.92513159979223403, 148.1843446569000093 ) ) ;
#79424=CARTESIAN_POINT ( 'NONE',  ( -25.85392304583074008, -7.514126903510844002, 173.7688241862487644 ) ) ;
#79565=VERTEX_POINT ( 'NONE', #5840 ) ;
#79572=CARTESIAN_POINT ( 'NONE',  ( 26.56065628307858262, 9.391201389438098346, 155.7923318601102380 ) ) ;
#79580=CARTESIAN_POINT ( 'NONE',  ( -2.996983800768426409, 28.38061290966174255, 139.9999999999999716 ) ) ;
#79644=CARTESIAN_POINT ( 'NONE',  ( 24.95432927374997334, 0.000000000000000000, 190.0000000000000000 ) ) ;
#79670=CARTESIAN_POINT ( 'NONE',  ( -24.10180676228322483, 9.559744493757339256, 166.3058469464611164 ) ) ;
#79706=EDGE_CURVE ( 'NONE', #101739, #103252, #111038, .T. ) ;
#79715=FACE_BOUND ( 'NONE', #82846, .T. ) ;
#79737=CARTESIAN_POINT ( 'NONE',  ( -27.73933785331498925, 9.013057229001089965, 140.7750000027311899 ) ) ;
#79742=ORIENTED_EDGE ( 'NONE', *, *, #104490, .F. ) ;
#79751=CARTESIAN_POINT ( 'NONE',  ( 27.96122637818066181, -7.045120623242188351, 161.2893955982186185 ) ) ;
#79767=B_SPLINE_CURVE_WITH_KNOTS ( 'NONE', 3,
 ( #153158, #138982, #94463, #170325, #460, #32812, #187507, #109641, #1457, #14659, #15655, #140971, #137997, #199681, #171324, #2459, #77314, #61146, #188487, #17642, #64141, #108647 ),
 .UNSPECIFIED., .F., .F.,
 ( 4, 2, 2, 2, 2, 2, 2, 2, 2, 2, 4 ),
 ( 0.000000000000000000, 0.005439051211804343464, 0.01087810242360868693, 0.01359762802951085953, 0.01631715363541303213, 0.02175620484721737039, 0.02719525605902171211, 0.03263430727082605037, 0.03807335848263039557, 0.04079288408853257164, 0.04351240969443474077 ),
 .UNSPECIFIED. ) ;
#79774=CARTESIAN_POINT ( 'NONE',  ( 21.54612633733962568, 7.439814990119595350, 174.3585332542395463 ) ) ;
#79934=EDGE_CURVE ( 'NONE', #148543, #147212, #131784, .T. ) ;
#80026=CARTESIAN_POINT ( 'NONE',  ( -25.12473289294612755, 7.795855283352524090, 170.9710361440363613 ) ) ;
#80047=CARTESIAN_POINT ( 'NONE',  ( 26.45594755429551626, -8.318738267476710746, 167.5492909577866101 ) ) ;
#80051=LINE ( 'NONE', #35540, #70826 ) ;
#80105=ORIENTED_EDGE ( 'NONE', *, *, #163400, .T. ) ;
#80125=CARTESIAN_POINT ( 'NONE',  ( 8.906447517083050158, 27.41122689804195645, 143.6500000054623740 ) ) ;
#80181=LINE ( 'NONE', #77207, #41189 ) ;
#80184=CARTESIAN_POINT ( 'NONE',  ( -17.79613651744294600, 24.49428055684532524, 147.9656553485623647 ) ) ;
#80204=DIRECTION ( 'NONE',  ( -0.9945218953682734009, 0.000000000000000000, -0.1045284632676528741 ) ) ;
#80211=CARTESIAN_POINT ( 'NONE',  ( -23.29544513554940721, -16.92513159979223758, 142.4656553485623647 ) ) ;
#80437=ORIENTED_EDGE ( 'NONE', *, *, #160998, .F. ) ;
#80550=ORIENTED_EDGE ( 'NONE', *, *, #99297, .T. ) ;
#80601=DIRECTION ( 'NONE',  ( 1.000000000000000000, 0.000000000000000000, -0.000000000000000000 ) ) ;
#80654=CARTESIAN_POINT ( 'NONE',  ( -24.29042230868038388, 8.936166115090465212, 166.5611006352799848 ) ) ;
#80692=DIRECTION ( 'NONE',  ( -1.000000000000000000, -0.000000000000000000, 0.000000000000000000 ) ) ;
#80714=CARTESIAN_POINT ( 'NONE',  ( 21.64434376887848899, 9.890319055725232289, 170.6724019390510421 ) ) ;
#80719=CARTESIAN_POINT ( 'NONE',  ( 17.14385361876520264, -23.59649016807271238, 141.5750000027312012 ) ) ;
#80826=ORIENTED_EDGE ( 'NONE', *, *, #199141, .T. ) ;
#80842=CARTESIAN_POINT ( 'NONE',  ( 23.64874990377914799, 15.04272038711346049, 165.8682408883346397 ) ) ;
#80948=CARTESIAN_POINT ( 'NONE',  ( 22.65770943308888263, 11.99324031494455589, 167.9410816520763206 ) ) ;
#81031=CARTESIAN_POINT ( 'NONE',  ( 25.34721418589261432, -10.09305078451928317, 170.5222919391072764 ) ) ;
#81037=FILL_AREA_STYLE_COLOUR ( '', #170318 ) ;
#81042=CARTESIAN_POINT ( 'NONE',  ( 23.88380138457669588, -7.642903512909267505, 172.4262750319489612 ) ) ;
#81048=DIRECTION ( 'NONE',  ( -0.8437662581494459468, -0.5367108174878556515, 0.000000000000000000 ) ) ;
#81088=ORIENTED_EDGE ( 'NONE', *, *, #32424, .F. ) ;
#81111=ORIENTED_EDGE ( 'NONE', *, *, #114259, .T. ) ;
#81166=CARTESIAN_POINT ( 'NONE',  ( -3.573655867282028392E-15, 12.39993551617566681, 167.9999999999999716 ) ) ;
#81227=ORIENTED_EDGE ( 'NONE', *, *, #51319, .T. ) ;
#81231=EDGE_LOOP ( 'NONE', ( #3644, #102177, #173337, #161852, #116906 ) ) ;
#81285=ORIENTED_EDGE ( 'NONE', *, *, #47103, .F. ) ;
#81344=CARTESIAN_POINT ( 'NONE',  ( -25.62086810090349687, 2.114847725256050184E-14, 167.9999999999999716 ) ) ;
#81524=ORIENTED_EDGE ( 'NONE', *, *, #137185, .F. ) ;
#81564=CARTESIAN_POINT ( 'NONE',  ( -23.71437922609632665, 10.61260870832700931, 165.9744018657351887 ) ) ;
#81602=ORIENTED_EDGE ( 'NONE', *, *, #28979, .T. ) ;
#81667=CARTESIAN_POINT ( 'NONE',  ( 19.49401214000076976, 12.39993551617566681, 164.9999999999999716 ) ) ;
#81687=CARTESIAN_POINT ( 'NONE',  ( 21.96985492114658811, 8.492568044003455441, 171.8755390570805730 ) ) ;
#81712=AXIS2_PLACEMENT_3D ( 'NONE', #24749, #134918, #119736 ) ;
#81798=FACE_OUTER_BOUND ( 'NONE', #41869, .T. ) ;
#81857=CARTESIAN_POINT ( 'NONE',  ( -8.571926809382601320, -26.38167802310801591, 139.2750000027311899 ) ) ;
#81918=DIRECTION ( 'NONE',  ( 0.000000000000000000, 0.000000000000000000, -1.000000000000000000 ) ) ;
#81985=CARTESIAN_POINT ( 'NONE',  ( -24.43795752428855650, -7.704305290315005550, 171.8420761435737916 ) ) ;
#82001=EDGE_LOOP ( 'NONE', ( #144397, #36269, #115118, #138705 ) ) ;
#82006=CARTESIAN_POINT ( 'NONE',  ( 21.94905633995417915, -8.886455535323333876, 171.4390084046505365 ) ) ;
#82030=CARTESIAN_POINT ( 'NONE',  ( -8.571926809382608425, 26.38167802310805854, 142.4750000027312069 ) ) ;
#82054=AXIS2_PLACEMENT_3D ( 'NONE', #82060, #99242, #83075 ) ;
#82060=CARTESIAN_POINT ( 'NONE',  ( 0.000000000000000000, 0.000000000000000000, 0.000000000000000000 ) ) ;
#82088=CARTESIAN_POINT ( 'NONE',  ( 27.73933785331498214, 9.013057229001095294, 142.4750000027311785 ) ) ;
#82090=CARTESIAN_POINT ( 'NONE',  ( -28.82186960331499037, 2.428612866367529932E-14, 148.2500000054623683 ) ) ;
#82091=ORIENTED_EDGE ( 'NONE', *, *, #14309, .T. ) ;
#82102=LINE ( 'NONE', #97273, #14909 ) ;
#82104=CARTESIAN_POINT ( 'NONE',  ( -17.14385361876520975, 23.59649016807275856, 149.0750000027312012 ) ) ;
#82175=DIRECTION ( 'NONE',  ( 0.000000000000000000, 0.000000000000000000, -1.000000000000000000 ) ) ;
#82184=VECTOR ( 'NONE', #150798, 1000.000000000000000 ) ;
#82231=ORIENTED_EDGE ( 'NONE', *, *, #114246, .F. ) ;
#82258=DIRECTION ( 'NONE',  ( -0.8437662581494472791, 0.5367108174878539861, 0.000000000000000000 ) ) ;
#82312=VERTEX_POINT ( 'NONE', #53260 ) ;
#82346=CARTESIAN_POINT ( 'NONE',  ( -3.573655867282028392E-15, 2.428612866367529932E-14, 150.0000000000000000 ) ) ;
#82363=( BOUNDED_CURVE ( )  B_SPLINE_CURVE ( 2, ( #172455, #17787, #141113, #125947, #77453, #49116, #139124, #601, #54091, #111770, #113742 ),
 .UNSPECIFIED., .F., .F. ) 
 B_SPLINE_CURVE_WITH_KNOTS ( ( 3, 2, 2, 2, 2, 3 ),
 ( 0.7000000000000033973, 0.7200000000000034150, 0.7400000000000034328, 0.7600000000000035616, 0.7800000000000035794, 0.8000000000000035971 ),
 .UNSPECIFIED. ) 
 CURVE ( )  GEOMETRIC_REPRESENTATION_ITEM ( )  RATIONAL_B_SPLINE_CURVE ( ( 0.9999999999999915623, 0.9510565162951619689, 1.000000000000000000, 0.9510565162951535312, 1.000000000000000000, 0.9510565162951535312, 1.000000000000000000, 0.9510565162951535312, 1.000000000000000000, 0.9510565162951448714, 1.000000000000008660 ) ) 
 REPRESENTATION_ITEM ( '' )  );
#82380=DIRECTION ( 'NONE',  ( -0.000000000000000000, -0.000000000000000000, -1.000000000000000000 ) ) ;
#82464=DIRECTION ( 'NONE',  ( 0.000000000000000000, 0.000000000000000000, -1.000000000000000000 ) ) ;
#82506=CARTESIAN_POINT ( 'NONE',  ( 24.37407968765134569, -13.84118768211351735, 165.9040744261181430 ) ) ;
#82572=CARTESIAN_POINT ( 'NONE',  ( -21.98685479826779954, 13.98560643873834408, 165.5209445330007441 ) ) ;
#82736=CARTESIAN_POINT ( 'NONE',  ( 21.38418241377623019, 7.427326039334300134, 174.4773576836617224 ) ) ;
#82755=DIRECTION ( 'NONE',  ( 0.000000000000000000, 0.000000000000000000, -1.000000000000000000 ) ) ;
#82799=DIRECTION ( 'NONE',  ( -1.000000000000000000, 0.000000000000000000, 0.000000000000000000 ) ) ;
#82846=EDGE_LOOP ( 'NONE', ( #9710, #16090, #190668, #133038 ) ) ;
#82857=CARTESIAN_POINT ( 'NONE',  ( -19.49401214000074489, -12.39993551617566503, 169.9999999999999716 ) ) ;
#83017=ADVANCED_FACE ( 'NONE', ( #8770 ), #103077, .T. ) ;
#83048=CARTESIAN_POINT ( 'NONE',  ( -22.44159573604009950, -16.30477369853688430, 143.0750000027311728 ) ) ;
#83075=DIRECTION ( 'NONE',  ( 1.000000000000000000, 0.000000000000000000, 0.000000000000000000 ) ) ;
#83105=CARTESIAN_POINT ( 'NONE',  ( 23.31738231874054890, -16.94106989632523508, 145.0500000054623513 ) ) ;
#83118=CARTESIAN_POINT ( 'NONE',  ( 22.44159573604009239, 16.30477369853692693, 146.5750000027312012 ) ) ;
#83186=CARTESIAN_POINT ( 'NONE',  ( 28.79475375365586132, 2.781246896534039337E-14, 150.0000000000000000 ) ) ;
#83191=CARTESIAN_POINT ( 'NONE',  ( -21.75836449082843060, 9.620754668593672676, 170.8405250346329467 ) ) ;
#83193=CARTESIAN_POINT ( 'NONE',  ( -17.79613651744293890, -24.49428055684528260, 142.5656553485623590 ) ) ;
#83231=CARTESIAN_POINT ( 'NONE',  ( 21.04946095171257525, 10.86023174791543866, 170.2405914574444239 ) ) ;
#83239=CIRCLE ( 'NONE', #15429, 27.91311885011353766 ) ;
#83263=AXIS2_PLACEMENT_3D ( 'NONE', #146458, #7951, #69634 ) ;
#83533=CARTESIAN_POINT ( 'NONE',  ( -28.79475375365606737, 9.355982642738961630, 147.8843446568999980 ) ) ;
#83544=CARTESIAN_POINT ( 'NONE',  ( 25.64061671795035124, 10.58440545630783269, 139.9999999999999716 ) ) ;
#83582=CARTESIAN_POINT ( 'NONE',  ( 21.98685479826779243, 13.98560643873834231, 165.5209445330007441 ) ) ;
#83632=CARTESIAN_POINT ( 'NONE',  ( 24.79447686064953160, -6.332871904612202840, 168.1804317516249512 ) ) ;
#83678=CARTESIAN_POINT ( 'NONE',  ( 22.40074995931641766, 13.33491940220945793, 165.5209445330007441 ) ) ;
#83766=CARTESIAN_POINT ( 'NONE',  ( -28.53458682541353042, -3.706052286928735562, 140.0000000000000568 ) ) ;
#83803=VECTOR ( 'NONE', #106833, 1000.000000000000114 ) ;
#83809=DIRECTION ( 'NONE',  ( -0.000000000000000000, 1.000000000000000000, -0.000000000000000000 ) ) ;
#83875=DIRECTION ( 'NONE',  ( 1.000000000000000000, 0.000000000000000000, 0.000000000000000000 ) ) ;
#83899=CARTESIAN_POINT ( 'NONE',  ( 22.54345066063599035, -5.578190839439335136, 172.9373910537578354 ) ) ;
#83933=CARTESIAN_POINT ( 'NONE',  ( 19.83802472612599743, 12.02135855755798133, 167.9999999999999716 ) ) ;
#83954=ORIENTED_EDGE ( 'NONE', *, *, #59210, .T. ) ;
#83992=ORIENTED_EDGE ( 'NONE', *, *, #141591, .F. ) ;
#83996=VERTEX_POINT ( 'NONE', #63459 ) ;
#84046=CARTESIAN_POINT ( 'NONE',  ( 22.44159573604009239, 16.30477369853692693, 144.0750000027311728 ) ) ;
#84099=CARTESIAN_POINT ( 'NONE',  ( -17.14385361876520619, 23.59649016807275856, 141.0750000027311728 ) ) ;
#84100=CARTESIAN_POINT ( 'NONE',  ( 1.993301997531345292E-15, -30.30510711980685912, 138.7500000054623683 ) ) ;
#84113=CARTESIAN_POINT ( 'NONE',  ( 27.73933785331498569, 2.768321779492822058E-14, 146.3750000027311842 ) ) ;
#84159=CARTESIAN_POINT ( 'NONE',  ( -28.79475375365585066, 2.428612866367529932E-14, 148.2656553485623760 ) ) ;
#84182=FACE_OUTER_BOUND ( 'NONE', #113390, .T. ) ;
#84225=CARTESIAN_POINT ( 'NONE',  ( 26.70292545465260048, 6.820347898102890660, 168.5277281069536741 ) ) ;
#84261=B_SPLINE_CURVE_WITH_KNOTS ( 'NONE', 3,
 ( #10453, #28619, #58927, #56955, #182290, #43770, #26625, #105434, #88268, #167119, #109400, #61891, #1214, #31576 ),
 .UNSPECIFIED., .F., .F.,
 ( 4, 2, 2, 2, 2, 2, 4 ),
 ( 0.000000000000000000, 0.05072380597786840806, 0.1014476119557368161, 0.2028952239114668876, 0.4057904478229276135, 0.6086856717343883671, 0.8115808956458491208 ),
 .UNSPECIFIED. ) ;
#84284=ORIENTED_EDGE ( 'NONE', *, *, #117196, .T. ) ;
#84305=FACE_OUTER_BOUND ( 'NONE', #174388, .T. ) ;
#84475=EDGE_CURVE ( 'NONE', #107664, #139693, #42987, .T. ) ;
#84481=ORIENTED_EDGE ( 'NONE', *, *, #171107, .T. ) ;
#84540=DIRECTION ( 'NONE',  ( -1.000000000000000000, -0.000000000000000000, 0.000000000000000000 ) ) ;
#84628=CARTESIAN_POINT ( 'NONE',  ( 23.03120525563227972, -11.22467059994892935, 168.0473679553712429 ) ) ;
#84653=VERTEX_POINT ( 'NONE', #83582 ) ;
#84730=CARTESIAN_POINT ( 'NONE',  ( 21.38418241377623019, 5.438282248597753110, 174.2683007571264113 ) ) ;
#84743=( BOUNDED_SURFACE ( )  B_SPLINE_SURFACE ( 1, 2, ( 
 ( #82090, #4268, #140802, #126619, #157969, #2291, #114438, #188320, #141794, #111464, #112455, #158949, #63973, #5264, #187340, #94298, #143782, #175131, #142786, #6264, #155976, #67944, #21444, #173149, #129597, #156978, #18475, #125643, #51778, #159957, #174144, #110464, #83105, #48811, #144781, #50796, #96283, #19462, #34624, #172146, #95294, #65947, #127619, #189319, #35616, #20438, #80125, #66946, #128608, #190301, #113438, #36598, #98254, #149792, #119461, #11296, #164971, #193306, #72968, #100277, #161956, #196323, #195313, #103291, #117452, #53783, #26465, #7260, #88108, #194313, #39609, #101268, #85099, #177148, #40619, #134637, #131621, #86114, #55780, #116455, #37609, #9290, #54780, #178143, #133620, #102289, #70956, #115459, #57791, #160958, #162958, #99271, #87115, #38620, #22451, #84100, #145779, #163978, #23452, #179151, #24464 ),
 ( #146785, #68945, #130608, #8278, #147805, #69956, #192304, #25475, #132625, #148802, #10291, #71949, #56794, #118466, #180158, #41627, #58762, #92067, #14246, #74936, #182124, #169923, #27467, #165965, #89109, #29438, #15251, #185094, #122416, #1054, #167939, #75918, #138580, #73960, #151780, #120432, #43608, #42619, #76909, #105273, #60743, #137593, #104285, #166960, #60, #61733, #136599, #91070, #152757, #28462, #197299, #199275, #150799, #59757, #184108, #153755, #108244, #31415, #45589, #93067, #30419, #168914, #12295, #121425, #90098, #154753, #16250, #13273, #107243, #198279, #77902, #123401, #135628, #46582, #183118, #44601, #139569, #62727, #106256, #181145, #2061, #35387, #157745, #18246, #125414, #113214, #170917, #109238, #32409, #172920, #158719, #128378, #65717, #144548, #111228, #19236, #81857, #17241, #95063, #63740, #187111 ) ),
 .UNSPECIFIED., .F., .F., .T. ) 
 B_SPLINE_SURFACE_WITH_KNOTS ( ( 2, 2 ),
 ( 3, 2, 2, 2, 2, 2, 2, 2, 2, 2, 2, 2, 2, 2, 2, 2, 2, 2, 2, 2, 2, 2, 2, 2, 2, 2, 2, 2, 2, 2, 2, 2, 2, 2, 2, 2, 2, 2, 2, 2, 2, 2, 2, 2, 2, 2, 2, 2, 2, 2, 3 ),
 ( 0.000000000000000000, 1.000000000000000000 ),
 ( 0.000000000000000000, 0.02000000000000000042, 0.04000000000000000083, 0.05999999999999999778, 0.08000000000000000167, 0.1000000000000000056, 0.1199999999999999956, 0.1400000000000000133, 0.1600000000000000033, 0.1799999999999999933, 0.2000000000000000111, 0.2200000000000000011, 0.2399999999999999911, 0.2600000000000000089, 0.2800000000000000266, 0.2999999999999999889, 0.3200000000000000067, 0.3400000000000000244, 0.3599999999999999867, 0.3800000000000000044, 0.4000000000000000222, 0.4199999999999999845, 0.4400000000000000022, 0.4600000000000000200, 0.4799999999999999822, 0.5000000000000000000, 0.5200000000000000178, 0.5400000000000000355, 0.5600000000000000533, 0.5799999999999999600, 0.5999999999999999778, 0.6199999999999999956, 0.6400000000000000133, 0.6600000000000000311, 0.6800000000000000488, 0.6999999999999999556, 0.7199999999999999734, 0.7399999999999999911, 0.7600000000000000089, 0.7800000000000000266, 0.8000000000000000444, 0.8199999999999999512, 0.8399999999999999689, 0.8599999999999999867, 0.8800000000000000044, 0.9000000000000000222, 0.9200000000000000400, 0.9399999999999999467, 0.9599999999999999645, 0.9799999999999999822, 1.000000000000000000 ),
 .UNSPECIFIED. ) 
 GEOMETRIC_REPRESENTATION_ITEM ( )  RATIONAL_B_SPLINE_SURFACE ( (
 ( 1.000000000000000000, 0.9510565162951535312, 1.000000000000000000, 0.9510565162951535312, 1.000000000000000000, 0.9510565162951535312, 1.000000000000000000, 0.9510565162951535312, 1.000000000000000000, 0.9510565162951535312, 1.000000000000000000, 0.9510565162951535312, 1.000000000000000000, 0.9510565162951535312, 1.000000000000000000, 0.9510565162951535312, 1.000000000000000000, 0.9510565162951535312, 1.000000000000000000, 0.9510565162951535312, 1.000000000000000000, 0.9510565162951535312, 1.000000000000000000, 0.9510565162951535312, 1.000000000000000000, 0.9510565162951535312, 1.000000000000000000, 0.9510565162951535312, 1.000000000000000000, 0.9510565162951535312, 1.000000000000000000, 0.9510565162951535312, 1.000000000000000000, 0.9510565162951535312, 1.000000000000000000, 0.9510565162951535312, 1.000000000000000000, 0.9510565162951535312, 1.000000000000000000, 0.9510565162951535312, 1.000000000000000000, 0.9510565162951535312, 1.000000000000000000, 0.9510565162951535312, 1.000000000000000000, 0.9510565162951535312, 1.000000000000000000, 0.9510565162951535312, 1.000000000000000000, 0.9510565162951535312, 1.000000000000000000, 0.9510565162951535312, 1.000000000000000000, 0.9510565162951535312, 1.000000000000000000, 0.9510565162951535312, 1.000000000000000000, 0.9510565162951535312, 1.000000000000000000, 0.9510565162951535312, 1.000000000000000000, 0.9510565162951535312, 1.000000000000000000, 0.9510565162951535312, 1.000000000000000000, 0.9510565162951535312, 1.000000000000000000, 0.9510565162951535312, 1.000000000000000000, 0.9510565162951535312, 1.000000000000000000, 0.9510565162951535312, 1.000000000000000000, 0.9510565162951535312, 1.000000000000000000, 0.9510565162951535312, 1.000000000000000000, 0.9510565162951535312, 1.000000000000000000, 0.9510565162951535312, 1.000000000000000000, 0.9510565162951535312, 1.000000000000000000, 0.9510565162951535312, 1.000000000000000000, 0.9510565162951535312, 1.000000000000000000, 0.9510565162951535312, 1.000000000000000000, 0.9510565162951535312, 1.000000000000000000, 0.9510565162951535312, 1.000000000000000000, 0.9510565162951535312, 1.000000000000000000, 0.9510565162951535312, 1.000000000000000000, 0.9510565162951535312, 1.000000000000000000, 0.9510565162951535312, 1.000000000000000000),
 ( 1.000000000000000000, 0.9510565162951535312, 1.000000000000000000, 0.9510565162951535312, 1.000000000000000000, 0.9510565162951535312, 1.000000000000000000, 0.9510565162951535312, 1.000000000000000000, 0.9510565162951535312, 1.000000000000000000, 0.9510565162951535312, 1.000000000000000000, 0.9510565162951535312, 1.000000000000000000, 0.9510565162951535312, 1.000000000000000000, 0.9510565162951535312, 1.000000000000000000, 0.9510565162951535312, 1.000000000000000000, 0.9510565162951535312, 1.000000000000000000, 0.9510565162951535312, 1.000000000000000000, 0.9510565162951535312, 1.000000000000000000, 0.9510565162951535312, 1.000000000000000000, 0.9510565162951535312, 1.000000000000000000, 0.9510565162951535312, 1.000000000000000000, 0.9510565162951535312, 1.000000000000000000, 0.9510565162951535312, 1.000000000000000000, 0.9510565162951535312, 1.000000000000000000, 0.9510565162951535312, 1.000000000000000000, 0.9510565162951535312, 1.000000000000000000, 0.9510565162951535312, 1.000000000000000000, 0.9510565162951535312, 1.000000000000000000, 0.9510565162951535312, 1.000000000000000000, 0.9510565162951535312, 1.000000000000000000, 0.9510565162951535312, 1.000000000000000000, 0.9510565162951535312, 1.000000000000000000, 0.9510565162951535312, 1.000000000000000000, 0.9510565162951535312, 1.000000000000000000, 0.9510565162951535312, 1.000000000000000000, 0.9510565162951535312, 1.000000000000000000, 0.9510565162951535312, 1.000000000000000000, 0.9510565162951535312, 1.000000000000000000, 0.9510565162951535312, 1.000000000000000000, 0.9510565162951535312, 1.000000000000000000, 0.9510565162951535312, 1.000000000000000000, 0.9510565162951535312, 1.000000000000000000, 0.9510565162951535312, 1.000000000000000000, 0.9510565162951535312, 1.000000000000000000, 0.9510565162951535312, 1.000000000000000000, 0.9510565162951535312, 1.000000000000000000, 0.9510565162951535312, 1.000000000000000000, 0.9510565162951535312, 1.000000000000000000, 0.9510565162951535312, 1.000000000000000000, 0.9510565162951535312, 1.000000000000000000, 0.9510565162951535312, 1.000000000000000000, 0.9510565162951535312, 1.000000000000000000, 0.9510565162951535312, 1.000000000000000000, 0.9510565162951535312, 1.000000000000000000, 0.9510565162951535312, 1.000000000000000000) ) ) 
 REPRESENTATION_ITEM ( '' )  SURFACE ( )  );
#84763=CARTESIAN_POINT ( 'NONE',  ( -27.66235494655239791, -7.573861383418037718, 139.9999999999999716 ) ) ;
#84832=FILL_AREA_STYLE_COLOUR ( '', #8045 ) ;
#84833=CARTESIAN_POINT ( 'NONE',  ( 25.22509938781154304, -6.326560822155840924, 165.8168946714177991 ) ) ;
#84929=CARTESIAN_POINT ( 'NONE',  ( 24.24393946303100122, 5.863316274095517144, 172.4343578713345551 ) ) ;
#84984=ADVANCED_FACE ( 'NONE', ( #53255 ), #145261, .F. ) ;
#84991=ORIENTED_EDGE ( 'NONE', *, *, #66645, .F. ) ;
#85017=CARTESIAN_POINT ( 'NONE',  ( -26.03370437638687918, 6.875205692009823011, 160.5968874236874910 ) ) ;
#85042=CARTESIAN_POINT ( 'NONE',  ( 27.73933785331498569, 2.768321779492822058E-14, 141.8750000027311842 ) ) ;
#85098=CARTESIAN_POINT ( 'NONE',  ( 8.571926809382603096, -26.38167802310801235, 141.9750000027312069 ) ) ;
#85099=CARTESIAN_POINT ( 'NONE',  ( 23.31738231874054890, -16.94106989632523508, 141.0500000054623513 ) ) ;
#85114=CARTESIAN_POINT ( 'NONE',  ( 17.14385361876520264, 23.59649016807275856, 146.6750000027311671 ) ) ;
#85169=CARTESIAN_POINT ( 'NONE',  ( -25.90238458237723052, -6.509645158105411333, 161.8463118039487085 ) ) ;
#85183=CARTESIAN_POINT ( 'NONE',  ( -23.64874990377915509, 15.04272038711346049, 165.8682408883346397 ) ) ;
#85228=CARTESIAN_POINT ( 'NONE',  ( 25.47140278216034304, 9.703455644539843661, 170.7619267275324262 ) ) ;
#85240=CARTESIAN_POINT ( 'NONE',  ( -17.14385361876520264, -23.59649016807271593, 139.6750000027311955 ) ) ;
#85345=ORIENTED_EDGE ( 'NONE', *, *, #177190, .F. ) ;
#85411=CARTESIAN_POINT ( 'NONE',  ( 25.41627434887081805, 11.65185368830120893, 166.2643564577823270 ) ) ;
#85599=CARTESIAN_POINT ( 'NONE',  ( -21.70479006154309687, -8.695791278452020379, 169.0563666577075423 ) ) ;
#85638=CARTESIAN_POINT ( 'NONE',  ( 24.10180676228338825, -9.559744493756877404, 166.3058469464611449 ) ) ;
#85776=ORIENTED_EDGE ( 'NONE', *, *, #117794, .F. ) ;
#85822=DIRECTION ( 'NONE',  ( 1.000000000000000000, 0.000000000000000000, -0.000000000000000000 ) ) ;
#86114=CARTESIAN_POINT ( 'NONE',  ( -17.81289503416611097, -24.51734667627696496, 140.5500000054623513 ) ) ;
#86117=ORIENTED_EDGE ( 'NONE', *, *, #125997, .T. ) ;
#86127=CARTESIAN_POINT ( 'NONE',  ( -27.73933785331498925, 2.428612866367529932E-14, 143.3750000027311842 ) ) ;
#86199=CARTESIAN_POINT ( 'NONE',  ( -25.11239783071224707, 12.35465959875007336, 166.1131185557730987 ) ) ;
#86239=CARTESIAN_POINT ( 'NONE',  ( 26.62494319856311975, 7.396441074661496806, 168.1134502243650104 ) ) ;
#86243=ORIENTED_EDGE ( 'NONE', *, *, #175605, .T. ) ;
#86250=CARTESIAN_POINT ( 'NONE',  ( -23.31738231874055600, 16.94106989632528837, 145.7999999999999829 ) ) ;
#86298=ORIENTED_EDGE ( 'NONE', *, *, #176519, .T. ) ;
#86306=CARTESIAN_POINT ( 'NONE',  ( 24.95432927374997334, -3.806786798636382141, 190.0000000000000000 ) ) ;
#86320=CARTESIAN_POINT ( 'NONE',  ( -28.96383432292632776, 7.816291847812730786, 151.8521076810907005 ) ) ;
#86409=CARTESIAN_POINT ( 'NONE',  ( -17.14385361876520975, 23.59649016807275856, 148.5750000027311728 ) ) ;
#86431=EDGE_LOOP ( 'NONE', ( #30629, #42750, #8497, #149741, #116878, #80437, #102238, #36723, #129348, #143098, #81524, #162174 ) ) ;
#86448=VECTOR ( 'NONE', #117671, 1000.000000000000000 ) ;
#86520=CARTESIAN_POINT ( 'NONE',  ( 26.53518950525897679, -7.921153050709833998, 167.7791411921787699 ) ) ;
#86599=CARTESIAN_POINT ( 'NONE',  ( -17.14385361876520264, -23.59649016807271593, 147.6750000027311671 ) ) ;
#86640=CARTESIAN_POINT ( 'NONE',  ( 24.85901545656367873, -5.346793810781269585, 169.1018111888375870 ) ) ;
#86742=CARTESIAN_POINT ( 'NONE',  ( 21.72193145969975703, 8.667250440200810147, 169.0624054586918987 ) ) ;
#86852=VERTEX_POINT ( 'NONE', #128851 ) ;
#86868=CARTESIAN_POINT ( 'NONE',  ( 8.898068258721473001, -27.38543819252872069, 146.5843446569000150 ) ) ;
#86879=CARTESIAN_POINT ( 'NONE',  ( -28.28060372831499336, 2.428612866367529932E-14, 149.6875000013656063 ) ) ;
#86933=CARTESIAN_POINT ( 'NONE',  ( -27.07824611089070999, -7.738748529344896987, 165.1039267699996458 ) ) ;
#86947=CARTESIAN_POINT ( 'NONE',  ( 24.50238749460113752, 2.981321037229033521, 173.3223451563238200 ) ) ;
#87040=CARTESIAN_POINT ( 'NONE',  ( -27.96813078753325144, 7.160245613316167379, 161.0900052257269692 ) ) ;
#87115=CARTESIAN_POINT ( 'NONE',  ( 23.31738231874054890, -16.94106989632523508, 139.0500000054623513 ) ) ;
#87129=CARTESIAN_POINT ( 'NONE',  ( 27.73933785331498569, 9.013057229001093518, 142.4750000027312069 ) ) ;
#87203=CARTESIAN_POINT ( 'NONE',  ( -24.54404792736085739, 12.06373989673656943, 169.8487138613016896 ) ) ;
#87254=CARTESIAN_POINT ( 'NONE',  ( 27.73933785331498925, -9.013057229001033122, 140.2750000027311330 ) ) ;
#87272=ORIENTED_EDGE ( 'NONE', *, *, #155178, .F. ) ;
#87340=CARTESIAN_POINT ( 'NONE',  ( 27.32543223595603266, -4.845308524273388429, 167.4404622590848817 ) ) ;
#87360=CARTESIAN_POINT ( 'NONE',  ( -3.573655867282028392E-15, 2.428612866367529932E-14, 164.9999999999999716 ) ) ;
#87411=CARTESIAN_POINT ( 'NONE',  ( -27.73933785331498925, 9.013057229001088189, 148.7750000027311899 ) ) ;
#87433=VERTEX_POINT ( 'NONE', #81344 ) ;
#87596=CARTESIAN_POINT ( 'NONE',  ( 22.44159573604009239, 16.30477369853692693, 148.5750000027312012 ) ) ;
#87636=CARTESIAN_POINT ( 'NONE',  ( 23.97133246043717136, -5.390759101651049434, 174.7603932261090733 ) ) ;
#87717=ADVANCED_FACE ( 'NONE', ( #35859 ), #173931, .T. ) ;
#87771=CIRCLE ( 'NONE', #123261, 23.10356920737165254 ) ;
#87825=CARTESIAN_POINT ( 'NONE',  ( -23.64874990377915509, 15.04272038711346049, 165.8682408883346397 ) ) ;
#87839=CARTESIAN_POINT ( 'NONE',  ( -3.573655867282028392E-15, 12.39993551617566681, 169.9999999999999716 ) ) ;
#87918=LINE ( 'NONE', #179968, #132615 ) ;
#88026=CARTESIAN_POINT ( 'NONE',  ( -22.94331271462295163, 0.000000000000000000, 190.0000000000000000 ) ) ;
#88085=VERTEX_POINT ( 'NONE', #80842 ) ;
#88108=CARTESIAN_POINT ( 'NONE',  ( 23.31738231874054534, 16.94106989632529192, 141.4500000054623854 ) ) ;
#88120=CARTESIAN_POINT ( 'NONE',  ( -27.05641397906351742, -3.631740835637518927, 169.9999999999999716 ) ) ;
#88149=DIRECTION ( 'NONE',  ( -0.5367108174878562066, -0.8437662581494459468, 0.000000000000000000 ) ) ;
#88243=CARTESIAN_POINT ( 'NONE',  ( 17.81289503416610742, 24.51734667627700404, 147.2999999999999545 ) ) ;
#88268=CARTESIAN_POINT ( 'NONE',  ( -23.48258780958832048, 5.709364865862125882, 171.6892424014284018 ) ) ;
#88289=EDGE_CURVE ( 'NONE', #62156, #107790, #143910, .T. ) ;
#88397=CARTESIAN_POINT ( 'NONE',  ( -17.14385361876520975, 23.59649016807275856, 146.5750000027311728 ) ) ;
#88409=CARTESIAN_POINT ( 'NONE',  ( -24.95432927374998044, -3.806786798636382585, 190.0000000000000000 ) ) ;
#88413=ORIENTED_EDGE ( 'NONE', *, *, #110272, .F. ) ;
#88416=ADVANCED_FACE ( 'NONE', ( #128335 ), #189051, .F. ) ;
#88489=ORIENTED_EDGE ( 'NONE', *, *, #160927, .T. ) ;
#88594=CARTESIAN_POINT ( 'NONE',  ( 22.44159573604009594, -16.30477369853687364, 148.1750000027311671 ) ) ;
#88636=CARTESIAN_POINT ( 'NONE',  ( -26.70292545465317247, -6.820347898097931072, 168.5277281069577953 ) ) ;
#88686=LINE ( 'NONE', #154335, #83803 ) ;
#88710=AXIS2_PLACEMENT_3D ( 'NONE', #81667, #112041, #143350 ) ;
#88742=CARTESIAN_POINT ( 'NONE',  ( 19.49401214000076621, 12.39993551617566681, 167.9999999999999716 ) ) ;
#88743=STYLED_ITEM ( 'NONE', ( #22183 ), #15828 ) ;
#88803=CARTESIAN_POINT ( 'NONE',  ( 28.79475375365586132, 2.781246896534039337E-14, 145.2656553485623760 ) ) ;
#88838=CARTESIAN_POINT ( 'NONE',  ( -19.49401214000074489, -12.39993551617566503, 169.9999999999999716 ) ) ;
#88860=CARTESIAN_POINT ( 'NONE',  ( -23.29544513554940721, -16.92513159979223403, 146.1843446569000093 ) ) ;
#88941=CARTESIAN_POINT ( 'NONE',  ( 24.22576942085165896, 7.195495839727253262, 170.3116806589316354 ) ) ;
#89005=CARTESIAN_POINT ( 'NONE',  ( -28.79475375365586842, 2.428612866367529932E-14, 142.2656553485623760 ) ) ;
#89032=CARTESIAN_POINT ( 'NONE',  ( -27.91697786073761023, 6.847065636290214918, 161.8035115693297712 ) ) ;
#89109=CARTESIAN_POINT ( 'NONE',  ( -8.571926809382608425, 26.38167802310805854, 146.4750000027311785 ) ) ;
#89176=FACE_OUTER_BOUND ( 'NONE', #107455, .T. ) ;
#89232=CARTESIAN_POINT ( 'NONE',  ( 26.26139018963107574, 3.005588016160658071, 174.9127113745526572 ) ) ;
#89247=CARTESIAN_POINT ( 'NONE',  ( -17.81289503416611097, -24.51734667627696496, 148.2999999999999545 ) ) ;
#89262=CARTESIAN_POINT ( 'NONE',  ( 23.35043118190389677, -14.19381810411683809, 169.8796877288295093 ) ) ;
#89266=( BOUNDED_CURVE ( )  B_SPLINE_CURVE ( 2, ( #186859, #167692, #75662, #47334, #94810, #90823, #1806, #171663, #60488, #2802, #122163 ),
 .UNSPECIFIED., .F., .F. ) 
 B_SPLINE_CURVE_WITH_KNOTS ( ( 3, 2, 2, 2, 2, 3 ),
 ( 0.5000000000000004441, 0.5200000000000004619, 0.5400000000000004796, 0.5600000000000006084, 0.5800000000000006262, 0.6000000000000005329 ),
 .UNSPECIFIED. ) 
 CURVE ( )  GEOMETRIC_REPRESENTATION_ITEM ( )  RATIONAL_B_SPLINE_CURVE ( ( 0.9999999999999988898, 0.9510565162951546414, 1.000000000000000000, 0.9510565162951535312, 1.000000000000000000, 0.9510565162951535312, 1.000000000000000000, 0.9510565162951535312, 1.000000000000000000, 0.9510565162951521989, 1.000000000000001332 ) ) 
 REPRESENTATION_ITEM ( '' )  );
#89388=CARTESIAN_POINT ( 'NONE',  ( -20.96339774546121504, -10.39907118706507561, 168.2889211417202944 ) ) ;
#89401=CARTESIAN_POINT ( 'NONE',  ( 27.73933785331498569, 2.768321779492822058E-14, 147.8750000027311842 ) ) ;
#89414=CARTESIAN_POINT ( 'NONE',  ( 28.79475375365586132, 2.781246896534039337E-14, 147.2656553485624045 ) ) ;
#89522=EDGE_CURVE ( 'NONE', #100170, #126623, #158273, .T. ) ;
#89532=AXIS2_PLACEMENT_3D ( 'NONE', #27113, #165614, #39263 ) ;
#89594=CARTESIAN_POINT ( 'NONE',  ( -8.571926809382601320, -26.38167802310801591, 141.7750000027311899 ) ) ;
#89633=CARTESIAN_POINT ( 'NONE',  ( -26.38458505201405657, -8.641005086744426578, 167.3773361139123779 ) ) ;
#89653=ADVANCED_FACE ( 'NONE', ( #147104, #8589 ), #73274, .F. ) ;
#89708=ORIENTED_EDGE ( 'NONE', *, *, #155738, .F. ) ;
#89811=EDGE_CURVE ( 'NONE', #126623, #10845, #76266, .T. ) ;
#89838=CARTESIAN_POINT ( 'NONE',  ( -21.16473053983486352, -10.71450305990368790, 170.2845851188454560 ) ) ;
#89860=CARTESIAN_POINT ( 'NONE',  ( 1.988064558232696151E-15, -30.27659582821216588, 146.4843446569000207 ) ) ;
#89941=CARTESIAN_POINT ( 'NONE',  ( -27.73933785331498925, 9.013057229001089965, 148.7750000027311899 ) ) ;
#90049=VERTEX_POINT ( 'NONE', #89414 ) ;
#90098=CARTESIAN_POINT ( 'NONE',  ( -8.571926809382608425, 26.38167802310805854, 142.4750000027312069 ) ) ;
#90143=CARTESIAN_POINT ( 'NONE',  ( -24.95432927374998755, 4.974562764236792667, 189.9999999999999716 ) ) ;
#90176=CARTESIAN_POINT ( 'NONE',  ( -26.45763050569055252, 3.219288925403916313, 173.6696415116524861 ) ) ;
#90181=AXIS2_PLACEMENT_3D ( 'NONE', #139386, #95874, #108050 ) ;
#90221=ORIENTED_EDGE ( 'NONE', *, *, #66504, .T. ) ;
#90233=CARTESIAN_POINT ( 'NONE',  ( 28.82186960331498327, 9.364793116373570925, 143.0999999999999659 ) ) ;
#90330=CARTESIAN_POINT ( 'NONE',  ( -21.97054992548789087, -7.027819292989581967, 170.5066066589220100 ) ) ;
#90523=LINE ( 'NONE', #152205, #72064 ) ;
#90578=CARTESIAN_POINT ( 'NONE',  ( -8.571926809382601320, -26.38167802310801591, 145.7750000027311899 ) ) ;
#90582=CARTESIAN_POINT ( 'NONE',  ( 27.73933785331498214, 9.013057229001095294, 144.4750000027311501 ) ) ;
#90618=CARTESIAN_POINT ( 'NONE',  ( -26.73207562759412070, -6.543912086054805677, 168.7462576975848378 ) ) ;
#90777=CARTESIAN_POINT ( 'NONE',  ( -23.29544513554940721, -16.92513159979223758, 144.4656553485623647 ) ) ;
#90823=CARTESIAN_POINT ( 'NONE',  ( -5.427562675786936573E-15, 30.27659582821221207, 145.4843446568999639 ) ) ;
#90878=ADVANCED_FACE ( 'NONE', ( #120732 ), #186407, .F. ) ;
#90886=CARTESIAN_POINT ( 'NONE',  ( -8.898068258721467672, -27.38543819252872069, 142.3843446568999980 ) ) ;
#90910=CARTESIAN_POINT ( 'NONE',  ( -27.73933785331498925, 2.428612866367529932E-14, 144.8750000027311842 ) ) ;
#91070=CARTESIAN_POINT ( 'NONE',  ( 17.14385361876520264, 23.59649016807275856, 144.1750000027311671 ) ) ;
#91110=CARTESIAN_POINT ( 'NONE',  ( 19.49401214000073068, -12.39993551617567391, 164.9999999999999716 ) ) ;
#91118=DIRECTION ( 'NONE',  ( -0.8437662581494473901, -0.5367108174878535420, 0.000000000000000000 ) ) ;
#91150=CARTESIAN_POINT ( 'NONE',  ( -21.47376810973062433, 7.452933495370294814, 174.2084625793499981 ) ) ;
#91203=CARTESIAN_POINT ( 'NONE',  ( 8.906447517083057264, -27.41122689804191026, 142.5999999999999943 ) ) ;
#91299=CARTESIAN_POINT ( 'NONE',  ( -24.81886791266594017, -6.075537473407860212, 168.3989613422462241 ) ) ;
#91300=ORIENTED_EDGE ( 'NONE', *, *, #5739, .F. ) ;
#91301=ORIENTED_EDGE ( 'NONE', *, *, #192849, .F. ) ;
#91553=CARTESIAN_POINT ( 'NONE',  ( -27.73933785331498925, 9.013057229001089965, 145.2750000027311899 ) ) ;
#91557=CARTESIAN_POINT ( 'NONE',  ( 1.784210473542230573E-15, -29.16686587814331588, 147.8750000027311273 ) ) ;
#91593=CARTESIAN_POINT ( 'NONE',  ( -26.78465914369777678, -5.761000505272561689, 169.4491075441772807 ) ) ;
#91714=CARTESIAN_POINT ( 'NONE',  ( -28.79475375365586842, 2.428612866367529932E-14, 144.2656553485623760 ) ) ;
#91729=EDGE_LOOP ( 'NONE', ( #72105, #199161, #73397, #13502, #7240 ) ) ;
#91794=CARTESIAN_POINT ( 'NONE',  ( -21.76481224609945642, -7.725237430229303648, 173.1951747752679580 ) ) ;
#91803=ORIENTED_EDGE ( 'NONE', *, *, #51319, .F. ) ;
#91852=CIRCLE ( 'NONE', #182249, 2.999999999999998668 ) ;
#91898=CARTESIAN_POINT ( 'NONE',  ( -27.73933785331498925, 9.013057229001089965, 142.7750000027311899 ) ) ;
#91903=ORIENTED_EDGE ( 'NONE', *, *, #36961, .T. ) ;
#91937=CARTESIAN_POINT ( 'NONE',  ( -27.32543223595607884, -4.845308524273512774, 167.4404622590845690 ) ) ;
#91987=CARTESIAN_POINT ( 'NONE',  ( -24.99788752995424446, -12.60079600866962579, 166.0698618172138197 ) ) ;
#92009=EDGE_CURVE ( 'NONE', #162114, #177366, #180830, .T. ) ;
#92020=VECTOR ( 'NONE', #186383, 1000.000000000000000 ) ;
#92067=CARTESIAN_POINT ( 'NONE',  ( -17.14385361876520264, -23.59649016807271593, 147.1750000027311671 ) ) ;
#92103=CARTESIAN_POINT ( 'NONE',  ( -17.79613651744293890, -24.49428055684527550, 140.2843446568999468 ) ) ;
#92116=EDGE_CURVE ( 'NONE', #139247, #122599, #87918, .T. ) ;
#92149=CARTESIAN_POINT ( 'NONE',  ( -26.36463166569313188, 3.076743934663749069, 174.2851114983683942 ) ) ;
#92210=CARTESIAN_POINT ( 'NONE',  ( 23.31738231874054534, 16.94106989632529192, 143.1999999999999886 ) ) ;
#92222=CARTESIAN_POINT ( 'NONE',  ( 26.79475375365586132, 2.756753960551091991E-14, 155.0000000000000000 ) ) ;
#92282=ADVANCED_FACE ( 'NONE', ( #58582, #79715 ), #123217, .F. ) ;
#92311=CARTESIAN_POINT ( 'NONE',  ( -24.79447686064995438, -6.332871904607631386, 168.1804317516292997 ) ) ;
#92313=EDGE_LOOP ( 'NONE', ( #37743, #59971 ) ) ;
#92317=ORIENTED_EDGE ( 'NONE', *, *, #177190, .T. ) ;
#92558=CARTESIAN_POINT ( 'NONE',  ( 1.784210473542230573E-15, -29.16686587814331588, 145.8750000027311273 ) ) ;
#92562=CARTESIAN_POINT ( 'NONE',  ( 27.73933785331498569, 2.768321779492822058E-14, 144.3750000027311842 ) ) ;
#92623=ORIENTED_EDGE ( 'NONE', *, *, #177902, .F. ) ;
#92749=CARTESIAN_POINT ( 'NONE',  ( 13.33220713530183765, 24.76230349490602833, 140.0000000000000853 ) ) ;
#92840=CARTESIAN_POINT ( 'NONE',  ( -24.85901545656372491, 5.346793810781125700, 169.1018111888375870 ) ) ;
#92903=CARTESIAN_POINT ( 'NONE',  ( 8.571926809382597767, 26.38167802310806209, 144.2750000027311899 ) ) ;
#92953=ORIENTED_EDGE ( 'NONE', *, *, #30184, .F. ) ;
#93038=( LENGTH_UNIT ( ) NAMED_UNIT ( * ) SI_UNIT ( .MILLI., .METRE. ) );
#93066=EDGE_CURVE ( 'NONE', #146461, #84653, #77330, .T. ) ;
#93067=CARTESIAN_POINT ( 'NONE',  ( -27.73933785331498925, -9.013057229001049109, 142.9750000027312069 ) ) ;
#93076=CARTESIAN_POINT ( 'NONE',  ( 22.24685556490046068, -12.75834802357495157, 167.9013491530738520 ) ) ;
#93102=CARTESIAN_POINT ( 'NONE',  ( 17.79613651744294245, -24.49428055684527195, 140.6843446568999809 ) ) ;
#93196=CARTESIAN_POINT ( 'NONE',  ( -22.19348515620997375, -7.491027558428858590, 173.8712782147084681 ) ) ;
#93205=CARTESIAN_POINT ( 'NONE',  ( 23.31738231874054534, 16.94106989632529192, 141.1999999999999886 ) ) ;
#93217=CARTESIAN_POINT ( 'NONE',  ( 21.81230582904510840, -7.807068725607987147, 172.9985625539908085 ) ) ;
#93221=CARTESIAN_POINT ( 'NONE',  ( 17.79613651744293534, 24.49428055684532524, 143.5656553485623590 ) ) ;
#93223=CARTESIAN_POINT ( 'NONE',  ( 20.74358237093906254, -11.24271120488110043, 170.1279846108370180 ) ) ;
#93255=DIRECTION ( 'NONE',  ( 0.000000000000000000, 0.000000000000000000, 1.000000000000000000 ) ) ;
#93307=VERTEX_POINT ( 'NONE', #8860 ) ;
#93397=EDGE_CURVE ( 'NONE', #84653, #148762, #26158, .T. ) ;
#93426=EDGE_LOOP ( 'NONE', ( #103294, #191502, #120812, #75954 ) ) ;
#93524=EDGE_LOOP ( 'NONE', ( #147843, #163476, #56286, #143145, #197889, #104178, #91903, #82091, #172330, #172649, #136492, #146285 ) ) ;
#93557=CARTESIAN_POINT ( 'NONE',  ( -8.571926809382608425, 26.38167802310805854, 142.9750000027312069 ) ) ;
#93558=DIRECTION ( 'NONE',  ( 0.000000000000000000, 0.000000000000000000, -1.000000000000000000 ) ) ;
#93587=CARTESIAN_POINT ( 'NONE',  ( -3.573655867282028392E-15, 2.428612866367529932E-14, 167.9999999999999716 ) ) ;
#93592=CARTESIAN_POINT ( 'NONE',  ( -26.61723430050314221, -3.645106422947788083, 172.4622069319862305 ) ) ;
#93751=CARTESIAN_POINT ( 'NONE',  ( -17.53359108020402957, 22.79239813733060416, 139.9999999999999716 ) ) ;
#93840=CARTESIAN_POINT ( 'NONE',  ( -20.56371838171435584, 11.04494471775268671, 168.1294998094271023 ) ) ;
#93905=CARTESIAN_POINT ( 'NONE',  ( 27.73933785331498214, 9.013057229001095294, 141.9750000027311501 ) ) ;
#94032=EDGE_CURVE ( 'NONE', #46062, #126623, #88686, .T. ) ;
#94191=CARTESIAN_POINT ( 'NONE',  ( -22.03292204642282570, -7.478118144893485919, 173.9941030799742805 ) ) ;
#94200=CARTESIAN_POINT ( 'NONE',  ( -8.906447517083053711, -27.41122689804191026, 144.4000000000000057 ) ) ;
#94214=CARTESIAN_POINT ( 'NONE',  ( 24.42783677680755972, -12.30119602009776969, 169.8172178118632587 ) ) ;
#94227=CARTESIAN_POINT ( 'NONE',  ( 23.84755066337006113, 5.771293611162917614, 171.0999092862842019 ) ) ;
#94268=CARTESIAN_POINT ( 'NONE',  ( -25.63014048727048433, 6.600871414792726100, 163.2070037194167185 ) ) ;
#94298=CARTESIAN_POINT ( 'NONE',  ( 1.993301997531345292E-15, -30.30510711980685912, 146.7500000054623683 ) ) ;
#94315=CARTESIAN_POINT ( 'NONE',  ( -27.73933785331498925, 2.428612866367529932E-14, 147.3750000027311842 ) ) ;
#94384=CYLINDRICAL_SURFACE ( 'NONE', #39809, 28.79475375365586487 ) ;
#94412=ORIENTED_EDGE ( 'NONE', *, *, #35307, .T. ) ;
#94426=ORIENTED_EDGE ( 'NONE', *, *, #75553, .T. ) ;
#94463=CARTESIAN_POINT ( 'NONE',  ( 26.85917411135797295, 7.165250986577666126, 139.9999999999999716 ) ) ;
#94498=CARTESIAN_POINT ( 'NONE',  ( -19.49401214000074489, -12.39993551617566325, 164.9999999999999716 ) ) ;
#94558=CARTESIAN_POINT ( 'NONE',  ( -3.573655867282028392E-15, 2.428612866367529932E-14, 150.0000000000000000 ) ) ;
#94617=ORIENTED_EDGE ( 'NONE', *, *, #17982, .F. ) ;
#94744=CARTESIAN_POINT ( 'NONE',  ( -8.492802586333358050, 27.26921223548736961, 140.0000000000000000 ) ) ;
#94804=ORIENTED_EDGE ( 'NONE', *, *, #89811, .F. ) ;
#94810=CARTESIAN_POINT ( 'NONE',  ( 8.898068258721464119, 27.38543819252877398, 145.3843446568999980 ) ) ;
#94837=CARTESIAN_POINT ( 'NONE',  ( -23.75112013235324682, 10.51683317207909063, 166.0021274478078226 ) ) ;
#94903=CARTESIAN_POINT ( 'NONE',  ( -27.73933785331498925, 9.013057229001089965, 149.2750000027311330 ) ) ;
#95063=CARTESIAN_POINT ( 'NONE',  ( -22.44159573604009950, -16.30477369853688430, 139.0750000027311728 ) ) ;
#95098=CARTESIAN_POINT ( 'NONE',  ( 21.50819313649865805, -5.452397343345025682, 174.1340046013950200 ) ) ;
#95191=CARTESIAN_POINT ( 'NONE',  ( -26.25049742697155253, 7.664248127782741449, 169.1476266185236454 ) ) ;
#95214=CARTESIAN_POINT ( 'NONE',  ( 24.54404792736082186, -12.06373989673630653, 169.8487138613017180 ) ) ;
#95231=CARTESIAN_POINT ( 'NONE',  ( -19.49401214000074489, -12.39993551617566148, 164.9999999999999716 ) ) ;
#95294=CARTESIAN_POINT ( 'NONE',  ( -28.82186960331499037, 2.428612866367529932E-14, 144.2500000054623683 ) ) ;
#95295=ORIENTED_EDGE ( 'NONE', *, *, #159341, .T. ) ;
#95307=CARTESIAN_POINT ( 'NONE',  ( -8.571926809382608425, 26.38167802310805854, 146.9750000027311785 ) ) ;
#95384=PRODUCT ( 'tip', 'tip', '', ( #114950 ) ) ;
#95417=ORIENTED_EDGE ( 'NONE', *, *, #171007, .F. ) ;
#95658=VERTEX_POINT ( 'NONE', #148675 ) ;
#95719=AXIS2_PLACEMENT_3D ( 'NONE', #1014, #27425, #122378 ) ;
#95738=CARTESIAN_POINT ( 'NONE',  ( 4.920875869067829811, 27.88293468337690229, 139.9999999999999147 ) ) ;
#95830=CARTESIAN_POINT ( 'NONE',  ( -24.22576942085221674, 7.195495839727391818, 170.3116806589316354 ) ) ;
#95871=CARTESIAN_POINT ( 'NONE',  ( 25.64061671795035124, 10.58440545630783269, 139.9999999999999716 ) ) ;
#95874=DIRECTION ( 'NONE',  ( -0.000000000000000000, -0.000000000000000000, -1.000000000000000000 ) ) ;
#95896=CARTESIAN_POINT ( 'NONE',  ( -8.571926809382601320, -26.38167802310801591, 139.2750000027311899 ) ) ;
#95933=DIRECTION ( 'NONE',  ( -0.1039620511844979445, 0.1039620511844979445, -0.9891328443778539814 ) ) ;
#96073=B_SPLINE_CURVE_WITH_KNOTS ( 'NONE', 3,
 ( #51709, #20369, #111394, #66874, #81042, #126552, #175063, #36529 ),
 .UNSPECIFIED., .F., .F.,
 ( 4, 2, 2, 4 ),
 ( -1.451984513606386853E-05, 0.002415095736453700456, 0.003629903527248606616, 0.004844711318043512342 ),
 .UNSPECIFIED. ) ;
#96121=CARTESIAN_POINT ( 'NONE',  ( 21.84611564451295962, 8.148379233837022895, 169.4346228884802485 ) ) ;
#96204=CARTESIAN_POINT ( 'NONE',  ( 26.78465914369787626, -5.761000505272217076, 169.4491075441770818 ) ) ;
#96283=CARTESIAN_POINT ( 'NONE',  ( -8.906447517083053711, -27.41122689804191026, 144.6500000054623740 ) ) ;
#96445=CARTESIAN_POINT ( 'NONE',  ( -23.29544513554940721, -16.92513159979223403, 144.1843446569000093 ) ) ;
#96554=CARTESIAN_POINT ( 'NONE',  ( 25.25560589046783022, -4.310829775027113620, 167.9999999999999716 ) ) ;
#96674=CYLINDRICAL_SURFACE ( 'NONE', #12018, 26.79475375365586487 ) ;
#96703=EDGE_LOOP ( 'NONE', ( #129749, #90221, #4018, #97018 ) ) ;
#96720=CARTESIAN_POINT ( 'NONE',  ( 19.57369961329614227, 19.99890699435813701, 140.0000000000000000 ) ) ;
#96803=B_SPLINE_CURVE_WITH_KNOTS ( 'NONE', 3,
 ( #177088, #53724, #9229, #100216, #176079, #143722, #131559, #5202, #38559, #97203, #37548, #20379 ),
 .UNSPECIFIED., .F., .F.,
 ( 4, 2, 2, 2, 2, 4 ),
 ( -0.003994749848159029684, -0.003130422923337863959, -0.002266095998516698233, -0.0005374421488743676492, 0.001191211700767963802, 0.002919865550410294386 ),
 .UNSPECIFIED. ) ;
#96811=CARTESIAN_POINT ( 'NONE',  ( -21.81230582904512261, 5.969922009378191063, 172.1979875755924922 ) ) ;
#96855=CARTESIAN_POINT ( 'NONE',  ( 24.66672740160585064, 7.254147403784513060, 167.4978451254145284 ) ) ;
#96875=CARTESIAN_POINT ( 'NONE',  ( 8.571926809382597767, 26.38167802310806209, 142.2750000027311899 ) ) ;
#96890=CARTESIAN_POINT ( 'NONE',  ( 27.94119071623654094, -7.398115196983436448, 160.8979257793636464 ) ) ;
#96931=CARTESIAN_POINT ( 'NONE',  ( -28.79475375365586842, 2.428612866367529932E-14, 139.9999999999999716 ) ) ;
#97010=FILL_AREA_STYLE ('',( #84832 ) ) ;
#97018=ORIENTED_EDGE ( 'NONE', *, *, #24747, .T. ) ;
#97183=CARTESIAN_POINT ( 'NONE',  ( 25.41223161463580027, -11.66315983254895627, 166.2610598689585117 ) ) ;
#97203=CARTESIAN_POINT ( 'NONE',  ( -22.15208335914311988, -5.528296758471276107, 173.4118699040215006 ) ) ;
#97207=CARTESIAN_POINT ( 'NONE',  ( -22.44159573604010305, 16.30477369853692338, 140.6750000027311671 ) ) ;
#97260=CARTESIAN_POINT ( 'NONE',  ( -8.571926809382601320, -26.38167802310801591, 147.7750000027311899 ) ) ;
#97273=CARTESIAN_POINT ( 'NONE',  ( -28.79475375365586842, 2.428612866367529932E-14, 155.0000000000000000 ) ) ;
#97343=CARTESIAN_POINT ( 'NONE',  ( 27.19095269391953806, -8.032454009542492557, 149.5864051666458181 ) ) ;
#97702=CARTESIAN_POINT ( 'NONE',  ( 21.79132363338460721, 17.42213977941835168, 139.9999999999999432 ) ) ;
#97728=CARTESIAN_POINT ( 'NONE',  ( -23.42531737588081242, 11.30614151570994430, 165.8025732123264788 ) ) ;
#97731=EDGE_CURVE ( 'NONE', #31087, #25364, #24085, .T. ) ;
#97740=CARTESIAN_POINT ( 'NONE',  ( 24.93942350307308686, 7.769968609432599926, 171.2173313942149946 ) ) ;
#97751=CARTESIAN_POINT ( 'NONE',  ( -21.94381615377314176, -13.26253372808251108, 167.9278110240112767 ) ) ;
#97767=ORIENTED_EDGE ( 'NONE', *, *, #93397, .T. ) ;
#97887=DIRECTION ( 'NONE',  ( -0.000000000000000000, 1.000000000000000000, -0.000000000000000000 ) ) ;
#97966=LINE ( 'NONE', #37318, #58162 ) ;
#98019=VECTOR ( 'NONE', #93558, 1000.000000000000000 ) ;
#98032=DIRECTION ( 'NONE',  ( 0.1736481776669307198, 0.000000000000000000, -0.9848077530122080203 ) ) ;
#98054=CARTESIAN_POINT ( 'NONE',  ( 22.32889156691206267, -5.550768075871988394, 173.1969276168243255 ) ) ;
#98086=CARTESIAN_POINT ( 'NONE',  ( 21.04946095171257525, 10.24435024061200572, 168.3368280404219774 ) ) ;
#98254=CARTESIAN_POINT ( 'NONE',  ( 23.31738231874054890, -16.94106989632523508, 143.0500000054623513 ) ) ;
#98268=CARTESIAN_POINT ( 'NONE',  ( -27.73933785331498925, 9.013057229001088189, 141.2750000027311899 ) ) ;
#98318=CARTESIAN_POINT ( 'NONE',  ( 8.898068258721465895, 27.38543819252877398, 147.6656553485623817 ) ) ;
#98387=FACE_OUTER_BOUND ( 'NONE', #91729, .T. ) ;
#98400=ORIENTED_EDGE ( 'NONE', *, *, #103264, .T. ) ;
#98427=DIRECTION ( 'NONE',  ( 0.5367108174878537641, 0.8437662581494472791, -0.000000000000000000 ) ) ;
#98490=CARTESIAN_POINT ( 'NONE',  ( -26.53518950525900166, 7.921153050709826893, 167.7791411921787699 ) ) ;
#98711=CARTESIAN_POINT ( 'NONE',  ( 27.95311704540609199, 7.352561457294874536, 160.8984504615112314 ) ) ;
#98738=CARTESIAN_POINT ( 'NONE',  ( -24.20534277172201598, 9.236732224056884988, 166.4300944521384906 ) ) ;
#98758=CARTESIAN_POINT ( 'NONE',  ( -23.03120525563285170, -11.22467059994836269, 168.0473679553712714 ) ) ;
#98796=CARTESIAN_POINT ( 'NONE',  ( 22.65770943308940488, -11.99324031494510479, 167.9410816520762921 ) ) ;
#98878=CARTESIAN_POINT ( 'NONE',  ( 27.89903062892809871, -7.496893268503402652, 160.9845644947723429 ) ) ;
#98920=FACE_OUTER_BOUND ( 'NONE', #151783, .T. ) ;
#99044=DIRECTION ( 'NONE',  ( 0.000000000000000000, 0.000000000000000000, 1.000000000000000000 ) ) ;
#99048=EDGE_CURVE ( 'NONE', #11685, #100170, #158915, .T. ) ;
#99088=CARTESIAN_POINT ( 'NONE',  ( -27.94130797166088698, -7.397772140681734498, 160.8977822374860125 ) ) ;
#99102=CARTESIAN_POINT ( 'NONE',  ( 20.14845677604831664, 11.63499142542225329, 168.0304984204095149 ) ) ;
#99201=CARTESIAN_POINT ( 'NONE',  ( 21.38418241377623019, -7.427326039334300134, 174.4773576836617224 ) ) ;
#99215=CARTESIAN_POINT ( 'NONE',  ( 17.14385361876520264, -23.59649016807270883, 143.5750000027311728 ) ) ;
#99242=DIRECTION ( 'NONE',  ( 0.000000000000000000, 0.000000000000000000, 1.000000000000000000 ) ) ;
#99270=CARTESIAN_POINT ( 'NONE',  ( 27.73933785331498569, 2.768321779492822058E-14, 142.3750000027311842 ) ) ;
#99271=CARTESIAN_POINT ( 'NONE',  ( 28.82186960331499392, -9.364793116373510529, 139.1500000054623456 ) ) ;
#99284=CARTESIAN_POINT ( 'NONE',  ( -22.44159573604009950, -16.30477369853688430, 143.5750000027311728 ) ) ;
#99297=EDGE_CURVE ( 'NONE', #84653, #172658, #103327, .T. ) ;
#99311=CARTESIAN_POINT ( 'NONE',  ( -3.573655867282028392E-15, 2.428612866367529932E-14, 164.9999999999999716 ) ) ;
#99335=CARTESIAN_POINT ( 'NONE',  ( -28.79475375365585066, 2.428612866367529932E-14, 148.2656553485623760 ) ) ;
#99358=CARTESIAN_POINT ( 'NONE',  ( -21.96844466259092243, 8.667631922777363940, 171.6690673070886533 ) ) ;
#99400=CARTESIAN_POINT ( 'NONE',  ( 21.75836449082842705, 9.620754668593672676, 170.8405250346329467 ) ) ;
#99447=DIRECTION ( 'NONE',  ( 0.000000000000000000, 0.000000000000000000, 1.000000000000000000 ) ) ;
#99500=CARTESIAN_POINT ( 'NONE',  ( -24.99734946672227665, 12.60193342193095667, 166.0696721667195845 ) ) ;
#99562=EDGE_CURVE ( 'NONE', #31966, #122086, #62775, .T. ) ;
#99644=DIRECTION ( 'NONE',  ( -1.000000000000000000, 0.000000000000000000, 0.000000000000000000 ) ) ;
#99658=ORIENTED_EDGE ( 'NONE', *, *, #16394, .T. ) ;
#99682=CARTESIAN_POINT ( 'NONE',  ( 25.28116846732000766, -11.97242897402594686, 166.1912472719372147 ) ) ;
#99718=CARTESIAN_POINT ( 'NONE',  ( 27.93407901761402456, 7.419329114306494333, 160.9060561961931057 ) ) ;
#99766=CARTESIAN_POINT ( 'NONE',  ( -20.69372460268612457, -10.84650605405325940, 168.1714143675833100 ) ) ;
#99805=CARTESIAN_POINT ( 'NONE',  ( 21.97054992548899222, -7.027819292989583744, 170.5066066589220100 ) ) ;
#99886=CARTESIAN_POINT ( 'NONE',  ( 27.86147134968521755, -7.555459793078237674, 161.1037931155416345 ) ) ;
#99992=CARTESIAN_POINT ( 'NONE',  ( 27.60098488412425155, 5.861468761071320976, 164.8187539380863313 ) ) ;
#100007=CARTESIAN_POINT ( 'NONE',  ( 28.79475375365586132, 2.781246896534039337E-14, 142.9843446568999639 ) ) ;
#100093=DIRECTION ( 'NONE',  ( 0.000000000000000000, 0.000000000000000000, 1.000000000000000000 ) ) ;
#100106=CARTESIAN_POINT ( 'NONE',  ( 21.73861122199407347, 5.803778330637469729, 172.6157762304496828 ) ) ;
#100170=VERTEX_POINT ( 'NONE', #172965 ) ;
#100216=CARTESIAN_POINT ( 'NONE',  ( -24.55187747166650425, -5.935858836270472061, 169.5341757581197726 ) ) ;
#100220=CARTESIAN_POINT ( 'NONE',  ( 1.784210473542230573E-15, -29.16686587814331588, 141.3750000027311557 ) ) ;
#100255=ORIENTED_EDGE ( 'NONE', *, *, #89811, .T. ) ;
#100277=CARTESIAN_POINT ( 'NONE',  ( -28.82186960331499392, -9.364793116373526516, 142.3500000054623342 ) ) ;
#100291=CARTESIAN_POINT ( 'NONE',  ( -8.571926809382601320, -26.38167802310801591, 141.7750000027311899 ) ) ;
#100362=CARTESIAN_POINT ( 'NONE',  ( -26.13941622279051913, 9.616497135380347672, 166.9083969906205311 ) ) ;
#100405=CARTESIAN_POINT ( 'NONE',  ( 24.44405923433096461, 13.71792739260091132, 165.9118100595185297 ) ) ;
#100416=CARTESIAN_POINT ( 'NONE',  ( -17.81289503416611808, 24.51734667627700404, 147.6999999999999886 ) ) ;
#100463=VERTEX_POINT ( 'NONE', #21497 ) ;
#100581=DIRECTION ( 'NONE',  ( 1.000000000000000000, 0.000000000000000000, -0.000000000000000000 ) ) ;
#100641=ORIENTED_EDGE ( 'NONE', *, *, #59210, .F. ) ;
#100741=CARTESIAN_POINT ( 'NONE',  ( -24.60782808046178616, 7.576750539519846228, 167.2921137806584113 ) ) ;
#100756=CARTESIAN_POINT ( 'NONE',  ( -27.73933785331498925, 2.428612866367529932E-14, 149.3750000027311842 ) ) ;
#100762=CARTESIAN_POINT ( 'NONE',  ( -24.10180676228339536, -9.559744493756875627, 166.3058469464611449 ) ) ;
#100797=CARTESIAN_POINT ( 'NONE',  ( 24.73536985823981027, -3.645104810711987664, 171.5180696409406096 ) ) ;
#100839=ADVANCED_FACE ( 'NONE', ( #189370 ), #16196, .T. ) ;
#100845=CARTESIAN_POINT ( 'NONE',  ( 21.98685479826779243, 13.98560643873834231, 165.5209445330007441 ) ) ;
#100901=CARTESIAN_POINT ( 'NONE',  ( 20.61165082012733762, 10.97245752705834221, 168.1443239908791156 ) ) ;
#100937=CARTESIAN_POINT ( 'NONE',  ( -20.84945647820398662, 10.59429869652067069, 168.2340845703681680 ) ) ;
#100981=PLANE ( 'NONE',  #38801 ) ;
#101144=CARTESIAN_POINT ( 'NONE',  ( 22.96528548301342809, 5.795830589372932273, 190.0000000000000000 ) ) ;
#101186=CARTESIAN_POINT ( 'NONE',  ( -25.57682740168942814, 5.495034664247683054, 164.9437814717017545 ) ) ;
#101268=CARTESIAN_POINT ( 'NONE',  ( 28.82186960331499392, -9.364793116373510529, 141.1500000054623740 ) ) ;
#101280=AXIS2_PLACEMENT_3D ( 'NONE', #4962, #21144, #82799 ) ;
#101282=CARTESIAN_POINT ( 'NONE',  ( 1.784210473542230573E-15, -29.16686587814331588, 145.8750000027311557 ) ) ;
#101339=DIRECTION ( 'NONE',  ( 0.8660254037844410391, 0.000000000000000000, 0.4999999999999958367 ) ) ;
#101352=CYLINDRICAL_SURFACE ( 'NONE', #144442, 2.000000000000001776 ) ;
#101394=CARTESIAN_POINT ( 'NONE',  ( 21.51693143705272959, 10.15780255052816550, 170.5200780514257133 ) ) ;
#101406=ADVANCED_FACE ( 'NONE', ( #158667 ), #38325, .T. ) ;
#101407=CARTESIAN_POINT ( 'NONE',  ( -23.31738231874055245, -16.94106989632524574, 146.1999999999999886 ) ) ;
#101469=CARTESIAN_POINT ( 'NONE',  ( -27.19095269391954517, 8.032454009542490780, 149.5864051666458181 ) ) ;
#101496=CARTESIAN_POINT ( 'NONE',  ( -26.58496454517000629, 7.626754437231443084, 167.9682100371138915 ) ) ;
#101555=CARTESIAN_POINT ( 'NONE',  ( -20.85011945226398566, -10.59319688750118083, 168.2343749380337954 ) ) ;
#101580=EDGE_CURVE ( 'NONE', #56947, #45770, #97966, .T. ) ;
#101656=ADVANCED_FACE ( 'NONE', ( #144492, #162665 ), #100981, .F. ) ;
#101710=CARTESIAN_POINT ( 'NONE',  ( 23.29544513554940011, 16.92513159979228021, 147.1843446568999809 ) ) ;
#101739=VERTEX_POINT ( 'NONE', #52484 ) ;
#101767=CARTESIAN_POINT ( 'NONE',  ( -27.73933785331498925, 2.428612866367529932E-14, 147.3750000027311842 ) ) ;
#101773=CARTESIAN_POINT ( 'NONE',  ( -20.14845677604829888, -11.63499142542225329, 168.0304984204095149 ) ) ;
#101810=CARTESIAN_POINT ( 'NONE',  ( 24.24393946302988212, -5.863316274099129366, 172.4343578713345266 ) ) ;
#101917=CARTESIAN_POINT ( 'NONE',  ( 21.75500197730212903, 5.836128546636256686, 172.5265712840238734 ) ) ;
#101952=CARTESIAN_POINT ( 'NONE',  ( -20.96276500525453912, 10.40013546722647853, 168.2886347277375592 ) ) ;
#101974=VERTEX_POINT ( 'NONE', #189038 ) ;
#102041=CARTESIAN_POINT ( 'NONE',  ( 22.77340942535172985, -12.66915129224429926, 165.5704402759698723 ) ) ;
#102177=ORIENTED_EDGE ( 'NONE', *, *, #142029, .F. ) ;
#102207=CARTESIAN_POINT ( 'NONE',  ( -25.77168321198461598, 6.124454116751229193, 163.0898522765303085 ) ) ;
#102213=CARTESIAN_POINT ( 'NONE',  ( -27.96892006433829181, 7.184979517970726981, 161.0508495487520406 ) ) ;
#102238=ORIENTED_EDGE ( 'NONE', *, *, #194670, .F. ) ;
#102288=CARTESIAN_POINT ( 'NONE',  ( 22.44159573604009594, -16.30477369853687364, 142.1750000027311671 ) ) ;
#102289=CARTESIAN_POINT ( 'NONE',  ( -5.429308488886486681E-15, 30.30510711980690175, 139.7500000054623683 ) ) ;
#102301=CARTESIAN_POINT ( 'NONE',  ( 8.571926809382597767, 26.38167802310806209, 146.7750000027311899 ) ) ;
#102371=CARTESIAN_POINT ( 'NONE',  ( -21.04946095171258236, 10.86023174791543866, 170.2405914574444239 ) ) ;
#102425=CARTESIAN_POINT ( 'NONE',  ( 28.82186960331499392, -9.364793116373510529, 148.9000000000000057 ) ) ;
#102468=AXIS2_PLACEMENT_3D ( 'NONE', #94558, #553, #167449 ) ;
#102493=MECHANICAL_DESIGN_GEOMETRIC_PRESENTATION_REPRESENTATION('',(#112150),#176833);
#102533=ORIENTED_EDGE ( 'NONE', *, *, #15702, .F. ) ;
#102573=CARTESIAN_POINT ( 'NONE',  ( -27.19095269391954517, -8.032454009542492557, 149.5864051666458181 ) ) ;
#102586=CARTESIAN_POINT ( 'NONE',  ( 27.73933785331498925, -9.013057229001034898, 145.7750000027311899 ) ) ;
#102772=CARTESIAN_POINT ( 'NONE',  ( 8.571926809382597767, 26.38167802310806209, 146.7750000027311899 ) ) ;
#102781=AXIS2_PLACEMENT_3D ( 'NONE', #190783, #173635, #80601 ) ;
#102808=EDGE_CURVE ( 'NONE', #33383, #136214, #179642, .T. ) ;
#102815=CARTESIAN_POINT ( 'NONE',  ( 24.40828949532303227, -2.848420800297167599, 173.9378174459542663 ) ) ;
#102950=CARTESIAN_POINT ( 'NONE',  ( -20.61108013404310668, 10.97331748574079491, 168.1441487092658349 ) ) ;
#103016=CARTESIAN_POINT ( 'NONE',  ( -21.77219501682365532, 9.607313489129737150, 170.8391438706019585 ) ) ;
#103022=LINE ( 'NONE', #87839, #193101 ) ;
#103077=( BOUNDED_SURFACE ( )  B_SPLINE_SURFACE ( 1, 2, ( 
 ( #100756, #135124, #195807, #42114, #56265, #192788, #103776, #148282, #87596, #116933, #193796, #146262, #88594, #7746, #131100, #177632, #132105, #86599, #133103, #117948, #101767, #39100, #179638, #163454, #9775, #41108, #102772, #25953, #105754, #184588, #107723, #15737, #138080, #74434, #62215, #92558, #90578, #123883, #198772, #169404, #185581, #91553, #152259, #30910, #77396, #136101, #76404, #119935, #14743, #183602, #167440, #122899, #197777, #199761, #46069, #154246, #60238, #182611, #151281, #43100, #106743, #45086, #139066, #544, #28937, #12770, #181620, #13744, #166456, #59243, #104768, #153240, #61228, #27953, #121909, #168418, #89594, #120912, #44096, #75412, #29913, #137084, #148939, #162097, #195456, #56931, #70093, #134776, #165107, #42759, #25610, #87254, #135765, #41763, #23593, #26600, #197436, #85240, #131762, #71091, #164112 ),
 ( #193444, #58902, #194445, #10429, #118605, #180295, #132758, #182262, #103428, #54920, #55916, #102425, #72087, #146931, #117590, #57928, #181282, #89247, #149928, #178281, #120568, #166105, #179292, #100416, #133761, #104422, #8421, #88243, #40756, #27607, #74095, #39744, #11435, #116592, #73106, #196458, #119599, #150939, #101407, #12433, #163100, #24603, #86250, #147940, #9426, #105410, #77048, #153895, #16388, #124549, #76055, #75069, #78035, #199415, #167094, #198417, #94200, #138719, #200, #139704, #122556, #30558, #154890, #1191, #61869, #2198, #28595, #15391, #92210, #90233, #59894, #62867, #123539, #151916, #91203, #186246, #47724, #125550, #185232, #43747, #13405, #46723, #170063, #137731, #121561, #108386, #31553, #140708, #93205, #109375, #183256, #171057, #63879, #152893, #136735, #32547, #44737, #106393, #79033, #155880, #107380 ) ),
 .UNSPECIFIED., .F., .F., .F. ) 
 B_SPLINE_SURFACE_WITH_KNOTS ( ( 2, 2 ),
 ( 3, 2, 2, 2, 2, 2, 2, 2, 2, 2, 2, 2, 2, 2, 2, 2, 2, 2, 2, 2, 2, 2, 2, 2, 2, 2, 2, 2, 2, 2, 2, 2, 2, 2, 2, 2, 2, 2, 2, 2, 2, 2, 2, 2, 2, 2, 2, 2, 2, 2, 3 ),
 ( 0.000000000000000000, 1.000000000000000000 ),
 ( 0.000000000000000000, 0.02000000000000000042, 0.04000000000000000083, 0.05999999999999999778, 0.08000000000000000167, 0.1000000000000000056, 0.1199999999999999956, 0.1400000000000000133, 0.1600000000000000033, 0.1799999999999999933, 0.2000000000000000111, 0.2200000000000000011, 0.2399999999999999911, 0.2600000000000000089, 0.2800000000000000266, 0.2999999999999999889, 0.3200000000000000067, 0.3400000000000000244, 0.3599999999999999867, 0.3800000000000000044, 0.4000000000000000222, 0.4199999999999999845, 0.4400000000000000022, 0.4600000000000000200, 0.4799999999999999822, 0.5000000000000000000, 0.5200000000000000178, 0.5400000000000000355, 0.5600000000000000533, 0.5799999999999999600, 0.5999999999999999778, 0.6199999999999999956, 0.6400000000000000133, 0.6600000000000000311, 0.6800000000000000488, 0.6999999999999999556, 0.7199999999999999734, 0.7399999999999999911, 0.7600000000000000089, 0.7800000000000000266, 0.8000000000000000444, 0.8199999999999999512, 0.8399999999999999689, 0.8599999999999999867, 0.8800000000000000044, 0.9000000000000000222, 0.9200000000000000400, 0.9399999999999999467, 0.9599999999999999645, 0.9799999999999999822, 1.000000000000000000 ),
 .UNSPECIFIED. ) 
 GEOMETRIC_REPRESENTATION_ITEM ( )  RATIONAL_B_SPLINE_SURFACE ( (
 ( 1.000000000000000000, 0.9510565162951535312, 1.000000000000000000, 0.9510565162951535312, 1.000000000000000000, 0.9510565162951535312, 1.000000000000000000, 0.9510565162951535312, 1.000000000000000000, 0.9510565162951535312, 1.000000000000000000, 0.9510565162951535312, 1.000000000000000000, 0.9510565162951535312, 1.000000000000000000, 0.9510565162951535312, 1.000000000000000000, 0.9510565162951535312, 1.000000000000000000, 0.9510565162951535312, 1.000000000000000000, 0.9510565162951535312, 1.000000000000000000, 0.9510565162951535312, 1.000000000000000000, 0.9510565162951535312, 1.000000000000000000, 0.9510565162951535312, 1.000000000000000000, 0.9510565162951535312, 1.000000000000000000, 0.9510565162951535312, 1.000000000000000000, 0.9510565162951535312, 1.000000000000000000, 0.9510565162951535312, 1.000000000000000000, 0.9510565162951535312, 1.000000000000000000, 0.9510565162951535312, 1.000000000000000000, 0.9510565162951535312, 1.000000000000000000, 0.9510565162951535312, 1.000000000000000000, 0.9510565162951535312, 1.000000000000000000, 0.9510565162951535312, 1.000000000000000000, 0.9510565162951535312, 1.000000000000000000, 0.9510565162951535312, 1.000000000000000000, 0.9510565162951535312, 1.000000000000000000, 0.9510565162951535312, 1.000000000000000000, 0.9510565162951535312, 1.000000000000000000, 0.9510565162951535312, 1.000000000000000000, 0.9510565162951535312, 1.000000000000000000, 0.9510565162951535312, 1.000000000000000000, 0.9510565162951535312, 1.000000000000000000, 0.9510565162951535312, 1.000000000000000000, 0.9510565162951535312, 1.000000000000000000, 0.9510565162951535312, 1.000000000000000000, 0.9510565162951535312, 1.000000000000000000, 0.9510565162951535312, 1.000000000000000000, 0.9510565162951535312, 1.000000000000000000, 0.9510565162951535312, 1.000000000000000000, 0.9510565162951535312, 1.000000000000000000, 0.9510565162951535312, 1.000000000000000000, 0.9510565162951535312, 1.000000000000000000, 0.9510565162951535312, 1.000000000000000000, 0.9510565162951535312, 1.000000000000000000, 0.9510565162951535312, 1.000000000000000000, 0.9510565162951535312, 1.000000000000000000, 0.9510565162951535312, 1.000000000000000000, 0.9510565162951535312, 1.000000000000000000, 0.9510565162951535312, 1.000000000000000000),
 ( 1.000000000000000000, 0.9510565162951535312, 1.000000000000000000, 0.9510565162951535312, 1.000000000000000000, 0.9510565162951535312, 1.000000000000000000, 0.9510565162951535312, 1.000000000000000000, 0.9510565162951535312, 1.000000000000000000, 0.9510565162951535312, 1.000000000000000000, 0.9510565162951535312, 1.000000000000000000, 0.9510565162951535312, 1.000000000000000000, 0.9510565162951535312, 1.000000000000000000, 0.9510565162951535312, 1.000000000000000000, 0.9510565162951535312, 1.000000000000000000, 0.9510565162951535312, 1.000000000000000000, 0.9510565162951535312, 1.000000000000000000, 0.9510565162951535312, 1.000000000000000000, 0.9510565162951535312, 1.000000000000000000, 0.9510565162951535312, 1.000000000000000000, 0.9510565162951535312, 1.000000000000000000, 0.9510565162951535312, 1.000000000000000000, 0.9510565162951535312, 1.000000000000000000, 0.9510565162951535312, 1.000000000000000000, 0.9510565162951535312, 1.000000000000000000, 0.9510565162951535312, 1.000000000000000000, 0.9510565162951535312, 1.000000000000000000, 0.9510565162951535312, 1.000000000000000000, 0.9510565162951535312, 1.000000000000000000, 0.9510565162951535312, 1.000000000000000000, 0.9510565162951535312, 1.000000000000000000, 0.9510565162951535312, 1.000000000000000000, 0.9510565162951535312, 1.000000000000000000, 0.9510565162951535312, 1.000000000000000000, 0.9510565162951535312, 1.000000000000000000, 0.9510565162951535312, 1.000000000000000000, 0.9510565162951535312, 1.000000000000000000, 0.9510565162951535312, 1.000000000000000000, 0.9510565162951535312, 1.000000000000000000, 0.9510565162951535312, 1.000000000000000000, 0.9510565162951535312, 1.000000000000000000, 0.9510565162951535312, 1.000000000000000000, 0.9510565162951535312, 1.000000000000000000, 0.9510565162951535312, 1.000000000000000000, 0.9510565162951535312, 1.000000000000000000, 0.9510565162951535312, 1.000000000000000000, 0.9510565162951535312, 1.000000000000000000, 0.9510565162951535312, 1.000000000000000000, 0.9510565162951535312, 1.000000000000000000, 0.9510565162951535312, 1.000000000000000000, 0.9510565162951535312, 1.000000000000000000, 0.9510565162951535312, 1.000000000000000000, 0.9510565162951535312, 1.000000000000000000, 0.9510565162951535312, 1.000000000000000000) ) ) 
 REPRESENTATION_ITEM ( '' )  SURFACE ( )  );
#103106=CARTESIAN_POINT ( 'NONE',  ( -27.96809023454855492, -7.159247544375828554, 161.0916313341220416 ) ) ;
#103252=VERTEX_POINT ( 'NONE', #41332 ) ;
#103264=EDGE_CURVE ( 'NONE', #75663, #131752, #69112, .T. ) ;
#103291=CARTESIAN_POINT ( 'NONE',  ( -17.81289503416611808, 24.51734667627700404, 141.9500000054623285 ) ) ;
#103293=CARTESIAN_POINT ( 'NONE',  ( -3.573655867282028392E-15, 12.39993551617566681, 175.0000000000000000 ) ) ;
#103294=ORIENTED_EDGE ( 'NONE', *, *, #69903, .F. ) ;
#103327=CIRCLE ( 'NONE', #197010, 3.000000000000001776 ) ;
#103373=DIRECTION ( 'NONE',  ( -0.1039620511844979445, -0.1039620511844979445, -0.9891328443778539814 ) ) ;
#103374=CARTESIAN_POINT ( 'NONE',  ( -25.47140278216145859, 9.703455644539296543, 170.7619267275324262 ) ) ;
#103428=CARTESIAN_POINT ( 'NONE',  ( 23.31738231874054534, 16.94106989632529192, 149.1999999999999886 ) ) ;
#103538=AXIS2_PLACEMENT_3D ( 'NONE', #7423, #115624, #129756 ) ;
#103545=CARTESIAN_POINT ( 'NONE',  ( 19.49401214000073779, -12.39993551617566503, 167.9999999999999716 ) ) ;
#103588=CARTESIAN_POINT ( 'NONE',  ( 27.73933785331498925, -9.013057229001034898, 147.7750000027311899 ) ) ;
#103776=CARTESIAN_POINT ( 'NONE',  ( 8.571926809382597767, 26.38167802310806209, 148.7750000027311899 ) ) ;
#103815=CARTESIAN_POINT ( 'NONE',  ( 23.14613071126333921, -10.96668486446927204, 168.1016194467971445 ) ) ;
#103946=ORIENTED_EDGE ( 'NONE', *, *, #163400, .F. ) ;
#104038=CARTESIAN_POINT ( 'NONE',  ( 24.79445957992280469, -6.337972767934337170, 168.1743082258862785 ) ) ;
#104106=EDGE_CURVE ( 'NONE', #199519, #144964, #162721, .T. ) ;
#104115=CARTESIAN_POINT ( 'NONE',  ( 24.27957997113399102, 6.290849861789209463, 171.5443985711292214 ) ) ;
#104178=ORIENTED_EDGE ( 'NONE', *, *, #175605, .F. ) ;
#104232=ORIENTED_EDGE ( 'NONE', *, *, #38420, .F. ) ;
#104285=CARTESIAN_POINT ( 'NONE',  ( -22.44159573604010305, 16.30477369853692338, 144.6750000027311671 ) ) ;
#104287=CYLINDRICAL_SURFACE ( 'NONE', #155605, 7.000000000000006217 ) ;
#104365=CARTESIAN_POINT ( 'NONE',  ( -1.435302771838241620, -27.95353791037918256, 140.0000000000001421 ) ) ;
#104422=CARTESIAN_POINT ( 'NONE',  ( -5.429308488886486681E-15, 30.30510711980690175, 147.5000000000000000 ) ) ;
#104490=EDGE_CURVE ( 'NONE', #69189, #83996, #169410, .T. ) ;
#104562=CARTESIAN_POINT ( 'NONE',  ( -21.44939319537014200, -9.428468639168981369, 168.6471776813584995 ) ) ;
#104760=VERTEX_POINT ( 'NONE', #36853 ) ;
#104768=CARTESIAN_POINT ( 'NONE',  ( 27.73933785331498569, 2.768321779492822058E-14, 142.3750000027311842 ) ) ;
#104807=CARTESIAN_POINT ( 'NONE',  ( -20.69372460268612457, -11.29034304323151616, 170.1224388339879567 ) ) ;
#104984=CARTESIAN_POINT ( 'NONE',  ( 26.56065628307859683, 7.402157598701552210, 155.5832749335749270 ) ) ;
#105007=CARTESIAN_POINT ( 'NONE',  ( -20.51359854606067401, -11.49117151696134087, 170.0775129446642779 ) ) ;
#105010=EDGE_CURVE ( 'NONE', #95658, #135939, #128556, .T. ) ;
#105011=B_SPLINE_CURVE_WITH_KNOTS ( 'NONE', 3,
 ( #62579, #184944, #112080, #46429, #79751, #141421, #31266, #177755, #35236, #176758, #130208, #96890, #38231, #191903, #98878, #99886, #131228, #158573, #4881, #113060, #67557, #20062, #55387, #161571, #51400, #53388, #160573, #174752 ),
 .UNSPECIFIED., .F., .F.,
 ( 4, 2, 2, 2, 2, 2, 2, 2, 2, 2, 2, 2, 2, 4 ),
 ( 3.084931484532069451E-17, 0.0005512667261461084295, 0.001102533452292185851, 0.001240350133828705152, 0.001378166815365224453, 0.001447075156133462853, 0.001515983496901700820, 0.001653800178438180439, 0.001929433541511138593, 0.002205066904584096748, 0.003307600356875847400, 0.004410133809167598486, 0.006615200713751101524, 0.008820267618334603696 ),
 .UNSPECIFIED. ) ;
#105023=ORIENTED_EDGE ( 'NONE', *, *, #136828, .T. ) ;
#105032=CARTESIAN_POINT ( 'NONE',  ( 17.79613651744294245, -24.49428055684527195, 146.6843446569000093 ) ) ;
#105114=CARTESIAN_POINT ( 'NONE',  ( -8.571926809382608425, 26.38167802310805854, 144.4750000027312069 ) ) ;
#105122=AXIS2_PLACEMENT_3D ( 'NONE', #97343, #33712, #80204 ) ;
#105181=DIRECTION ( 'NONE',  ( 0.000000000000000000, 0.000000000000000000, -1.000000000000000000 ) ) ;
#105236=DIRECTION ( 'NONE',  ( 0.000000000000000000, 0.000000000000000000, 1.000000000000000000 ) ) ;
#105273=CARTESIAN_POINT ( 'NONE',  ( -27.73933785331498925, -9.013057229001049109, 144.9750000027312069 ) ) ;
#105284=DIRECTION ( 'NONE',  ( 0.000000000000000000, 0.000000000000000000, -1.000000000000000000 ) ) ;
#105306=VERTEX_POINT ( 'NONE', #27716 ) ;
#105343=CARTESIAN_POINT ( 'NONE',  ( -22.96528548301343520, 5.795830589372932273, 190.0000000000000000 ) ) ;
#105351=CARTESIAN_POINT ( 'NONE',  ( -18.50817386519043595, -21.48060456978424781, 139.9999999999999716 ) ) ;
#105410=CARTESIAN_POINT ( 'NONE',  ( -5.429308488886486681E-15, 30.30510711980690175, 145.4999999999999432 ) ) ;
#105434=CARTESIAN_POINT ( 'NONE',  ( -23.14225647005877917, 5.657937718899317403, 172.1775255543086018 ) ) ;
#105511=CARTESIAN_POINT ( 'NONE',  ( -24.17640770809926565, -7.553848413216235791, 169.9412368235645943 ) ) ;
#105635=ORIENTED_EDGE ( 'NONE', *, *, #59575, .T. ) ;
#105700=CARTESIAN_POINT ( 'NONE',  ( 21.38418241377623019, -5.438282248597753110, 174.2683007571264113 ) ) ;
#105726=VERTEX_POINT ( 'NONE', #103545 ) ;
#105754=CARTESIAN_POINT ( 'NONE',  ( 22.44159573604009239, 16.30477369853692693, 146.5750000027312012 ) ) ;
#105758=CARTESIAN_POINT ( 'NONE',  ( -22.44159573604009950, -16.30477369853688430, 143.5750000027311728 ) ) ;
#105784=VECTOR ( 'NONE', #56521, 1000.000000000000000 ) ;
#105795=CARTESIAN_POINT ( 'NONE',  ( -26.77293948118418854, -6.014770499717744912, 169.2063755025621674 ) ) ;
#105841=LINE ( 'NONE', #56351, #114511 ) ;
#105992=CARTESIAN_POINT ( 'NONE',  ( -19.76520975163527538, -12.18675982963091897, 170.0000000000000000 ) ) ;
#106094=CARTESIAN_POINT ( 'NONE',  ( -8.571926809382601320, -26.38167802310801591, 145.2750000027311899 ) ) ;
#106109=B_SPLINE_CURVE_WITH_KNOTS ( 'NONE', 3,
 ( #84730, #56415, #38251, #101917, #193946, #161591, #164600, #72592, #177775, #163599, #86742, #148427, #134266, #146408, #9922, #100901, #57426, #162585, #71581, #88742 ),
 .UNSPECIFIED., .F., .F.,
 ( 4, 2, 2, 2, 2, 2, 2, 2, 2, 4 ),
 ( 0.000000000000000000, 0.001368201656092171790, 0.002736403312184343579, 0.004104604968276515803, 0.005472806624368687159, 0.006841008280460856780, 0.008209209936553026402, 0.008893310764599102539, 0.009577411592645178676, 0.01094561324873732401 ),
 .UNSPECIFIED. ) ;
#106154=CARTESIAN_POINT ( 'NONE',  ( 26.03370437638686852, 6.875205692009825675, 160.5968874236875195 ) ) ;
#106182=CARTESIAN_POINT ( 'NONE',  ( -26.58496454517000629, 7.626754437231443084, 167.9682100371138915 ) ) ;
#106184=DIRECTION ( 'NONE',  ( -0.000000000000000000, 1.000000000000000000, -0.000000000000000000 ) ) ;
#106256=CARTESIAN_POINT ( 'NONE',  ( -22.44159573604009950, -16.30477369853688430, 141.0750000027311728 ) ) ;
#106334=CARTESIAN_POINT ( 'NONE',  ( -4.817327537821083361, -27.72747260876182551, 139.9999999999999432 ) ) ;
#106364=( BOUNDED_CURVE ( )  B_SPLINE_CURVE ( 2, ( #128695, #158057, #36686, #189405, #160045, #21532, #111551, #83193, #80211, #187430, #37696 ),
 .UNSPECIFIED., .F., .T. ) 
 B_SPLINE_CURVE_WITH_KNOTS ( ( 3, 2, 2, 2, 2, 3 ),
 ( 0.5000000000000032196, 0.5200000000000032374, 0.5400000000000032552, 0.5600000000000033840, 0.5800000000000032907, 0.6000000000000033085 ),
 .UNSPECIFIED. ) 
 CURVE ( )  GEOMETRIC_REPRESENTATION_ITEM ( )  RATIONAL_B_SPLINE_CURVE ( ( 0.9999999999999921174, 0.9510565162951614138, 1.000000000000000000, 0.9510565162951535312, 1.000000000000000000, 0.9510565162951535312, 1.000000000000000000, 0.9510565162951535312, 1.000000000000000000, 0.9510565162951454266, 1.000000000000008216 ) ) 
 REPRESENTATION_ITEM ( '' )  );
#106378=ORIENTED_EDGE ( 'NONE', *, *, #124946, .F. ) ;
#106379=CARTESIAN_POINT ( 'NONE',  ( 21.92083080610932200, 8.096106818377439396, 172.4353877980870493 ) ) ;
#106393=CARTESIAN_POINT ( 'NONE',  ( -17.81289503416611097, -24.51734667627696496, 140.2999999999999545 ) ) ;
#106493=CARTESIAN_POINT ( 'NONE',  ( -24.04614410381461553, -5.408324479809799357, 174.2944578187863840 ) ) ;
#106573=CARTESIAN_POINT ( 'NONE',  ( -28.79475375365586842, 2.428612866367529932E-14, 147.9843446568999923 ) ) ;
#106632=VECTOR ( 'NONE', #117767, 1000.000000000000000 ) ;
#106636=EDGE_CURVE ( 'NONE', #131506, #140232, #173115, .T. ) ;
#106743=CARTESIAN_POINT ( 'NONE',  ( -27.73933785331498925, 2.428612866367529932E-14, 143.3750000027311842 ) ) ;
#106747=CARTESIAN_POINT ( 'NONE',  ( 27.73933785331498925, -9.013057229001033122, 146.2750000027311899 ) ) ;
#106783=CARTESIAN_POINT ( 'NONE',  ( -25.04733094907770763, -10.92720321514065418, 170.1247377027656285 ) ) ;
#106812=EDGE_LOOP ( 'NONE', ( #172273, #12211, #95417, #147012, #86243, #164100 ) ) ;
#106833=DIRECTION ( 'NONE',  ( 0.1039620511844979306, 0.1039620511844979306, 0.9891328443778538704 ) ) ;
#106919=CARTESIAN_POINT ( 'NONE',  ( -21.97154029300585520, 7.270820338085815848, 170.2141396987978794 ) ) ;
#107080=CARTESIAN_POINT ( 'NONE',  ( -8.571926809382601320, -26.38167802310801591, 143.2750000027311899 ) ) ;
#107119=CARTESIAN_POINT ( 'NONE',  ( -27.74069374691385192, -6.311165852667877552, 163.4895129000211114 ) ) ;
#107243=CARTESIAN_POINT ( 'NONE',  ( 22.44159573604009239, 16.30477369853692693, 142.0750000027311728 ) ) ;
#107380=CARTESIAN_POINT ( 'NONE',  ( -28.82186960331499037, 2.428612866367529932E-14, 139.9999999999999716 ) ) ;
#107455=EDGE_LOOP ( 'NONE', ( #106378, #157458, #190914, #113337, #87272, #78132, #198230, #180194, #81602, #114329, #147252, #80826 ) ) ;
#107476=CARTESIAN_POINT ( 'NONE',  ( -21.56952297831670151, -5.557039098534934496, 173.4609804364286276 ) ) ;
#107578=B_SPLINE_CURVE_WITH_KNOTS ( 'NONE', 3,
 ( #28196, #153488, #72690, #138322, #122150, #200004, #179884, #41352, #103016, #164699, #26195, #155481, #109969, #17976, #140302, #61470, #33138, #16973 ),
 .UNSPECIFIED., .F., .F.,
 ( 4, 2, 2, 2, 2, 2, 2, 2, 4 ),
 ( 3.878959614448864246E-18, 0.001023866006848668780, 0.002047732013697333656, 0.003071598020545998533, 0.004095464027394662976, 0.005119330034243327852, 0.006143196041091992729, 0.007167062047940657606, 0.008190928054789322482 ),
 .UNSPECIFIED. ) ;
#107606=VERTEX_POINT ( 'NONE', #14020 ) ;
#107664=VERTEX_POINT ( 'NONE', #59522 ) ;
#107667=CARTESIAN_POINT ( 'NONE',  ( 19.49401214000073779, -12.39993551617566503, 167.9999999999999716 ) ) ;
#107723=CARTESIAN_POINT ( 'NONE',  ( 27.73933785331498569, 2.768321779492822058E-14, 146.3750000027311842 ) ) ;
#107727=CARTESIAN_POINT ( 'NONE',  ( -27.73933785331498925, 2.428612866367529932E-14, 145.3750000027311842 ) ) ;
#107762=CARTESIAN_POINT ( 'NONE',  ( -26.79623349963142331, -5.044589688426236229, 170.2051123914322375 ) ) ;
#107790=VERTEX_POINT ( 'NONE', #45366 ) ;
#107900=EDGE_LOOP ( 'NONE', ( #17150, #140022, #180284 ) ) ;
#107934=CARTESIAN_POINT ( 'NONE',  ( -28.79475375365676726, -9.355982642737950883, 144.3656553485623704 ) ) ;
#108009=CARTESIAN_POINT ( 'NONE',  ( -21.94905633995364269, 7.481063542984161430, 170.0146117665088923 ) ) ;
#108050=DIRECTION ( 'NONE',  ( -1.000000000000000000, 0.000000000000000000, 0.000000000000000000 ) ) ;
#108074=CARTESIAN_POINT ( 'NONE',  ( -22.44159573604010305, 16.30477369853692338, 144.6750000027311671 ) ) ;
#108088=CARTESIAN_POINT ( 'NONE',  ( -25.63014143074632400, -6.600872056147844447, 163.2069976173303871 ) ) ;
#108149=ADVANCED_FACE ( 'NONE', ( #135405 ), #111103, .F. ) ;
#108244=CARTESIAN_POINT ( 'NONE',  ( -8.571926809382601320, -26.38167802310801591, 143.2750000027311899 ) ) ;
#108252=CARTESIAN_POINT ( 'NONE',  ( 21.94381615377040973, -13.26253372808111308, 167.9278110240102251 ) ) ;
#108323=CARTESIAN_POINT ( 'NONE',  ( -26.61723430050333050, 3.645106422946821301, 172.4622069319858895 ) ) ;
#108386=CARTESIAN_POINT ( 'NONE',  ( -5.429308488886486681E-15, 30.30510711980690175, 141.5000000000000000 ) ) ;
#108398=CARTESIAN_POINT ( 'NONE',  ( 26.57611637973592877, -7.696099174150921485, 167.9177021574032267 ) ) ;
#108519=CARTESIAN_POINT ( 'NONE',  ( -26.58496454516998853, -7.626754437231455519, 167.9682100371138915 ) ) ;
#108560=CARTESIAN_POINT ( 'NONE',  ( 17.79613651744294245, -24.49428055684527195, 148.6843446568999809 ) ) ;
#108610=ORIENTED_EDGE ( 'NONE', *, *, #151508, .T. ) ;
#108647=CARTESIAN_POINT ( 'NONE',  ( 10.65970682939788716, -25.60940286011448919, 139.9999999999999716 ) ) ;
#108672=CARTESIAN_POINT ( 'NONE',  ( 21.75476783670601222, -5.835674035550355576, 172.5278397751181387 ) ) ;
#108683=PLANE ( 'NONE',  #134581 ) ;
#108735=CARTESIAN_POINT ( 'NONE',  ( -17.14385361876520619, 23.59649016807275856, 147.0750000027311728 ) ) ;
#108876=DIRECTION ( 'NONE',  ( -1.000000000000000000, 0.000000000000000000, 0.000000000000000000 ) ) ;
#108979=VECTOR ( 'NONE', #57717, 1000.000000000000114 ) ;
#109015=CARTESIAN_POINT ( 'NONE',  ( -24.66578506923906033, 3.377805382905409104, 172.1149105766468494 ) ) ;
#109079=CARTESIAN_POINT ( 'NONE',  ( -17.14385361876520264, -23.59649016807271593, 147.1750000027311671 ) ) ;
#109187=ORIENTED_EDGE ( 'NONE', *, *, #93066, .F. ) ;
#109238=CARTESIAN_POINT ( 'NONE',  ( 17.14385361876520264, 23.59649016807275856, 140.1750000027311955 ) ) ;
#109245=CARTESIAN_POINT ( 'NONE',  ( 20.56371838171487454, -11.04494471775322495, 168.1294998094270170 ) ) ;
#109375=CARTESIAN_POINT ( 'NONE',  ( 28.82186960331498327, 9.364793116373570925, 141.0999999999999943 ) ) ;
#109390=CARTESIAN_POINT ( 'NONE',  ( 26.73207562759457190, -6.543912086049391341, 168.7462576975893285 ) ) ;
#109400=CARTESIAN_POINT ( 'NONE',  ( -24.27707668318815237, 5.858708095980201591, 170.2635530474734651 ) ) ;
#109471=CARTESIAN_POINT ( 'NONE',  ( -24.73536985823983869, -3.645104810711615961, 171.5180696409408085 ) ) ;
#109537=DIRECTION ( 'NONE',  ( 0.000000000000000000, 0.000000000000000000, -1.000000000000000000 ) ) ;
#109599=VERTEX_POINT ( 'NONE', #15525 ) ;
#109641=CARTESIAN_POINT ( 'NONE',  ( 27.51614237185798117, -3.626410569495110980, 140.0000000000000000 ) ) ;
#109772=AXIS2_PLACEMENT_3D ( 'NONE', #139602, #182161, #15286 ) ;
#109969=CARTESIAN_POINT ( 'NONE',  ( -21.94207162742807071, 8.184381772639664376, 172.2902002187020116 ) ) ;
#110008=CARTESIAN_POINT ( 'NONE',  ( -24.27995301597377775, 6.552671593954475071, 171.1165850637241874 ) ) ;
#110071=CARTESIAN_POINT ( 'NONE',  ( 19.76520975163528249, 12.18675982963092075, 169.9999999999999716 ) ) ;
#110076=CARTESIAN_POINT ( 'NONE',  ( -27.73933785331498925, -9.013057229001049109, 140.9750000027311501 ) ) ;
#110081=VERTEX_POINT ( 'NONE', #194347 ) ;
#110090=CARTESIAN_POINT ( 'NONE',  ( -25.22510128165246712, -6.326562104755758753, 165.8168824682947502 ) ) ;
#110162=CARTESIAN_POINT ( 'NONE',  ( -24.37439536253436501, -13.84063584238319500, 165.9041067986157998 ) ) ;
#110272=EDGE_CURVE ( 'NONE', #139247, #107606, #117079, .T. ) ;
#110300=CARTESIAN_POINT ( 'NONE',  ( 22.24685556490157978, 12.75834802357609377, 167.9013491530738520 ) ) ;
#110383=CARTESIAN_POINT ( 'NONE',  ( 26.13941622279003951, -9.616497135381504080, 166.9083969906208722 ) ) ;
#110389=CARTESIAN_POINT ( 'NONE',  ( 20.02432819973540035, -11.96332215053014991, 170.0134113894037000 ) ) ;
#110400=DIRECTION ( 'NONE',  ( -0.000000000000000000, -0.000000000000000000, 1.000000000000000000 ) ) ;
#110416=AXIS2_PLACEMENT_3D ( 'NONE', #53546, #176916, #38387 ) ;
#110464=CARTESIAN_POINT ( 'NONE',  ( 28.82186960331499392, -9.364793116373510529, 145.1500000054623456 ) ) ;
#110478=CARTESIAN_POINT ( 'NONE',  ( -8.571926809382608425, 26.38167802310805854, 148.9750000027311785 ) ) ;
#110716=DIRECTION ( 'NONE',  ( -1.000000000000000000, 0.000000000000000000, 0.000000000000000000 ) ) ;
#110836=CARTESIAN_POINT ( 'NONE',  ( -21.38418241377623374, -7.427326039334300134, 174.4773576836617224 ) ) ;
#110863=DIRECTION ( 'NONE',  ( 0.000000000000000000, 0.000000000000000000, -1.000000000000000000 ) ) ;
#110965=ORIENTED_EDGE ( 'NONE', *, *, #76057, .F. ) ;
#110998=CARTESIAN_POINT ( 'NONE',  ( -19.49401214000077687, 12.39993551617566681, 167.9999999999999716 ) ) ;
#111019=ORIENTED_EDGE ( 'NONE', *, *, #176927, .F. ) ;
#111038=LINE ( 'NONE', #64545, #67107 ) ;
#111065=CARTESIAN_POINT ( 'NONE',  ( -8.571926809382601320, -26.38167802310801591, 141.2750000027311899 ) ) ;
#111070=ORIENTED_EDGE ( 'NONE', *, *, #17592, .T. ) ;
#111101=CARTESIAN_POINT ( 'NONE',  ( -8.898068258721469448, -27.38543819252872069, 146.6656553485624102 ) ) ;
#111103=( BOUNDED_SURFACE ( )  B_SPLINE_SURFACE ( 3, 2, ( 
 ( #166733, #28237, #110998 ),
 ( #170694, #76685, #169694 ),
 ( #123180, #32183, #126173 ),
 ( #139348, #141341, #93840 ),
 ( #33178, #154525, #111999 ),
 ( #157514, #16022, #77680 ),
 ( #94837, #2828, #155519 ),
 ( #79670, #18017, #173689 ),
 ( #80654, #78666, #140343 ),
 ( #64506, #61511, #1831 ),
 ( #49336, #827, #17014 ),
 ( #125188, #156516, #142330 ),
 ( #34168, #172684, #48354 ),
 ( #46351, #184869, #35155 ),
 ( #50341, #63513, #108009 ),
 ( #187868, #95830, #31188 ),
 ( #92840, #47360, #186884 ),
 ( #62502, #110008, #171689 ),
 ( #19008, #124173, #3810 ),
 ( #185874, #65488, #96811 ),
 ( #109015, #158497, #127150 ),
 ( #188858, #138361, #200042 ),
 ( #164252, #36141, #25747 ),
 ( #196591, #58061, #56055 ) ),
 .UNSPECIFIED., .F., .F., .T. ) 
 B_SPLINE_SURFACE_WITH_KNOTS ( ( 4, 2, 2, 2, 2, 2, 2, 2, 2, 2, 2, 4 ),
 ( 3, 3 ),
 ( -4.336808689942017736E-18, 0.001899702839891686873, 0.002849554259837532369, 0.003799405679783378082, 0.005699108519675069075, 0.006648959939620915222, 0.007598811359566760501, 0.008548662779512605780, 0.009498514199458452795, 0.01139821703935014335, 0.01329791987924183391, 0.01519762271913352447 ),
 ( 0.000000000000000000, 1.000000000000000000 ),
 .UNSPECIFIED. ) 
 GEOMETRIC_REPRESENTATION_ITEM ( )  RATIONAL_B_SPLINE_SURFACE ( (
 ( 1.000000000000000000, 0.7660444431189795678, 1.000000000000000000),
 ( 1.000000000000000000, 0.7753720600382404404, 1.000000000000000000),
 ( 1.000000000000000000, 0.7832595754285938128, 1.000000000000000000),
 ( 1.000000000000000000, 0.7928595458705487431, 1.000000000000000000),
 ( 1.000000000000000000, 0.7956872332516108370, 1.000000000000000000),
 ( 1.000000000000000000, 0.8005750596157604759, 1.000000000000000000),
 ( 1.000000000000000000, 0.8026302056541175789, 1.000000000000000000),
 ( 1.000000000000000000, 0.8075080643849508188, 1.000000000000000000),
 ( 1.000000000000000000, 0.8091143015810811079, 1.000000000000000000),
 ( 1.000000000000000000, 0.8093067629632566540, 1.000000000000000000),
 ( 1.000000000000000000, 0.8089952915731981609, 1.000000000000000000),
 ( 1.000000000000000000, 0.8076919994862008512, 1.000000000000000000),
 ( 1.000000000000000000, 0.8067078407648894389, 1.000000000000000000),
 ( 1.000000000000000000, 0.8041786842467456564, 1.000000000000000000),
 ( 1.000000000000000000, 0.8026334674876740571, 1.000000000000000000),
 ( 1.000000000000000000, 0.7990747329469689575, 1.000000000000000000),
 ( 1.000000000000000000, 0.7970509760941789645, 1.000000000000000000),
 ( 1.000000000000000000, 0.7904793850863397475, 1.000000000000000000),
 ( 1.000000000000000000, 0.7855040224313790675, 1.000000000000000000),
 ( 1.000000000000000000, 0.7751942650507511745, 1.000000000000000000),
 ( 1.000000000000000000, 0.7698260778212776545, 1.000000000000000000),
 ( 1.000000000000000000, 0.7598259884959711608, 1.000000000000000000),
 ( 1.000000000000000000, 0.7551428682221226207, 1.000000000000000000),
 ( 1.000000000000000000, 0.7510191126010858920, 1.000000000000000000) ) ) 
 REPRESENTATION_ITEM ( '' )  SURFACE ( )  );
#111152=CARTESIAN_POINT ( 'NONE',  ( 0.000000000000000000, 3.784814030245899019, 190.0000000000000000 ) ) ;
#111228=CARTESIAN_POINT ( 'NONE',  ( 8.571926809382603096, -26.38167802310801235, 139.4750000027311785 ) ) ;
#111263=CARTESIAN_POINT ( 'NONE',  ( 24.81835880841864039, -6.052260367207979996, 168.4265213779230521 ) ) ;
#111295=CARTESIAN_POINT ( 'NONE',  ( 21.35462415990330243, 9.648971641161622870, 168.5494316893080793 ) ) ;
#111380=CARTESIAN_POINT ( 'NONE',  ( 26.45763050569066266, -3.219288925403527735, 173.6696415116520598 ) ) ;
#111388=CARTESIAN_POINT ( 'NONE',  ( 21.77219501682363401, -9.607313489129742479, 170.8391438706019585 ) ) ;
#111394=CARTESIAN_POINT ( 'NONE',  ( 22.68041372103478182, -7.529096845820644646, 173.5090731399503454 ) ) ;
#111464=CARTESIAN_POINT ( 'NONE',  ( 28.82186960331498327, 9.364793116373570925, 147.3500000054623627 ) ) ;
#111551=CARTESIAN_POINT ( 'NONE',  ( -8.898068258721469448, -27.38543819252872069, 142.6656553485623817 ) ) ;
#111770=CARTESIAN_POINT ( 'NONE',  ( -28.79475375365689160, -9.355982642737773247, 140.3656553485623135 ) ) ;
#111908=CARTESIAN_POINT ( 'NONE',  ( 23.74938543818037218, 14.67923089136166936, 139.9999999999999716 ) ) ;
#111999=CARTESIAN_POINT ( 'NONE',  ( -20.69372460268614589, 10.84650605405326296, 168.1714143675833100 ) ) ;
#112041=DIRECTION ( 'NONE',  ( 0.5367108174878537641, -0.8437662581494472791, 0.000000000000000000 ) ) ;
#112045=CARTESIAN_POINT ( 'NONE',  ( 24.81835718235489807, 6.052279806424484931, 168.4265042179603142 ) ) ;
#112066=CARTESIAN_POINT ( 'NONE',  ( 22.44159573604009594, -16.30477369853687364, 141.6750000027311671 ) ) ;
#112080=CARTESIAN_POINT ( 'NONE',  ( 27.91697786073761023, -6.847065636290183832, 161.8035115693297143 ) ) ;
#112150=STYLED_ITEM ( 'NONE', ( #34551 ), #73950 ) ;
#112207=VERTEX_POINT ( 'NONE', #176946 ) ;
#112375=CARTESIAN_POINT ( 'NONE',  ( 25.55222625260920921, -11.31436996698924879, 166.3494238031457257 ) ) ;
#112415=ORIENTED_EDGE ( 'NONE', *, *, #102808, .T. ) ;
#112454=CARTESIAN_POINT ( 'NONE',  ( -17.14385361876520264, -23.59649016807271593, 145.6750000027311671 ) ) ;
#112455=CARTESIAN_POINT ( 'NONE',  ( 28.82186960331498327, 2.781578969918950771E-14, 147.2500000054623683 ) ) ;
#112467=CARTESIAN_POINT ( 'NONE',  ( 17.14385361876520264, 23.59649016807275856, 148.6750000027311387 ) ) ;
#112538=DIRECTION ( 'NONE',  ( -1.000000000000000000, 0.000000000000000000, 0.000000000000000000 ) ) ;
#112845=SHAPE_REPRESENTATION ( 'tip', ( #82054 ), #166266 ) ;
#112919=CARTESIAN_POINT ( 'NONE',  ( 27.91311885011353411, 2.428612866367529932E-14, 155.0000000000000000 ) ) ;
#112930=CARTESIAN_POINT ( 'NONE',  ( 26.24776304279840389, 7.664901067105983401, 169.1545021717930126 ) ) ;
#113060=CARTESIAN_POINT ( 'NONE',  ( 27.67867608143718527, -7.698234437107398520, 161.8893175680481704 ) ) ;
#113081=CARTESIAN_POINT ( 'NONE',  ( 28.79475375365584711, -9.355982642739206767, 147.1656553485623533 ) ) ;
#113083=CYLINDRICAL_SURFACE ( 'NONE', #170162, 1.999999999999998224 ) ;
#113134=CARTESIAN_POINT ( 'NONE',  ( -29.15849868437705439, -5.438282248597753110, 174.2683007571264113 ) ) ;
#113214=CARTESIAN_POINT ( 'NONE',  ( -5.359611314223446995E-15, 29.16686587814335496, 140.3750000027311842 ) ) ;
#113275=CARTESIAN_POINT ( 'NONE',  ( 23.14613071126502675, 10.96668486446926138, 168.1016194467927392 ) ) ;
#113337=ORIENTED_EDGE ( 'NONE', *, *, #36547, .T. ) ;
#113390=EDGE_LOOP ( 'NONE', ( #31021, #198315, #192195, #77626, #23960 ) ) ;
#113437=CARTESIAN_POINT ( 'NONE',  ( -22.44159573604009950, -16.30477369853688430, 139.5750000027311728 ) ) ;
#113438=CARTESIAN_POINT ( 'NONE',  ( 28.82186960331498327, 2.781578969918950771E-14, 143.2500000054623683 ) ) ;
#113610=CARTESIAN_POINT ( 'NONE',  ( 28.79475375365674239, 9.355982642738014832, 145.3656553485623419 ) ) ;
#113742=CARTESIAN_POINT ( 'NONE',  ( -28.79475375365586842, 2.428612866367529932E-14, 140.2656553485623760 ) ) ;
#113878=CARTESIAN_POINT ( 'NONE',  ( 27.20512408147139993, 7.754361572990046803, 164.3878212768029243 ) ) ;
#113915=CARTESIAN_POINT ( 'NONE',  ( 25.82491430096449747, 7.758527484246121375, 169.9682266581730232 ) ) ;
#113925=CARTESIAN_POINT ( 'NONE',  ( -22.65770943308886487, -11.99324031494455589, 167.9410816520763206 ) ) ;
#113963=CARTESIAN_POINT ( 'NONE',  ( 19.49401214000073779, -12.39993551617566503, 167.9999999999999716 ) ) ;
#114066=CARTESIAN_POINT ( 'NONE',  ( -27.05641397906351742, 2.428612866367529932E-14, 169.9999999999999716 ) ) ;
#114113=LINE ( 'NONE', #48504, #119188 ) ;
#114127=ADVANCED_FACE ( 'NONE', ( #26744 ), #11581, .T. ) ;
#114204=DIRECTION ( 'NONE',  ( 1.000000000000000000, 0.000000000000000000, 0.000000000000000000 ) ) ;
#114246=EDGE_CURVE ( 'NONE', #158282, #131752, #41909, .T. ) ;
#114253=CARTESIAN_POINT ( 'NONE',  ( -27.94727380668284056, -6.976214527057364556, 161.4607934398989642 ) ) ;
#114259=EDGE_CURVE ( 'NONE', #66692, #189536, #174941, .T. ) ;
#114269=CARTESIAN_POINT ( 'NONE',  ( 23.63516320021127370, 9.722623904420892416, 168.4908852323012809 ) ) ;
#114329=ORIENTED_EDGE ( 'NONE', *, *, #121851, .T. ) ;
#114379=CARTESIAN_POINT ( 'NONE',  ( 8.571926809382603096, -26.38167802310801235, 141.4750000027312069 ) ) ;
#114385=EDGE_CURVE ( 'NONE', #181921, #70413, #59283, .T. ) ;
#114438=CARTESIAN_POINT ( 'NONE',  ( 8.906447517083050158, 27.41122689804195645, 147.6500000054623740 ) ) ;
#114441=ORIENTED_EDGE ( 'NONE', *, *, #142029, .T. ) ;
#114451=CARTESIAN_POINT ( 'NONE',  ( 22.44159573604009239, 16.30477369853692693, 140.5750000027311728 ) ) ;
#114511=VECTOR ( 'NONE', #179724, 1000.000000000000114 ) ;
#114524=CARTESIAN_POINT ( 'NONE',  ( -24.86475712555796491, 11.37215039200969002, 169.9824823118007657 ) ) ;
#114558=MECHANICAL_DESIGN_GEOMETRIC_PRESENTATION_REPRESENTATION('',(#88743),#192069);
#114568=VERTEX_POINT ( 'NONE', #156014 ) ;
#114573=EDGE_LOOP ( 'NONE', ( #132080, #160855, #51392, #181181, #81285 ) ) ;
#114608=CARTESIAN_POINT ( 'NONE',  ( 8.898068258721473001, -27.38543819252872069, 144.5843446568999866 ) ) ;
#114671=CARTESIAN_POINT ( 'NONE',  ( -26.47577687012306313, 8.223210953690959002, 167.6032987643051229 ) ) ;
#114699=CARTESIAN_POINT ( 'NONE',  ( -3.573655867282028392E-15, 2.428612866367529932E-14, 155.0000000000000000 ) ) ;
#114950=PRODUCT_CONTEXT ( 'NONE', #68669, 'mechanical' ) ;
#114982=CARTESIAN_POINT ( 'NONE',  ( 21.04946095171255394, -10.24435024061060950, 168.3368280404224606 ) ) ;
#114998=ADVANCED_FACE ( 'NONE', ( #143820 ), #162569, .T. ) ;
#115105=CYLINDRICAL_SURFACE ( 'NONE', #173526, 28.79475375365586487 ) ;
#115118=ORIENTED_EDGE ( 'NONE', *, *, #24178, .T. ) ;
#115133=CARTESIAN_POINT ( 'NONE',  ( 24.45434260692612227, 5.907237110200220798, 169.8064932912610345 ) ) ;
#115141=DIRECTION ( 'NONE',  ( 1.000000000000000000, -0.000000000000000000, -0.000000000000000000 ) ) ;
#115174=CARTESIAN_POINT ( 'NONE',  ( 27.18966431762751412, 4.276553394868218838, 168.7322077152536508 ) ) ;
#115288=CARTESIAN_POINT ( 'NONE',  ( 21.36928693577338834, 5.431965077040404211, 174.3311293403526179 ) ) ;
#115404=CARTESIAN_POINT ( 'NONE',  ( 27.73933785331498925, -9.013057229001034898, 143.7750000027311614 ) ) ;
#115459=CARTESIAN_POINT ( 'NONE',  ( 17.81289503416610742, 24.51734667627700404, 139.5500000054623229 ) ) ;
#115472=CARTESIAN_POINT ( 'NONE',  ( -17.14385361876520264, -23.59649016807271238, 145.6750000027311671 ) ) ;
#115545=CARTESIAN_POINT ( 'NONE',  ( -24.06609220500515178, 14.38661408136930575, 165.8682408874382475 ) ) ;
#115588=CARTESIAN_POINT ( 'NONE',  ( 26.73207562759453992, 6.543912086049501475, 168.7462576975894422 ) ) ;
#115624=DIRECTION ( 'NONE',  ( -0.9945218953682734009, 0.000000000000000000, 0.1045284632676537068 ) ) ;
#115627=CARTESIAN_POINT ( 'NONE',  ( 28.79475375365599987, -9.355982642738995381, 144.8843446568999980 ) ) ;
#115808=B_SPLINE_CURVE_WITH_KNOTS ( 'NONE', 3,
 ( #101496, #98490, #114671, #178366, #176367, #20665, #68165, #37840, #116676, #99500, #161181, #146003, #7486, #175356 ),
 .UNSPECIFIED., .F., .F.,
 ( 4, 2, 2, 2, 2, 2, 4 ),
 ( -0.0006136969902427322687, 0.0004464899733162382622, 0.001506676936875208685, 0.003627050863993181839, 0.004687237827552175572, 0.005747424791111170606, 0.007867798718229164143 ),
 .UNSPECIFIED. ) ;
#115865=CARTESIAN_POINT ( 'NONE',  ( 24.99734946672222335, -12.60193342193096555, 166.0696721667194993 ) ) ;
#115870=CARTESIAN_POINT ( 'NONE',  ( -27.19095269391954517, -10.02149780027903780, 149.7954620931811291 ) ) ;
#115880=DIRECTION ( 'NONE',  ( 0.000000000000000000, 0.9945218953682734009, 0.1045284632676537068 ) ) ;
#115900=CARTESIAN_POINT ( 'NONE',  ( 27.96111904526279091, 7.044650443041771126, 161.2906300811259541 ) ) ;
#115985=CARTESIAN_POINT ( 'NONE',  ( 24.30454888808799296, -2.781629622375088928, 174.5654150192188183 ) ) ;
#116133=CARTESIAN_POINT ( 'NONE',  ( 24.71161622716358153, 5.993525217005513994, 168.9855167950506143 ) ) ;
#116191=( NAMED_UNIT ( * ) PLANE_ANGLE_UNIT ( ) SI_UNIT ( $, .RADIAN. ) );
#116192=CARTESIAN_POINT ( 'NONE',  ( 24.81835880841864039, -6.052260367207979996, 168.4265213779230521 ) ) ;
#116212=DIRECTION ( 'NONE',  ( -0.000000000000000000, -1.000000000000000000, -0.000000000000000000 ) ) ;
#116269=CARTESIAN_POINT ( 'NONE',  ( -27.20512408146884908, -7.754361572989796336, 164.3878212768171920 ) ) ;
#116370=CARTESIAN_POINT ( 'NONE',  ( -25.90244409532896697, 6.509810826857618693, 161.8457455760362222 ) ) ;
#116394=CARTESIAN_POINT ( 'NONE',  ( 27.73933785331498569, 2.768321779492822058E-14, 143.8750000027311842 ) ) ;
#116444=AXIS2_PLACEMENT_3D ( 'NONE', #47884, #45887, #109537 ) ;
#116455=CARTESIAN_POINT ( 'NONE',  ( -28.82186960331499392, -9.364793116373526516, 140.3500000054623627 ) ) ;
#116468=CARTESIAN_POINT ( 'NONE',  ( -8.571926809382608425, 26.38167802310805854, 144.9750000027312069 ) ) ;
#116499=DIRECTION ( 'NONE',  ( 1.000000000000000000, 0.000000000000000000, -0.000000000000000000 ) ) ;
#116581=CARTESIAN_POINT ( 'NONE',  ( 20.14845677604831664, 11.85354687992394496, 170.0217845860066745 ) ) ;
#116592=CARTESIAN_POINT ( 'NONE',  ( 17.81289503416611453, -24.51734667627695785, 146.6999999999999886 ) ) ;
#116676=CARTESIAN_POINT ( 'NONE',  ( -25.28116846732003964, 11.97242897402593442, 166.1912472719371863 ) ) ;
#116692=EDGE_CURVE ( 'NONE', #35595, #34840, #190457, .T. ) ;
#116746=CARTESIAN_POINT ( 'NONE',  ( -5.359611314223446995E-15, 29.16686587814335851, 148.3750000027311842 ) ) ;
#116818=ORIENTED_EDGE ( 'NONE', *, *, #42863, .T. ) ;
#116855=CARTESIAN_POINT ( 'NONE',  ( 23.64874990377911246, -15.04272038711346937, 165.8682408883346397 ) ) ;
#116878=ORIENTED_EDGE ( 'NONE', *, *, #33729, .F. ) ;
#116906=ORIENTED_EDGE ( 'NONE', *, *, #75822, .F. ) ;
#116933=CARTESIAN_POINT ( 'NONE',  ( 27.73933785331498214, 9.013057229001095294, 148.4750000027311785 ) ) ;
#116956=VERTEX_POINT ( 'NONE', #166996 ) ;
#116977=CARTESIAN_POINT ( 'NONE',  ( 24.81886791266633097, -6.075537473402710553, 168.3989613422507432 ) ) ;
#117079=B_SPLINE_CURVE_WITH_KNOTS ( 'NONE', 3,
 ( #164012, #93, #198311, #59789, #119495, #122448 ),
 .UNSPECIFIED., .F., .F.,
 ( 4, 2, 4 ),
 ( 0.0003734705499822683190, 0.004296280022385642362, 0.008219089494789017653 ),
 .UNSPECIFIED. ) ;
#117196=EDGE_CURVE ( 'NONE', #82312, #122086, #33382, .T. ) ;
#117207=CARTESIAN_POINT ( 'NONE',  ( -21.38418241377623374, -5.438282248597753110, 174.2683007571264113 ) ) ;
#117374=CARTESIAN_POINT ( 'NONE',  ( -23.29544513554941076, 16.92513159979227666, 141.7843446568999752 ) ) ;
#117452=CARTESIAN_POINT ( 'NONE',  ( -8.906447517083060816, 27.41122689804195645, 141.8500000054623911 ) ) ;
#117466=CARTESIAN_POINT ( 'NONE',  ( -27.73933785331498925, 9.013057229001088189, 143.2750000027311899 ) ) ;
#117537=CARTESIAN_POINT ( 'NONE',  ( -21.84611564451296672, 9.363109600221495299, 171.0247306346272751 ) ) ;
#117578=ORIENTED_EDGE ( 'NONE', *, *, #89522, .F. ) ;
#117579=CARTESIAN_POINT ( 'NONE',  ( 25.62062145120080103, 9.171473787276196887, 171.1688781158127028 ) ) ;
#117590=CARTESIAN_POINT ( 'NONE',  ( 8.906447517083057264, -27.41122689804191026, 148.5999999999999943 ) ) ;
#117602=CLOSED_SHELL ( 'NONE', ( #184481, #38662, #22207, #47032, #64370, #67491, #30330, #45643, #140183, #165578, #191364, #27705, #1779, #13777, #136809, #162076, #92282, #173652, #114127, #129217, #100839, #197994, #89653, #21634, #70806, #42424, #36421, #90878, #153015, #171965, #114998, #127422, #191910, #87717, #156285, #170129, #181717, #154536, #148251, #84984, #42332, #59345, #130630, #88416, #195013, #172668, #133971, #101406, #26137, #127217, #180603, #50685, #108149, #150543, #163464, #101656, #127617, #52761, #83017, #12349, #51269 ) ) ;
#117609=ORIENTED_EDGE ( 'NONE', *, *, #137956, .T. ) ;
#117662=DIRECTION ( 'NONE',  ( 0.000000000000000000, 0.000000000000000000, -1.000000000000000000 ) ) ;
#117671=DIRECTION ( 'NONE',  ( 0.000000000000000000, 0.000000000000000000, -1.000000000000000000 ) ) ;
#117739=CARTESIAN_POINT ( 'NONE',  ( -21.27717364736663797, -9.815017990598716935, 168.4818444780605375 ) ) ;
#117755=CARTESIAN_POINT ( 'NONE',  ( -22.44159573604009950, -16.30477369853688430, 145.0750000027311728 ) ) ;
#117767=DIRECTION ( 'NONE',  ( -0.000000000000000000, -1.000000000000000000, -0.000000000000000000 ) ) ;
#117794=EDGE_CURVE ( 'NONE', #186058, #110081, #172435, .T. ) ;
#117948=CARTESIAN_POINT ( 'NONE',  ( -27.73933785331498925, -9.013057229001049109, 147.4750000027311785 ) ) ;
#117968=ORIENTED_EDGE ( 'NONE', *, *, #84475, .F. ) ;
#117990=CARTESIAN_POINT ( 'NONE',  ( 21.96844466259035400, -7.174710485416647465, 170.3366942299255413 ) ) ;
#118128=CARTESIAN_POINT ( 'NONE',  ( -26.81441202005693114, -10.25421135757314950, 139.9999999999999716 ) ) ;
#118193=CARTESIAN_POINT ( 'NONE',  ( -21.35096542554161658, -10.43949311476039554, 170.3901443614043671 ) ) ;
#118217=CARTESIAN_POINT ( 'NONE',  ( 21.98685479826775335, -13.98560643873835652, 165.5209445330007441 ) ) ;
#118277=CARTESIAN_POINT ( 'NONE',  ( 23.29544513554940366, -16.92513159979222337, 142.7843446568999752 ) ) ;
#118282=CARTESIAN_POINT ( 'NONE',  ( -27.89898386897531068, -7.496946767028572545, 160.9847407630206817 ) ) ;
#118296=CARTESIAN_POINT ( 'NONE',  ( 24.27995301597489686, 6.552671593954989326, 171.1165850637242443 ) ) ;
#118388=CARTESIAN_POINT ( 'NONE',  ( -27.40223502306384873, 7.751740014893099051, 163.3164180876359524 ) ) ;
#118405=DIRECTION ( 'NONE',  ( 1.000000000000000000, 0.000000000000000000, -0.000000000000000000 ) ) ;
#118449=ORIENTED_EDGE ( 'NONE', *, *, #89522, .T. ) ;
#118465=LINE ( 'NONE', #27466, #82184 ) ;
#118466=CARTESIAN_POINT ( 'NONE',  ( 17.14385361876520264, -23.59649016807271238, 147.5750000027311444 ) ) ;
#118480=CARTESIAN_POINT ( 'NONE',  ( 22.44159573604009239, 16.30477369853692693, 142.5750000027311728 ) ) ;
#118500=CIRCLE ( 'NONE', #12003, 27.29906736325805028 ) ;
#118605=CARTESIAN_POINT ( 'NONE',  ( -8.906447517083060816, 27.41122689804195645, 149.5999999999999943 ) ) ;
#118714=B_SPLINE_CURVE_WITH_KNOTS ( 'NONE', 3,
 ( #85017, #116370, #102207, #101186, #21366, #146698, #70875, #69870 ),
 .UNSPECIFIED., .F., .F.,
 ( 4, 2, 2, 4 ),
 ( 0.03534151991400969611, 0.03926041079282524549, 0.04121985623223305140, 0.04317930167164086425 ),
 .UNSPECIFIED. ) ;
#118748=CARTESIAN_POINT ( 'NONE',  ( -19.49401214000074489, -12.39993551617566503, 167.9999999999999716 ) ) ;
#118761=CARTESIAN_POINT ( 'NONE',  ( -27.73933785331498925, 2.428612866367529932E-14, 146.8750000027311842 ) ) ;
#118773=CARTESIAN_POINT ( 'NONE',  ( 24.99788752995426577, 12.60079600866962046, 166.0698618172138481 ) ) ;
#118960=CARTESIAN_POINT ( 'NONE',  ( -3.573655867282028392E-15, 2.428612866367529932E-14, 169.9999999999999716 ) ) ;
#118996=CARTESIAN_POINT ( 'NONE',  ( 23.84827716990776381, -9.022217638662555217, 168.8513102586128696 ) ) ;
#119024=ORIENTED_EDGE ( 'NONE', *, *, #130470, .F. ) ;
#119127=ORIENTED_EDGE ( 'NONE', *, *, #114246, .T. ) ;
#119188=VECTOR ( 'NONE', #171837, 1000.000000000000000 ) ;
#119215=CARTESIAN_POINT ( 'NONE',  ( 22.40075113267181450, -13.33491755757044572, 165.5209445330007441 ) ) ;
#119292=CARTESIAN_POINT ( 'NONE',  ( 21.97054992548844865, 7.027819292989578415, 170.5066066589220100 ) ) ;
#119461=CARTESIAN_POINT ( 'NONE',  ( 8.906447517083057264, -27.41122689804191026, 142.8500000054623911 ) ) ;
#119495=CARTESIAN_POINT ( 'NONE',  ( 25.90238458237720565, 6.509645158105397122, 161.8463118039489643 ) ) ;
#119499=VERTEX_POINT ( 'NONE', #24876 ) ;
#119522=CARTESIAN_POINT ( 'NONE',  ( -29.15849868437705439, -10.00000000000000000, 150.0000000000000000 ) ) ;
#119545=CARTESIAN_POINT ( 'NONE',  ( -26.26139018963108285, 3.005588016160658071, 174.9127113745526572 ) ) ;
#119587=CARTESIAN_POINT ( 'NONE',  ( 21.73861122199407347, 7.688394669363296963, 173.2969830217476499 ) ) ;
#119599=CARTESIAN_POINT ( 'NONE',  ( -8.906447517083053711, -27.41122689804191026, 146.4000000000000057 ) ) ;
#119645=ORIENTED_EDGE ( 'NONE', *, *, #15702, .T. ) ;
#119736=DIRECTION ( 'NONE',  ( 1.000000000000000000, 0.000000000000000000, -0.000000000000000000 ) ) ;
#119883=CARTESIAN_POINT ( 'NONE',  ( 21.71408805923169183, -8.664832797227230543, 169.0754946983649631 ) ) ;
#119935=CARTESIAN_POINT ( 'NONE',  ( 17.14385361876520264, 23.59649016807275856, 144.6750000027311671 ) ) ;
#119973=CARTESIAN_POINT ( 'NONE',  ( -21.84611564451295962, -9.363109600220301587, 171.0247306346281277 ) ) ;
#120075=EDGE_CURVE ( 'NONE', #10845, #181921, #146187, .T. ) ;
#120123=CARTESIAN_POINT ( 'NONE',  ( 25.12473289294614176, -7.795855283352525866, 170.9710361440363329 ) ) ;
#120163=FACE_OUTER_BOUND ( 'NONE', #11300, .T. ) ;
#120183=ORIENTED_EDGE ( 'NONE', *, *, #30184, .T. ) ;
#120192=CARTESIAN_POINT ( 'NONE',  ( 28.79475375365606737, -9.355982642738910116, 146.8843446568999980 ) ) ;
#120271=CARTESIAN_POINT ( 'NONE',  ( 17.14385361876520264, 23.59649016807275856, 144.1750000027311671 ) ) ;
#120353=DIRECTION ( 'NONE',  ( -0.000000000000000000, -1.000000000000000000, -0.000000000000000000 ) ) ;
#120411=ORIENTED_EDGE ( 'NONE', *, *, #125821, .F. ) ;
#120432=CARTESIAN_POINT ( 'NONE',  ( 1.784210473542230573E-15, -29.16686587814331588, 145.3750000027311842 ) ) ;
#120513=CARTESIAN_POINT ( 'NONE',  ( -13.35345327432327878, -24.89324389316316655, 139.9999999999999716 ) ) ;
#120555=CARTESIAN_POINT ( 'NONE',  ( 26.77313074627685197, 4.631999166354653141, 170.7390164845645870 ) ) ;
#120568=CARTESIAN_POINT ( 'NONE',  ( -28.82186960331499037, 2.428612866367529932E-14, 148.0000000000000000 ) ) ;
#120634=VECTOR ( 'NONE', #64407, 1000.000000000000114 ) ;
#120732=FACE_OUTER_BOUND ( 'NONE', #93426, .T. ) ;
#120806=B_SPLINE_CURVE_WITH_KNOTS ( 'NONE', 3,
 ( #155621, #63614, #48457, #172791, #156624, #126273, #67580, #175768, #36239, #160594, #79774, #82736 ),
 .UNSPECIFIED., .F., .F.,
 ( 4, 2, 2, 2, 2, 4 ),
 ( 0.003927129849554318076, 0.005134622258946400924, 0.006342114668338482905, 0.007549607077730566621, 0.008153353282426611948, 0.008757099487122657275 ),
 .UNSPECIFIED. ) ;
#120812=ORIENTED_EDGE ( 'NONE', *, *, #57861, .F. ) ;
#120844=ORIENTED_EDGE ( 'NONE', *, *, #68275, .T. ) ;
#120912=CARTESIAN_POINT ( 'NONE',  ( -17.14385361876520264, -23.59649016807271593, 141.6750000027311103 ) ) ;
#120916=CARTESIAN_POINT ( 'NONE',  ( -17.14385361876520619, 23.59649016807275856, 145.0750000027311728 ) ) ;
#120921=DIRECTION ( 'NONE',  ( 1.000000000000000000, 0.000000000000000000, 0.000000000000000000 ) ) ;
#120953=CARTESIAN_POINT ( 'NONE',  ( -25.75939503182733858, -8.559839547494508594, 171.7912139782359588 ) ) ;
#121123=CARTESIAN_POINT ( 'NONE',  ( -27.73933785331498925, 2.428612866367529932E-14, 148.8750000027311842 ) ) ;
#121139=CARTESIAN_POINT ( 'NONE',  ( 24.13306144861383729, 5.795830589372933161, 190.0000000000000000 ) ) ;
#121159=CARTESIAN_POINT ( 'NONE',  ( -21.96410559793011785, -8.829621495424600397, 171.4826196141302717 ) ) ;
#121173=ORIENTED_EDGE ( 'NONE', *, *, #104106, .F. ) ;
#121237=CARTESIAN_POINT ( 'NONE',  ( 26.58496454516999563, 7.626754437231445749, 167.9682100371138915 ) ) ;
#121263=CARTESIAN_POINT ( 'NONE',  ( 8.571926809382603096, -26.38167802310801235, 145.4750000027311785 ) ) ;
#121350=CARTESIAN_POINT ( 'NONE',  ( -27.79722099587806028, 7.618187661584445713, 161.3616444162223900 ) ) ;
#121425=CARTESIAN_POINT ( 'NONE',  ( -17.14385361876520619, 23.59649016807275856, 142.5750000027312012 ) ) ;
#121462=CARTESIAN_POINT ( 'NONE',  ( 28.79475375365590040, -9.355982642739126831, 140.8843446568999696 ) ) ;
#121474=CARTESIAN_POINT ( 'NONE',  ( 28.79475375365586132, 2.781246896534039337E-14, 155.0000000000000000 ) ) ;
#121505=CARTESIAN_POINT ( 'NONE',  ( 8.545215834362450025, -26.44289320400097409, 139.9999999999999716 ) ) ;
#121561=CARTESIAN_POINT ( 'NONE',  ( -8.906447517083060816, 27.41122689804195645, 141.5999999999999943 ) ) ;
#121660=CARTESIAN_POINT ( 'NONE',  ( -23.91168844458710652, -8.792376985860583360, 168.9858545422750353 ) ) ;
#121718=( BOUNDED_SURFACE ( )  B_SPLINE_SURFACE ( 3, 2, ( 
 ( #30571, #57943, #181297 ),
 ( #166121, #89262, #150954 ),
 ( #12448, #74110, #135780 ),
 ( #136749, #4186, #174067 ),
 ( #5182, #1204, #48729 ),
 ( #97183, #94214, #156900 ),
 ( #112375, #95214, #128526 ),
 ( #18396, #66863, #3206 ),
 ( #110383, #127537, #20358 ),
 ( #186259, #126541, #172065 ),
 ( #80047, #81031, #190220 ),
 ( #108398, #33552, #158869 ),
 ( #47737, #173068, #17391 ),
 ( #50717, #170075, #31566 ),
 ( #109390, #155893, #82006 ),
 ( #140721, #34545, #189239 ),
 ( #96204, #141716, #65865 ),
 ( #62881, #19382, #124562 ),
 ( #64880, #187260, #188240 ),
 ( #157893, #2211, #93217 ),
 ( #35536, #49715, #125563 ),
 ( #111380, #154902, #142707 ),
 ( #16401, #143700, #78047 ),
 ( #139716, #171070, #32560 ) ),
 .UNSPECIFIED., .F., .F., .F. ) 
 B_SPLINE_SURFACE_WITH_KNOTS ( ( 4, 2, 2, 2, 2, 2, 2, 2, 2, 2, 2, 4 ),
 ( 3, 3 ),
 ( 0.000000000000000000, 0.001899702839891691426, 0.002849554259837537139, 0.003799405679783382853, 0.005699108519675074279, 0.006648959939620920426, 0.007598811359566765705, 0.008548662779512610985, 0.009498514199458456264, 0.01139821703935014856, 0.01329791987924184085, 0.01519762271913353141 ),
 ( 0.000000000000000000, 1.000000000000000000 ),
 .UNSPECIFIED. ) 
 GEOMETRIC_REPRESENTATION_ITEM ( )  RATIONAL_B_SPLINE_SURFACE ( (
 ( 1.000000000000000000, 0.7660444431189777914, 1.000000000000000000),
 ( 1.000000000000000000, 0.7753720600381861505, 1.000000000000000000),
 ( 1.000000000000000000, 0.7832595754286625356, 1.000000000000000000),
 ( 1.000000000000000000, 0.7928595458705119947, 1.000000000000000000),
 ( 1.000000000000000000, 0.7956872332516093937, 1.000000000000000000),
 ( 1.000000000000000000, 0.8005750596157590326, 1.000000000000000000),
 ( 1.000000000000000000, 0.8026302056541338992, 1.000000000000000000),
 ( 1.000000000000000000, 0.8075080643849141815, 1.000000000000000000),
 ( 1.000000000000000000, 0.8091143015809389993, 1.000000000000000000),
 ( 1.000000000000000000, 0.8093067629633259319, 1.000000000000000000),
 ( 1.000000000000000000, 0.8089952915731264405, 1.000000000000000000),
 ( 1.000000000000000000, 0.8076919994862710173, 1.000000000000000000),
 ( 1.000000000000000000, 0.8067078407648710092, 1.000000000000000000),
 ( 1.000000000000000000, 0.8041786842467625318, 1.000000000000000000),
 ( 1.000000000000000000, 0.8026334674876911546, 1.000000000000000000),
 ( 1.000000000000000000, 0.7990747329469507498, 1.000000000000000000),
 ( 1.000000000000000000, 0.7970509760941782984, 1.000000000000000000),
 ( 1.000000000000000000, 0.7904793850863390814, 1.000000000000000000),
 ( 1.000000000000000000, 0.7855040224314148167, 1.000000000000000000),
 ( 1.000000000000000000, 0.7751942650507165355, 1.000000000000000000),
 ( 1.000000000000000000, 0.7698260778210667121, 1.000000000000000000),
 ( 1.000000000000000000, 0.7598259884961829913, 1.000000000000000000),
 ( 1.000000000000000000, 0.7551428682219649691, 1.000000000000000000),
 ( 1.000000000000000000, 0.7510191126010862250, 1.000000000000000000) ) ) 
 REPRESENTATION_ITEM ( '' )  SURFACE ( )  );
#121753=FACE_OUTER_BOUND ( 'NONE', #193218, .T. ) ;
#121851=EDGE_CURVE ( 'NONE', #122599, #68306, #129233, .T. ) ;
#121909=CARTESIAN_POINT ( 'NONE',  ( 8.571926809382603096, -26.38167802310801235, 141.9750000027312069 ) ) ;
#121913=CARTESIAN_POINT ( 'NONE',  ( -22.44159573604010305, 16.30477369853692338, 145.1750000027311671 ) ) ;
#121938=AXIS2_PLACEMENT_3D ( 'NONE', #43344, #182859, #139316 ) ;
#121950=CARTESIAN_POINT ( 'NONE',  ( -19.49401214000074489, -12.39993551617566325, 169.9999999999999716 ) ) ;
#121993=EDGE_CURVE ( 'NONE', #109599, #131044, #27282, .T. ) ;
#122086=VERTEX_POINT ( 'NONE', #69116 ) ;
#122100=CARTESIAN_POINT ( 'NONE',  ( -7.950080215733696498, 27.42129086533356030, 140.0000000000000284 ) ) ;
#122150=CARTESIAN_POINT ( 'NONE',  ( -20.74358237093910162, 11.24271120488109865, 170.1279846108370180 ) ) ;
#122163=CARTESIAN_POINT ( 'NONE',  ( -28.79475375365586842, 2.428612866367529932E-14, 145.9843446568999923 ) ) ;
#122252=CARTESIAN_POINT ( 'NONE',  ( -22.44159573604009950, -16.30477369853688430, 147.0750000027312012 ) ) ;
#122309=CARTESIAN_POINT ( 'NONE',  ( 24.81835718235489807, 6.052279806424484931, 168.4265042179603142 ) ) ;
#122378=DIRECTION ( 'NONE',  ( -1.000000000000000000, 0.000000000000000000, 0.000000000000000000 ) ) ;
#122416=CARTESIAN_POINT ( 'NONE',  ( 22.44159573604009239, 16.30477369853692693, 146.0750000027311728 ) ) ;
#122448=CARTESIAN_POINT ( 'NONE',  ( 26.03370437638686852, 6.875205692009825675, 160.5968874236875195 ) ) ;
#122497=CARTESIAN_POINT ( 'NONE',  ( -2.002489259400932919, -27.92993298909506095, 139.9999999999999716 ) ) ;
#122542=VERTEX_POINT ( 'NONE', #150971 ) ;
#122545=ORIENTED_EDGE ( 'NONE', *, *, #31673, .F. ) ;
#122556=CARTESIAN_POINT ( 'NONE',  ( -28.82186960331499037, 2.428612866367529932E-14, 144.0000000000000000 ) ) ;
#122568=DIRECTION ( 'NONE',  ( 0.000000000000000000, 0.000000000000000000, -1.000000000000000000 ) ) ;
#122599=VERTEX_POINT ( 'NONE', #74126 ) ;
#122655=CARTESIAN_POINT ( 'NONE',  ( -24.22576942085221674, -7.195495839723525577, 170.3116806589360124 ) ) ;
#122892=ORIENTED_EDGE ( 'NONE', *, *, #97731, .F. ) ;
#122899=CARTESIAN_POINT ( 'NONE',  ( 27.73933785331498925, -9.013057229001033122, 144.2750000027311899 ) ) ;
#122903=CARTESIAN_POINT ( 'NONE',  ( 8.571926809382597767, 26.38167802310806209, 144.7750000027311899 ) ) ;
#122939=CARTESIAN_POINT ( 'NONE',  ( -21.94905633995418270, -8.886455535326843957, 171.4390084046468132 ) ) ;
#122945=EDGE_CURVE ( 'NONE', #70413, #46062, #13079, .T. ) ;
#122987=EDGE_CURVE ( 'NONE', #68306, #139247, #35161, .T. ) ;
#123107=CARTESIAN_POINT ( 'NONE',  ( 17.79613651744294245, -24.49428055684527550, 144.9656553485623647 ) ) ;
#123180=CARTESIAN_POINT ( 'NONE',  ( -22.72581825106501796, 12.75361973299702534, 165.5645137041830139 ) ) ;
#123217=PLANE ( 'NONE',  #193971 ) ;
#123240=CARTESIAN_POINT ( 'NONE',  ( 17.14385361876520264, 23.59649016807275856, 146.1750000027311387 ) ) ;
#123261=AXIS2_PLACEMENT_3D ( 'NONE', #51553, #143548, #114204 ) ;
#123322=DIRECTION ( 'NONE',  ( -1.000000000000000000, 0.000000000000000000, 0.000000000000000000 ) ) ;
#123401=CARTESIAN_POINT ( 'NONE',  ( 27.73933785331498925, -9.013057229001033122, 141.7750000027311899 ) ) ;
#123446=DIRECTION ( 'NONE',  ( 0.5367108174878536531, -0.8437662581494473901, 0.000000000000000000 ) ) ;
#123538=EDGE_CURVE ( 'NONE', #69189, #184349, #124086, .T. ) ;
#123539=CARTESIAN_POINT ( 'NONE',  ( 23.31738231874054890, -16.94106989632523508, 142.7999999999999829 ) ) ;
#123561=CARTESIAN_POINT ( 'NONE',  ( 0.000000000000000000, -3.784814030245899019, 190.0000000000000000 ) ) ;
#123570=CARTESIAN_POINT ( 'NONE',  ( -28.79475375365586842, 2.428612866367529932E-14, 155.0000000000000000 ) ) ;
#123634=CARTESIAN_POINT ( 'NONE',  ( -21.96844466259036111, -7.174710485412877148, 170.3366942299294635 ) ) ;
#123722=DIRECTION ( 'NONE',  ( -0.1039620511844979306, -0.1039620511844979306, 0.9891328443778538704 ) ) ;
#123724=CARTESIAN_POINT ( 'NONE',  ( -27.88129983271673851, -6.733757357603135318, 162.1517353552107750 ) ) ;
#123796=FACE_OUTER_BOUND ( 'NONE', #50236, .T. ) ;
#123883=CARTESIAN_POINT ( 'NONE',  ( -17.14385361876520264, -23.59649016807271593, 145.6750000027311671 ) ) ;
#123887=CARTESIAN_POINT ( 'NONE',  ( 27.73933785331498925, -9.013057229001033122, 148.2750000027311330 ) ) ;
#123921=CARTESIAN_POINT ( 'NONE',  ( -21.95653654802831412, -8.266568072468361450, 172.1684357517875412 ) ) ;
#124079=CARTESIAN_POINT ( 'NONE',  ( -5.222609727149285952, 28.09897361876272726, 140.0000000000000284 ) ) ;
#124086=( BOUNDED_CURVE ( )  B_SPLINE_CURVE ( 2, ( #136752, #32564, #198436, #59909, #187264, #48733, #31570, #93221, #216, #16405, #185250 ),
 .UNSPECIFIED., .F., .T. ) 
 B_SPLINE_CURVE_WITH_KNOTS ( ( 3, 2, 2, 2, 2, 3 ),
 ( 0.4000000000000031308, 0.4200000000000030931, 0.4400000000000031664, 0.4600000000000031841, 0.4800000000000032019, 0.5000000000000032196 ),
 .UNSPECIFIED. ) 
 CURVE ( )  GEOMETRIC_REPRESENTATION_ITEM ( )  RATIONAL_B_SPLINE_CURVE ( ( 0.9999999999999923395, 0.9510565162951611917, 1.000000000000000000, 0.9510565162951535312, 1.000000000000000000, 0.9510565162951535312, 1.000000000000000000, 0.9510565162951535312, 1.000000000000000000, 0.9510565162951456486, 1.000000000000007772 ) ) 
 REPRESENTATION_ITEM ( '' )  );
#124110=CARTESIAN_POINT ( 'NONE',  ( -24.39440776506090458, -8.562465606919657191, 166.7298475161185252 ) ) ;
#124148=DIRECTION ( 'NONE',  ( -0.000000000000000000, 1.000000000000000000, -0.000000000000000000 ) ) ;
#124170=VECTOR ( 'NONE', #98032, 1000.000000000000000 ) ;
#124173=CARTESIAN_POINT ( 'NONE',  ( -24.27957997113400879, 6.290849861785950736, 171.5443985711291077 ) ) ;
#124243=CARTESIAN_POINT ( 'NONE',  ( -27.73933785331498925, -9.013057229001049109, 146.9750000027311785 ) ) ;
#124280=FACE_BOUND ( 'NONE', #56704, .T. ) ;
#124375=CARTESIAN_POINT ( 'NONE',  ( -17.79613651744294600, 24.49428055684532524, 149.6843446568999809 ) ) ;
#124410=CARTESIAN_POINT ( 'NONE',  ( -27.12243378312306064, 3.972435522077925718, 169.3718635229811298 ) ) ;
#124495=AXIS2_PLACEMENT_3D ( 'NONE', #142063, #151547, #126887 ) ;
#124540=CARTESIAN_POINT ( 'NONE',  ( -22.98342225928958982, -7.557218236066893802, 173.2415159841883394 ) ) ;
#124549=CARTESIAN_POINT ( 'NONE',  ( 28.82186960331498327, 9.364793116373570925, 145.1000000000000227 ) ) ;
#124562=CARTESIAN_POINT ( 'NONE',  ( 21.95653654802608301, -8.266568072468363226, 172.1684357517875412 ) ) ;
#124568=CARTESIAN_POINT ( 'NONE',  ( 21.94207162742805650, -8.184381772639680364, 172.2902002187019832 ) ) ;
#124663=CARTESIAN_POINT ( 'NONE',  ( -17.14385361876520264, -23.59649016807271238, 147.6750000027311671 ) ) ;
#124720=EDGE_CURVE ( 'NONE', #107790, #33383, #80051, .T. ) ;
#124835=ORIENTED_EDGE ( 'NONE', *, *, #32424, .T. ) ;
#124903=CARTESIAN_POINT ( 'NONE',  ( -22.44159573604010305, 16.30477369853692338, 147.1750000027311671 ) ) ;
#124908=CARTESIAN_POINT ( 'NONE',  ( 24.93942350307310107, -7.769968609432603479, 171.2173313942149377 ) ) ;
#124938=CARTESIAN_POINT ( 'NONE',  ( -26.45763050569073727, -3.219288925402985946, 173.6696415116520882 ) ) ;
#124946=EDGE_CURVE ( 'NONE', #87433, #116956, #20362, .T. ) ;
#125045=CARTESIAN_POINT ( 'NONE',  ( 25.25560589046783022, 4.310829775027161581, 167.9999999999999716 ) ) ;
#125188=CARTESIAN_POINT ( 'NONE',  ( -24.68411608548793268, 7.148172978119906595, 167.5704058020754701 ) ) ;
#125246=CARTESIAN_POINT ( 'NONE',  ( 21.35096542554163079, 10.43949311476039554, 170.3901443614043671 ) ) ;
#125251=CARTESIAN_POINT ( 'NONE',  ( -22.44159573604009950, -16.30477369853688430, 139.0750000027311728 ) ) ;
#125289=DIRECTION ( 'NONE',  ( 0.5367108174878537641, 0.8437662581494472791, -0.000000000000000000 ) ) ;
#125324=ORIENTED_EDGE ( 'NONE', *, *, #173096, .F. ) ;
#125329=CARTESIAN_POINT ( 'NONE',  ( -17.79613651744294600, 24.49428055684532524, 143.6843446569000093 ) ) ;
#125336=CARTESIAN_POINT ( 'NONE',  ( -28.79475375365586842, 2.428612866367529932E-14, 155.0000000000000000 ) ) ;
#125338=DIRECTION ( 'NONE',  ( -0.000000000000000000, -0.000000000000000000, -1.000000000000000000 ) ) ;
#125392=DIRECTION ( 'NONE',  ( 0.9945218953682734009, 0.000000000000000000, 0.1045284632676537068 ) ) ;
#125414=CARTESIAN_POINT ( 'NONE',  ( -8.571926809382608425, 26.38167802310805854, 140.4750000027312069 ) ) ;
#125421=CARTESIAN_POINT ( 'NONE',  ( 19.83802472612679324, -12.02135855755840232, 167.9999999999999716 ) ) ;
#125504=EDGE_CURVE ( 'NONE', #122086, #162114, #72, .T. ) ;
#125550=CARTESIAN_POINT ( 'NONE',  ( -17.81289503416611097, -24.51734667627696496, 142.2999999999999829 ) ) ;
#125563=CARTESIAN_POINT ( 'NONE',  ( 21.73861122199297569, -7.688394669363299627, 173.2969830217476215 ) ) ;
#125643=CARTESIAN_POINT ( 'NONE',  ( 17.81289503416610742, 24.51734667627700404, 145.5500000054623513 ) ) ;
#125658=CARTESIAN_POINT ( 'NONE',  ( -22.44159573604010305, 16.30477369853692338, 149.1750000027311671 ) ) ;
#125821=EDGE_CURVE ( 'NONE', #35378, #181866, #74862, .T. ) ;
#125841=CARTESIAN_POINT ( 'NONE',  ( -3.573655867282028392E-15, 2.428612866367529932E-14, 167.9999999999999716 ) ) ;
#125947=CARTESIAN_POINT ( 'NONE',  ( 17.79613651744294245, -24.49428055684527550, 140.9656553485623363 ) ) ;
#125997=EDGE_CURVE ( 'NONE', #63582, #88085, #193503, .T. ) ;
#126148=ORIENTED_EDGE ( 'NONE', *, *, #120075, .F. ) ;
#126173=CARTESIAN_POINT ( 'NONE',  ( -20.14845677604832375, 11.63499142542279152, 168.0304984204094296 ) ) ;
#126233=CARTESIAN_POINT ( 'NONE',  ( 21.96410559793011075, 8.829621495424600397, 171.4826196141302717 ) ) ;
#126238=CARTESIAN_POINT ( 'NONE',  ( 22.44159573604009239, 16.30477369853692693, 140.0750000027311728 ) ) ;
#126273=CARTESIAN_POINT ( 'NONE',  ( 22.98342225928956850, 7.557218236066892914, 173.2415159841882542 ) ) ;
#126275=DIRECTION ( 'NONE',  ( -0.9945218953682734009, 0.000000000000000000, 0.1045284632676530684 ) ) ;
#126364=CARTESIAN_POINT ( 'NONE',  ( -8.898068258721474777, 27.38543819252877043, 149.5843446568999866 ) ) ;
#126461=CARTESIAN_POINT ( 'NONE',  ( 22.72581825106501086, 12.75361973299702001, 165.5645137041830139 ) ) ;
#126480=EDGE_CURVE ( 'NONE', #131506, #31781, #114113, .T. ) ;
#126541=CARTESIAN_POINT ( 'NONE',  ( 25.27727188472196573, -10.29814791481116920, 170.4127952078933674 ) ) ;
#126552=CARTESIAN_POINT ( 'NONE',  ( 24.43796699203919331, -7.704306453272278254, 171.8420650787744250 ) ) ;
#126554=CARTESIAN_POINT ( 'NONE',  ( 24.55187747166651135, 5.935858836270472949, 169.5341757581197157 ) ) ;
#126619=CARTESIAN_POINT ( 'NONE',  ( -17.81289503416611808, 24.51734667627700404, 147.9500000054623570 ) ) ;
#126623=VERTEX_POINT ( 'NONE', #18165 ) ;
#126678=CARTESIAN_POINT ( 'NONE',  ( 17.79613651744293534, 24.49428055684532524, 147.5656553485623306 ) ) ;
#126801=ORIENTED_EDGE ( 'NONE', *, *, #21058, .F. ) ;
#126887=DIRECTION ( 'NONE',  ( 0.000000000000000000, 0.1045284632676537068, 0.9945218953682734009 ) ) ;
#127150=CARTESIAN_POINT ( 'NONE',  ( -21.73861122199408058, 5.803778330637469729, 172.6157762304496828 ) ) ;
#127214=CARTESIAN_POINT ( 'NONE',  ( -27.73933785331498925, 2.428612866367529932E-14, 138.8750000027311842 ) ) ;
#127217=ADVANCED_FACE ( 'NONE', ( #2068 ), #166648, .F. ) ;
#127253=CARTESIAN_POINT ( 'NONE',  ( -17.79613651744293890, -24.49428055684528260, 146.5656553485623306 ) ) ;
#127255=CARTESIAN_POINT ( 'NONE',  ( -28.79475375365586842, 2.428612866367529932E-14, 147.9843446568999923 ) ) ;
#127304=DIRECTION ( 'NONE',  ( -1.000000000000000000, 0.000000000000000000, -0.000000000000000000 ) ) ;
#127326=CARTESIAN_POINT ( 'NONE',  ( -3.573655867282028392E-15, 2.428612866367529932E-14, 155.0000000000000000 ) ) ;
#127353=( LENGTH_UNIT ( ) NAMED_UNIT ( * ) SI_UNIT ( .MILLI., .METRE. ) );
#127384=CARTESIAN_POINT ( 'NONE',  ( -28.79475375365586487, 2.428612866367529932E-14, 149.9843446568999923 ) ) ;
#127422=ADVANCED_FACE ( 'NONE', ( #70482 ), #165459, .T. ) ;
#127450=CARTESIAN_POINT ( 'NONE',  ( 20.56371838171434874, 11.04494471775294961, 168.1294998094270454 ) ) ;
#127537=CARTESIAN_POINT ( 'NONE',  ( 25.04733094907550850, -10.92720321514008575, 170.1247377027657421 ) ) ;
#127617=ADVANCED_FACE ( 'NONE', ( #18762 ), #50092, .F. ) ;
#127619=CARTESIAN_POINT ( 'NONE',  ( -23.31738231874055600, 16.94106989632528837, 144.0500000054623513 ) ) ;
#127632=CARTESIAN_POINT ( 'NONE',  ( 8.571926809382597767, 26.38167802310806209, 148.7750000027311899 ) ) ;
#127655=DIRECTION ( 'NONE',  ( 1.000000000000000000, 0.000000000000000000, 0.000000000000000000 ) ) ;
#127698=CYLINDRICAL_SURFACE ( 'NONE', #105122, 2.000000000000001776 ) ;
#127744=EDGE_LOOP ( 'NONE', ( #183099, #18037, #50170, #19178 ) ) ;
#127867=CARTESIAN_POINT ( 'NONE',  ( -22.68041372103478182, 7.529096845820648198, 173.5090731399504875 ) ) ;
#128029=DIRECTION ( 'NONE',  ( 1.000000000000000000, -0.000000000000000000, -0.000000000000000000 ) ) ;
#128059=CARTESIAN_POINT ( 'NONE',  ( 27.88129983271499768, 6.733757357597986548, 162.1517353552272880 ) ) ;
#128084=CARTESIAN_POINT ( 'NONE',  ( -24.81835880841865816, 6.052260367207988878, 168.4265213779230521 ) ) ;
#128210=CARTESIAN_POINT ( 'NONE',  ( 21.49230439284897187, 7.461675232480832420, 174.1505469413571348 ) ) ;
#128249=CARTESIAN_POINT ( 'NONE',  ( -28.79475375365672107, -9.355982642738018384, 146.3656553485623419 ) ) ;
#128298=LINE ( 'NONE', #113134, #53356 ) ;
#128335=FACE_OUTER_BOUND ( 'NONE', #10034, .T. ) ;
#128348=EDGE_LOOP ( 'NONE', ( #65907, #44036 ) ) ;
#128378=CARTESIAN_POINT ( 'NONE',  ( 27.73933785331498925, -9.013057229001033122, 139.7750000027311899 ) ) ;
#128411=CARTESIAN_POINT ( 'NONE',  ( 24.04960827311052540, -5.809912860844005600, 170.7323280178997891 ) ) ;
#128439=CARTESIAN_POINT ( 'NONE',  ( 20.69372460268669300, 10.84650605405351875, 168.1714143675832247 ) ) ;
#128505=CARTESIAN_POINT ( 'NONE',  ( -26.58496454517000629, 7.626754437231443084, 167.9682100371138915 ) ) ;
#128526=CARTESIAN_POINT ( 'NONE',  ( 21.04946095171200326, -10.86023174791519530, 170.2405914574445092 ) ) ;
#128554=EDGE_LOOP ( 'NONE', ( #48184, #16957 ) ) ;
#128556=B_SPLINE_CURVE_WITH_KNOTS ( 'NONE', 3,
 ( #146031, #50058, #127867, #5520, #54040, #4514, #18727, #67200 ),
 .UNSPECIFIED., .F., .F.,
 ( 4, 2, 2, 4 ),
 ( -1.451984513602681931E-05, 0.002415095736453747293, 0.003629903527248607049, 0.004844711318043467239 ),
 .UNSPECIFIED. ) ;
#128601=EDGE_LOOP ( 'NONE', ( #171404, #69312, #80550, #124835 ) ) ;
#128607=CARTESIAN_POINT ( 'NONE',  ( -27.73933785331498925, 2.428612866367529932E-14, 139.3750000027311842 ) ) ;
#128608=CARTESIAN_POINT ( 'NONE',  ( 23.31738231874054534, 16.94106989632529192, 143.4500000054623854 ) ) ;
#128622=CARTESIAN_POINT ( 'NONE',  ( 27.73933785331498569, 2.768321779492822058E-14, 148.3750000027311842 ) ) ;
#128649=CARTESIAN_POINT ( 'NONE',  ( -3.573655867282028392E-15, 2.428612866367529932E-14, 169.9999999999999716 ) ) ;
#128668=CARTESIAN_POINT ( 'NONE',  ( 23.29544513554940011, 16.92513159979228021, 147.4656553485623647 ) ) ;
#128695=CARTESIAN_POINT ( 'NONE',  ( 28.79475375365586132, 2.781246896534039337E-14, 143.2656553485623760 ) ) ;
#128734=CARTESIAN_POINT ( 'NONE',  ( 25.27727188472143283, 10.29814791481116032, 170.4127952078933674 ) ) ;
#128830=CARTESIAN_POINT ( 'NONE',  ( -21.53032740501643261, 19.35460773160097503, 140.0335582641266683 ) ) ;
#128851=CARTESIAN_POINT ( 'NONE',  ( 26.03370437638690049, -6.875205692009868308, 160.5968874236871784 ) ) ;
#128891=CARTESIAN_POINT ( 'NONE',  ( -21.56952297831670151, -7.512152360717307964, 173.9007003117370971 ) ) ;
#128968=ORIENTED_EDGE ( 'NONE', *, *, #192109, .T. ) ;
#129179=CARTESIAN_POINT ( 'NONE',  ( 23.42531391676913088, 11.30614932247368642, 165.8025715494068493 ) ) ;
#129197=CARTESIAN_POINT ( 'NONE',  ( 21.16473053983487418, 10.71450305990368967, 170.2845851188453992 ) ) ;
#129214=CARTESIAN_POINT ( 'NONE',  ( -28.79475375365586842, 2.428612866367529932E-14, 142.2656553485623760 ) ) ;
#129217=ADVANCED_FACE ( 'NONE', ( #54825 ), #164021, .T. ) ;
#129233=CIRCLE ( 'NONE', #51740, 25.62086810090349331 ) ;
#129321=AXIS2_PLACEMENT_3D ( 'NONE', #170322, #78291, #140968 ) ;
#129348=ORIENTED_EDGE ( 'NONE', *, *, #131623, .F. ) ;
#129381=DIRECTION ( 'NONE',  ( 0.000000000000000000, 0.000000000000000000, 1.000000000000000000 ) ) ;
#129541=CARTESIAN_POINT ( 'NONE',  ( -5.359611314223446995E-15, 29.16686587814335851, 140.3750000027311842 ) ) ;
#129596=CARTESIAN_POINT ( 'NONE',  ( -27.73933785331498925, -9.013057229001049109, 139.4750000027311785 ) ) ;
#129597=CARTESIAN_POINT ( 'NONE',  ( -8.906447517083060816, 27.41122689804195645, 145.8500000054623627 ) ) ;
#129611=CARTESIAN_POINT ( 'NONE',  ( -5.359611314223446995E-15, 29.16686587814335851, 140.8750000027311842 ) ) ;
#129679=CARTESIAN_POINT ( 'NONE',  ( -26.77293948118379063, 6.014770499723010033, 169.2063755025576199 ) ) ;
#129722=CARTESIAN_POINT ( 'NONE',  ( 25.11239783071223997, 12.35465959875007336, 166.1131185557730987 ) ) ;
#129726=CARTESIAN_POINT ( 'NONE',  ( -26.03370437638690049, -6.875205692009850544, 160.5968874236872637 ) ) ;
#129749=ORIENTED_EDGE ( 'NONE', *, *, #117794, .T. ) ;
#129756=DIRECTION ( 'NONE',  ( 0.1045284632676537068, 0.000000000000000000, 0.9945218953682734009 ) ) ;
#129759=CARTESIAN_POINT ( 'NONE',  ( -28.79475375365586842, 2.428612866367529932E-14, 143.9843446568999923 ) ) ;
#130005=CARTESIAN_POINT ( 'NONE',  ( -29.15849868437705439, -7.427326039334300134, 174.4773576836617224 ) ) ;
#130035=CARTESIAN_POINT ( 'NONE',  ( 27.96625882250224393, 7.271219613198154796, 160.9431592986539101 ) ) ;
#130126=CARTESIAN_POINT ( 'NONE',  ( 24.02130208662952171, -8.352503713170980504, 169.2769999910312890 ) ) ;
#130150=ORIENTED_EDGE ( 'NONE', *, *, #177902, .T. ) ;
#130171=CARTESIAN_POINT ( 'NONE',  ( 24.75981411741738825, 6.635778407391001110, 167.9383864321132194 ) ) ;
#130208=CARTESIAN_POINT ( 'NONE',  ( 27.95290315088917055, -7.353483241874310572, 160.8982923760598567 ) ) ;
#130276=CARTESIAN_POINT ( 'NONE',  ( 21.77012268028601483, 5.483007391791947072, 173.8427694445095426 ) ) ;
#130305=CARTESIAN_POINT ( 'NONE',  ( -3.573655867282028392E-15, -12.39993551617566503, 175.0000000000000000 ) ) ;
#130361=AXIS2_PLACEMENT_3D ( 'NONE', #198724, #60191, #74390 ) ;
#130367=CYLINDRICAL_SURFACE ( 'NONE', #110416, 28.79475375365586487 ) ;
#130432=CARTESIAN_POINT ( 'NONE',  ( 24.24385185424126377, 7.025880200331397596, 170.5073520790474788 ) ) ;
#130470=EDGE_CURVE ( 'NONE', #100463, #105726, #35301, .T. ) ;
#130537=AXIS2_PLACEMENT_3D ( 'NONE', #16059, #156558, #865 ) ;
#130608=CARTESIAN_POINT ( 'NONE',  ( -22.44159573604010305, 16.30477369853692338, 148.6750000027311671 ) ) ;
#130621=CARTESIAN_POINT ( 'NONE',  ( 27.73933785331498925, -9.013057229001034898, 144.2750000027311899 ) ) ;
#130630=ADVANCED_FACE ( 'NONE', ( #74976 ), #73009, .F. ) ;
#130693=CARTESIAN_POINT ( 'NONE',  ( -27.19095269391954517, -8.032454009542490780, 149.5864051666458181 ) ) ;
#130694=CARTESIAN_POINT ( 'NONE',  ( -21.97054992548845576, 8.562709642470919036, 171.7904333278019351 ) ) ;
#130739=CARTESIAN_POINT ( 'NONE',  ( 23.03403192006594224, 14.65170476119024201, 169.9999999999999716 ) ) ;
#131019=B_SPLINE_CURVE_WITH_KNOTS ( 'NONE', 3,
 ( #106154, #149691, #167836, #122309 ),
 .UNSPECIFIED., .F., .F.,
 ( 4, 4 ),
 ( 0.000000000000000000, 0.007966001190080656408 ),
 .UNSPECIFIED. ) ;
#131020=CARTESIAN_POINT ( 'NONE',  ( 26.00011078373264795, -10.07146799416501359, 166.7325096689061752 ) ) ;
#131044=VERTEX_POINT ( 'NONE', #101 ) ;
#131083=CARTESIAN_POINT ( 'NONE',  ( -24.79445753310783473, -6.337991946471490223, 168.1742925226654393 ) ) ;
#131100=CARTESIAN_POINT ( 'NONE',  ( 8.571926809382603096, -26.38167802310801235, 147.9750000027311785 ) ) ;
#131106=CARTESIAN_POINT ( 'NONE',  ( -23.46037622756033869, -10.21219847193828123, 168.3031241911537847 ) ) ;
#131132=AXIS2_PLACEMENT_3D ( 'NONE', #6543, #82380, #7543 ) ;
#131190=CARTESIAN_POINT ( 'NONE',  ( 23.27014042476076838, 11.64952740454485713, 165.7333935355015342 ) ) ;
#131228=CARTESIAN_POINT ( 'NONE',  ( 27.83964505791056254, -7.578386611925591154, 161.1890226338703940 ) ) ;
#131387=FACE_OUTER_BOUND ( 'NONE', #40329, .T. ) ;
#131448=CARTESIAN_POINT ( 'NONE',  ( 24.81886791266634162, 6.075537473402705224, 168.3989613422507432 ) ) ;
#131506=VERTEX_POINT ( 'NONE', #121123 ) ;
#131559=CARTESIAN_POINT ( 'NONE',  ( -23.84755066337005758, -5.771293611162919390, 171.0999092862842303 ) ) ;
#131621=CARTESIAN_POINT ( 'NONE',  ( -8.906447517083053711, -27.41122689804191026, 140.6500000054623740 ) ) ;
#131623=EDGE_CURVE ( 'NONE', #131044, #69189, #47565, .T. ) ;
#131635=CARTESIAN_POINT ( 'NONE',  ( 27.73933785331498925, -9.013057229001034898, 142.2750000027311899 ) ) ;
#131694=CARTESIAN_POINT ( 'NONE',  ( -28.79475375365586842, 2.428612866367529932E-14, 141.9843446568999923 ) ) ;
#131708=CARTESIAN_POINT ( 'NONE',  ( -25.41223161463592106, 11.66315983254869693, 166.2610598689586254 ) ) ;
#131750=CARTESIAN_POINT ( 'NONE',  ( 26.13941622279051558, 9.616497135380347672, 166.9083969906205311 ) ) ;
#131752=VERTEX_POINT ( 'NONE', #166659 ) ;
#131762=CARTESIAN_POINT ( 'NONE',  ( -22.44159573604009950, -16.30477369853688430, 139.5750000027311728 ) ) ;
#131784=CIRCLE ( 'NONE', #41310, 28.79475375365586487 ) ;
#131830=DIRECTION ( 'NONE',  ( -0.1039620511844979306, 0.1039620511844979306, -0.9891328443778538704 ) ) ;
#131908=CARTESIAN_POINT ( 'NONE',  ( -21.97143472835162825, -7.273127645264535701, 170.2116391040481176 ) ) ;
#131931=CARTESIAN_POINT ( 'NONE',  ( 24.84792715949108199, 12.91290060751520130, 166.0205615092970106 ) ) ;
#132080=ORIENTED_EDGE ( 'NONE', *, *, #99048, .F. ) ;
#132105=CARTESIAN_POINT ( 'NONE',  ( -8.571926809382601320, -26.38167802310801591, 147.7750000027311899 ) ) ;
#132248=B_SPLINE_CURVE_WITH_KNOTS ( 'NONE', 3,
 ( #7935, #69618, #179818, #39280, #102950, #100937, #101952, #9956, #194972, #164634, #11963, #73628, #198948, #60415, #106919, #12945, #151457, #59421, #165630, #27128, #150468, #72626 ),
 .UNSPECIFIED., .F., .F.,
 ( 4, 2, 2, 2, 2, 2, 2, 2, 2, 2, 4 ),
 ( 0.000000000000000000, 0.001361773908209231061, 0.002042660862313851362, 0.002723547816418472097, 0.004085321724627708796, 0.004766208678732329965, 0.005447095632836950266, 0.006808869541046243777, 0.008170643449255537288, 0.009532417357464831667, 0.01089419126567412605 ),
 .UNSPECIFIED. ) ;
#132288=CARTESIAN_POINT ( 'NONE',  ( -28.67965155328242233, -2.583289564940497218, 139.9999999999999716 ) ) ;
#132403=CARTESIAN_POINT ( 'NONE',  ( -3.573655867282028392E-15, 2.428612866367529932E-14, 167.9999999999999716 ) ) ;
#132442=CARTESIAN_POINT ( 'NONE',  ( -27.95311704539973974, -7.352561457324001459, 160.8984504615040976 ) ) ;
#132518=ORIENTED_EDGE ( 'NONE', *, *, #48174, .F. ) ;
#132546=CARTESIAN_POINT ( 'NONE',  ( 8.898068258721464119, 27.38543819252877398, 141.3843446568999980 ) ) ;
#132554=CARTESIAN_POINT ( 'NONE',  ( -23.64874990377911956, -15.04272038711346582, 165.8682408883346397 ) ) ;
#132567=CARTESIAN_POINT ( 'NONE',  ( 27.73933785331498925, -9.013057229001034898, 141.7750000027311899 ) ) ;
#132615=VECTOR ( 'NONE', #26276, 1000.000000000000000 ) ;
#132624=CARTESIAN_POINT ( 'NONE',  ( 22.44159573604009239, 16.30477369853692693, 142.5750000027311728 ) ) ;
#132625=CARTESIAN_POINT ( 'NONE',  ( 22.44159573604009239, 16.30477369853692693, 148.0750000027312012 ) ) ;
#132638=CARTESIAN_POINT ( 'NONE',  ( -5.359611314223446995E-15, 29.16686587814335851, 142.8750000027311842 ) ) ;
#132707=CARTESIAN_POINT ( 'NONE',  ( -26.45594755429569034, 8.318738267476192050, 167.5492909577866385 ) ) ;
#132747=CARTESIAN_POINT ( 'NONE',  ( 24.95262708931866058, 12.69764001896744432, 166.0532406165024497 ) ) ;
#132758=CARTESIAN_POINT ( 'NONE',  ( 8.906447517083050158, 27.41122689804195645, 149.4000000000000057 ) ) ;
#132792=CARTESIAN_POINT ( 'NONE',  ( -28.79475375365501932, 9.355982642740395150, 146.1656553485623249 ) ) ;
#132901=CARTESIAN_POINT ( 'NONE',  ( -21.38418241377623374, -5.438282248597753110, 174.2683007571264113 ) ) ;
#132915=CARTESIAN_POINT ( 'NONE',  ( -8.571926809382601320, -26.38167802310801591, 145.2750000027311899 ) ) ;
#132927=CARTESIAN_POINT ( 'NONE',  ( -24.95432927374998755, -4.974562764236790002, 190.0000000000000000 ) ) ;
#133038=ORIENTED_EDGE ( 'NONE', *, *, #43155, .F. ) ;
#133075=ORIENTED_EDGE ( 'NONE', *, *, #165138, .T. ) ;
#133103=CARTESIAN_POINT ( 'NONE',  ( -22.44159573604009950, -16.30477369853688430, 147.5750000027312012 ) ) ;
#133144=CARTESIAN_POINT ( 'NONE',  ( 24.51266705573319626, -8.027923408435217567, 167.0300397585817791 ) ) ;
#133164=B_SPLINE_CURVE_WITH_KNOTS ( 'NONE', 3,
 ( #52371, #128210, #67539, #17073, #36198, #174735, #140403, #4861, #81687, #126233, #189907, #48415, #51382, #80714, #171751, #125246, #129197, #49397, #173749, #78727, #110071, #64568 ),
 .UNSPECIFIED., .F., .F.,
 ( 4, 2, 2, 2, 2, 2, 2, 2, 2, 2, 4 ),
 ( 0.000000000000000000, 0.001027542925581743189, 0.002055085851163486379, 0.002568857313954357648, 0.003082628776745229785, 0.004110171702327031738, 0.004623943165117908212, 0.005137714627908783818, 0.006165257553490564521, 0.007192800479072345224, 0.008220343404654125927 ),
 .UNSPECIFIED. ) ;
#133168=EDGE_CURVE ( 'NONE', #62156, #193436, #25231, .T. ) ;
#133370=CARTESIAN_POINT ( 'NONE',  ( -28.79475375365571210, -9.355982642739411048, 146.0843446569000434 ) ) ;
#133437=CARTESIAN_POINT ( 'NONE',  ( -27.67912082739735524, -7.698001346388012145, 161.8872396492397741 ) ) ;
#133451=CARTESIAN_POINT ( 'NONE',  ( 21.94905633995363559, 7.481063542984161430, 170.0146117665088923 ) ) ;
#133542=CARTESIAN_POINT ( 'NONE',  ( -27.94119071623633843, 7.398115196984048403, 160.8979257793639590 ) ) ;
#133582=ORIENTED_EDGE ( 'NONE', *, *, #126480, .T. ) ;
#133620=CARTESIAN_POINT ( 'NONE',  ( -8.906447517083060816, 27.41122689804195645, 139.8500000054623911 ) ) ;
#133635=CARTESIAN_POINT ( 'NONE',  ( 8.571926809382603096, -26.38167802310801235, 141.9750000027312069 ) ) ;
#133705=CARTESIAN_POINT ( 'NONE',  ( -20.56371838171435584, 11.43208494587337043, 170.0924998638764976 ) ) ;
#133761=CARTESIAN_POINT ( 'NONE',  ( -8.906447517083060816, 27.41122689804195645, 147.5999999999999943 ) ) ;
#133870=EDGE_LOOP ( 'NONE', ( #92317, #28128 ) ) ;
#133925=CARTESIAN_POINT ( 'NONE',  ( -8.571926809382608425, 26.38167802310805854, 148.4750000027311785 ) ) ;
#133971=ADVANCED_FACE ( 'NONE', ( #184857 ), #189586, .F. ) ;
#134131=ORIENTED_EDGE ( 'NONE', *, *, #122987, .F. ) ;
#134159=CARTESIAN_POINT ( 'NONE',  ( 21.70479006154308621, -8.695791278452025708, 169.0563666577075423 ) ) ;
#134205=EDGE_CURVE ( 'NONE', #75891, #66692, #96803, .T. ) ;
#134266=CARTESIAN_POINT ( 'NONE',  ( 21.27717364736664152, 9.815017990598704500, 168.4818444780604523 ) ) ;
#134342=B_SPLINE_CURVE_WITH_KNOTS ( 'NONE', 3,
 ( #53216, #188768, #7705, #20888, #113878, #177590, #143225, #142238, #190747, #189761, #144228, #68383, #176588, #3723, #159393, #99718, #52221, #98711, #66397, #130035, #38062, #4707, #192746, #115900, #18918, #22894, #39057, #128059 ),
 .UNSPECIFIED., .F., .F.,
 ( 4, 2, 2, 2, 2, 2, 2, 2, 2, 2, 2, 2, 2, 4 ),
 ( 0.000000000000000000, 0.002181393419099474963, 0.004362786838198949926, 0.005453483547748686974, 0.006544180257298424890, 0.006816854434685860019, 0.007089528612073295148, 0.007225865700767011846, 0.007294034245113868893, 0.007362202789460725941, 0.007498539878154482537, 0.007634876966848239133, 0.008180225321623478887, 0.008725573676398716907 ),
 .UNSPECIFIED. ) ;
#134541=CONICAL_SURFACE ( 'NONE', #173181, 28.85599147140294107, 0.1745329251994333364 ) ;
#134581=AXIS2_PLACEMENT_3D ( 'NONE', #125841, #170361, #30865 ) ;
#134637=CARTESIAN_POINT ( 'NONE',  ( 1.993301997531345292E-15, -30.30510711980685912, 140.7500000054623683 ) ) ;
#134720=CARTESIAN_POINT ( 'NONE',  ( 10.65970682939788716, -25.60940286011448919, 139.9999999999999716 ) ) ;
#134775=EDGE_CURVE ( 'NONE', #105306, #104760, #30844, .T. ) ;
#134776=CARTESIAN_POINT ( 'NONE',  ( 17.14385361876520264, 23.59649016807275856, 140.6750000027311387 ) ) ;
#134844=AXIS2_PLACEMENT_3D ( 'NONE', #62652, #125338, #76834 ) ;
#134872=CIRCLE ( 'NONE', #89532, 28.79475375365586487 ) ;
#134882=ORIENTED_EDGE ( 'NONE', *, *, #120075, .T. ) ;
#134918=DIRECTION ( 'NONE',  ( 0.000000000000000000, 0.000000000000000000, 1.000000000000000000 ) ) ;
#134966=DIRECTION ( 'NONE',  ( 1.000000000000000000, 0.000000000000000000, 0.000000000000000000 ) ) ;
#135008=( BOUNDED_SURFACE ( )  B_SPLINE_SURFACE ( 1, 2, ( 
 ( #150637, #89941, #138423, #170758, #62566, #14086, #139409, #154589, #182957, #137429, #29278, #151622, #200103, #15087, #135470, #891, #167780, #109079, #122252, #124243, #181963, #59589, #32247, #76748, #197138, #13115, #61571, #123240, #185938, #44440, #47423, #184931, #43445, #46416, #121263, #153589, #106094, #12133, #16085, #73797, #90910, #45427, #108074, #199109, #105114, #58605, #92903, #120271, #152595, #183942, #136441, #169758, #166800, #75752, #28301, #60576, #107080, #74779, #168752, #198122, #30255, #91898, #31253, #77743, #18082, #156587, #96875, #49402, #2894, #93905, #48420, #187933, #112066, #80719, #188928, #155583, #111065, #17078, #186949, #110076, #50406, #79737, #141406, #64573, #171756, #140408, #157579, #173754, #126238, #35222, #172753, #65555, #34234, #78732, #1897, #63577, #95896, #33245, #125251, #19072, #127214 ),
 ( #142397, #94903, #3876, #50795, #14747, #45090, #15741, #29917, #1547, #199765, #63223, #123887, #74438, #189318, #76408, #91557, #97260, #30914, #61232, #158948, #137088, #46073, #124903, #108735, #140057, #136105, #169408, #197781, #28941, #13748, #78381, #106747, #153244, #168422, #75416, #59247, #77400, #112454, #138084, #16733, #107727, #170412, #121913, #120916, #155243, #174143, #122903, #44100, #182615, #90582, #92562, #167444, #152263, #35615, #184592, #154250, #139070, #548, #105758, #62219, #185585, #47075, #31904, #198776, #93557, #60242, #183606, #20437, #132624, #82088, #99270, #54779, #102288, #23451, #85098, #5263, #176138, #51777, #143781, #159955, #8277, #40618, #194312, #84099, #9289, #24463, #52768, #7259, #160957, #21443, #69955, #146784, #66945, #70954, #37607, #179150, #192303, #55778, #113437, #129596, #128607 ) ),
 .UNSPECIFIED., .F., .F., .T. ) 
 B_SPLINE_SURFACE_WITH_KNOTS ( ( 2, 2 ),
 ( 3, 2, 2, 2, 2, 2, 2, 2, 2, 2, 2, 2, 2, 2, 2, 2, 2, 2, 2, 2, 2, 2, 2, 2, 2, 2, 2, 2, 2, 2, 2, 2, 2, 2, 2, 2, 2, 2, 2, 2, 2, 2, 2, 2, 2, 2, 2, 2, 2, 2, 3 ),
 ( 0.000000000000000000, 1.000000000000000000 ),
 ( 0.000000000000000000, 0.02000000000000000042, 0.04000000000000000083, 0.05999999999999999778, 0.08000000000000000167, 0.1000000000000000056, 0.1199999999999999956, 0.1400000000000000133, 0.1600000000000000033, 0.1799999999999999933, 0.2000000000000000111, 0.2200000000000000011, 0.2399999999999999911, 0.2600000000000000089, 0.2800000000000000266, 0.2999999999999999889, 0.3200000000000000067, 0.3400000000000000244, 0.3599999999999999867, 0.3800000000000000044, 0.4000000000000000222, 0.4199999999999999845, 0.4400000000000000022, 0.4600000000000000200, 0.4799999999999999822, 0.5000000000000000000, 0.5200000000000000178, 0.5400000000000000355, 0.5600000000000000533, 0.5799999999999999600, 0.5999999999999999778, 0.6199999999999999956, 0.6400000000000000133, 0.6600000000000000311, 0.6800000000000000488, 0.6999999999999999556, 0.7199999999999999734, 0.7399999999999999911, 0.7600000000000000089, 0.7800000000000000266, 0.8000000000000000444, 0.8199999999999999512, 0.8399999999999999689, 0.8599999999999999867, 0.8800000000000000044, 0.9000000000000000222, 0.9200000000000000400, 0.9399999999999999467, 0.9599999999999999645, 0.9799999999999999822, 1.000000000000000000 ),
 .UNSPECIFIED. ) 
 GEOMETRIC_REPRESENTATION_ITEM ( )  RATIONAL_B_SPLINE_SURFACE ( (
 ( 1.000000000000000000, 0.9510565162951535312, 1.000000000000000000, 0.9510565162951535312, 1.000000000000000000, 0.9510565162951535312, 1.000000000000000000, 0.9510565162951535312, 1.000000000000000000, 0.9510565162951535312, 1.000000000000000000, 0.9510565162951535312, 1.000000000000000000, 0.9510565162951535312, 1.000000000000000000, 0.9510565162951535312, 1.000000000000000000, 0.9510565162951535312, 1.000000000000000000, 0.9510565162951535312, 1.000000000000000000, 0.9510565162951535312, 1.000000000000000000, 0.9510565162951535312, 1.000000000000000000, 0.9510565162951535312, 1.000000000000000000, 0.9510565162951535312, 1.000000000000000000, 0.9510565162951535312, 1.000000000000000000, 0.9510565162951535312, 1.000000000000000000, 0.9510565162951535312, 1.000000000000000000, 0.9510565162951535312, 1.000000000000000000, 0.9510565162951535312, 1.000000000000000000, 0.9510565162951535312, 1.000000000000000000, 0.9510565162951535312, 1.000000000000000000, 0.9510565162951535312, 1.000000000000000000, 0.9510565162951535312, 1.000000000000000000, 0.9510565162951535312, 1.000000000000000000, 0.9510565162951535312, 1.000000000000000000, 0.9510565162951535312, 1.000000000000000000, 0.9510565162951535312, 1.000000000000000000, 0.9510565162951535312, 1.000000000000000000, 0.9510565162951535312, 1.000000000000000000, 0.9510565162951535312, 1.000000000000000000, 0.9510565162951535312, 1.000000000000000000, 0.9510565162951535312, 1.000000000000000000, 0.9510565162951535312, 1.000000000000000000, 0.9510565162951535312, 1.000000000000000000, 0.9510565162951535312, 1.000000000000000000, 0.9510565162951535312, 1.000000000000000000, 0.9510565162951535312, 1.000000000000000000, 0.9510565162951535312, 1.000000000000000000, 0.9510565162951535312, 1.000000000000000000, 0.9510565162951535312, 1.000000000000000000, 0.9510565162951535312, 1.000000000000000000, 0.9510565162951535312, 1.000000000000000000, 0.9510565162951535312, 1.000000000000000000, 0.9510565162951535312, 1.000000000000000000, 0.9510565162951535312, 1.000000000000000000, 0.9510565162951535312, 1.000000000000000000, 0.9510565162951535312, 1.000000000000000000, 0.9510565162951535312, 1.000000000000000000, 0.9510565162951535312, 1.000000000000000000, 0.9510565162951535312, 1.000000000000000000),
 ( 1.000000000000000000, 0.9510565162951535312, 1.000000000000000000, 0.9510565162951535312, 1.000000000000000000, 0.9510565162951535312, 1.000000000000000000, 0.9510565162951535312, 1.000000000000000000, 0.9510565162951535312, 1.000000000000000000, 0.9510565162951535312, 1.000000000000000000, 0.9510565162951535312, 1.000000000000000000, 0.9510565162951535312, 1.000000000000000000, 0.9510565162951535312, 1.000000000000000000, 0.9510565162951535312, 1.000000000000000000, 0.9510565162951535312, 1.000000000000000000, 0.9510565162951535312, 1.000000000000000000, 0.9510565162951535312, 1.000000000000000000, 0.9510565162951535312, 1.000000000000000000, 0.9510565162951535312, 1.000000000000000000, 0.9510565162951535312, 1.000000000000000000, 0.9510565162951535312, 1.000000000000000000, 0.9510565162951535312, 1.000000000000000000, 0.9510565162951535312, 1.000000000000000000, 0.9510565162951535312, 1.000000000000000000, 0.9510565162951535312, 1.000000000000000000, 0.9510565162951535312, 1.000000000000000000, 0.9510565162951535312, 1.000000000000000000, 0.9510565162951535312, 1.000000000000000000, 0.9510565162951535312, 1.000000000000000000, 0.9510565162951535312, 1.000000000000000000, 0.9510565162951535312, 1.000000000000000000, 0.9510565162951535312, 1.000000000000000000, 0.9510565162951535312, 1.000000000000000000, 0.9510565162951535312, 1.000000000000000000, 0.9510565162951535312, 1.000000000000000000, 0.9510565162951535312, 1.000000000000000000, 0.9510565162951535312, 1.000000000000000000, 0.9510565162951535312, 1.000000000000000000, 0.9510565162951535312, 1.000000000000000000, 0.9510565162951535312, 1.000000000000000000, 0.9510565162951535312, 1.000000000000000000, 0.9510565162951535312, 1.000000000000000000, 0.9510565162951535312, 1.000000000000000000, 0.9510565162951535312, 1.000000000000000000, 0.9510565162951535312, 1.000000000000000000, 0.9510565162951535312, 1.000000000000000000, 0.9510565162951535312, 1.000000000000000000, 0.9510565162951535312, 1.000000000000000000, 0.9510565162951535312, 1.000000000000000000, 0.9510565162951535312, 1.000000000000000000, 0.9510565162951535312, 1.000000000000000000, 0.9510565162951535312, 1.000000000000000000, 0.9510565162951535312, 1.000000000000000000, 0.9510565162951535312, 1.000000000000000000) ) ) 
 REPRESENTATION_ITEM ( '' )  SURFACE ( )  );
#135124=CARTESIAN_POINT ( 'NONE',  ( -27.73933785331498925, 9.013057229001089965, 149.2750000027311330 ) ) ;
#135144=VERTEX_POINT ( 'NONE', #165903 ) ;
#135165=CARTESIAN_POINT ( 'NONE',  ( -24.54404792736193386, -12.06373989673657654, 169.8487138613016896 ) ) ;
#135238=ORIENTED_EDGE ( 'NONE', *, *, #57626, .T. ) ;
#135262=VERTEX_POINT ( 'NONE', #154688 ) ;
#135365=CARTESIAN_POINT ( 'NONE',  ( -21.81018892176227553, -9.477090470496813523, 170.9397748289982246 ) ) ;
#135405=FACE_OUTER_BOUND ( 'NONE', #159261, .T. ) ;
#135470=CARTESIAN_POINT ( 'NONE',  ( 8.571926809382603096, -26.38167802310801235, 147.4750000027311785 ) ) ;
#135553=CARTESIAN_POINT ( 'NONE',  ( 28.79475375365586132, 2.781246896534039337E-14, 140.9843446568999923 ) ) ;
#135555=CARTESIAN_POINT ( 'NONE',  ( -27.89903062892789620, 7.496893268503697527, 160.9845644947731387 ) ) ;
#135628=CARTESIAN_POINT ( 'NONE',  ( 22.44159573604009594, -16.30477369853687364, 141.6750000027311671 ) ) ;
#135695=CARTESIAN_POINT ( 'NONE',  ( 27.29906736325804673, 2.428612866367529932E-14, 169.9999999999999716 ) ) ;
#135710=CARTESIAN_POINT ( 'NONE',  ( -10.24465944170948895, -26.23679381505269959, 139.9999999999999716 ) ) ;
#135765=CARTESIAN_POINT ( 'NONE',  ( 22.44159573604009594, -16.30477369853687364, 140.1750000027311955 ) ) ;
#135780=CARTESIAN_POINT ( 'NONE',  ( 20.14845677604719754, -11.85354687992394496, 170.0217845860066745 ) ) ;
#135865=EDGE_LOOP ( 'NONE', ( #138257, #133582, #120183, #102533 ) ) ;
#135915=CARTESIAN_POINT ( 'NONE',  ( 27.73933785331498569, 9.013057229001093518, 145.9750000027311785 ) ) ;
#135939=VERTEX_POINT ( 'NONE', #143657 ) ;
#136101=CARTESIAN_POINT ( 'NONE',  ( -5.359611314223446995E-15, 29.16686587814335496, 144.8750000027311557 ) ) ;
#136105=CARTESIAN_POINT ( 'NONE',  ( -5.359611314223446995E-15, 29.16686587814335496, 146.8750000027311273 ) ) ;
#136110=CARTESIAN_POINT ( 'NONE',  ( 19.49401214000076621, 12.39993551617566681, 167.9999999999999716 ) ) ;
#136142=CARTESIAN_POINT ( 'NONE',  ( -20.56371838171433097, -11.43208494587363688, 170.0924998638764691 ) ) ;
#136214=VERTEX_POINT ( 'NONE', #101144 ) ;
#136259=CARTESIAN_POINT ( 'NONE',  ( 25.62086810090348976, 2.428612866367529932E-14, 167.9999999999999716 ) ) ;
#136341=CARTESIAN_POINT ( 'NONE',  ( -21.83923006935332367, -7.858462611068593340, 172.8812894384829519 ) ) ;
#136441=CARTESIAN_POINT ( 'NONE',  ( 27.73933785331498569, 2.768321779492822058E-14, 143.8750000027311842 ) ) ;
#136492=ORIENTED_EDGE ( 'NONE', *, *, #122945, .T. ) ;
#136526=CARTESIAN_POINT ( 'NONE',  ( -27.94727395831376882, 6.976223361892389896, 161.4607800657733492 ) ) ;
#136541=PLANE ( 'NONE',  #194989 ) ;
#136563=CARTESIAN_POINT ( 'NONE',  ( 27.05641397906351386, 3.631740835637567333, 169.9999999999999716 ) ) ;
#136598=FACE_OUTER_BOUND ( 'NONE', #37861, .T. ) ;
#136599=CARTESIAN_POINT ( 'NONE',  ( 8.571926809382597767, 26.38167802310806209, 144.2750000027311899 ) ) ;
#136656=EDGE_CURVE ( 'NONE', #146461, #119499, #91852, .T. ) ;
#136679=CARTESIAN_POINT ( 'NONE',  ( -26.79623349963135581, 5.044589688426436069, 170.2051123914324080 ) ) ;
#136735=CARTESIAN_POINT ( 'NONE',  ( 8.906447517083057264, -27.41122689804191026, 140.5999999999999943 ) ) ;
#136749=CARTESIAN_POINT ( 'NONE',  ( 24.95262708931878493, -12.69764001896723116, 166.0532406165022508 ) ) ;
#136752=CARTESIAN_POINT ( 'NONE',  ( -28.79475375365586842, 2.428612866367529932E-14, 144.2656553485623760 ) ) ;
#136776=EDGE_CURVE ( 'NONE', #31087, #46062, #2631, .T. ) ;
#136809=ADVANCED_FACE ( 'NONE', ( #124280, #151661 ), #13155, .T. ) ;
#136828=EDGE_CURVE ( 'NONE', #107664, #60981, #120806, .T. ) ;
#136838=CARTESIAN_POINT ( 'NONE',  ( -24.66578506923897152, -3.377805382906099219, 172.1149105766467926 ) ) ;
#136930=CARTESIAN_POINT ( 'NONE',  ( -3.573655867282028392E-15, 2.428612866367529932E-14, 155.0000000000000000 ) ) ;
#136965=ORIENTED_EDGE ( 'NONE', *, *, #32058, .T. ) ;
#137026=LINE ( 'NONE', #198716, #175387 ) ;
#137084=CARTESIAN_POINT ( 'NONE',  ( -27.73933785331498925, 9.013057229001089965, 141.2750000027311614 ) ) ;
#137088=CARTESIAN_POINT ( 'NONE',  ( -27.73933785331498925, 2.428612866367529932E-14, 147.3750000027311842 ) ) ;
#137091=( BOUNDED_CURVE ( )  B_SPLINE_CURVE ( 2, ( #35838, #70181, #143007, #128830, #55006 ),
 .UNSPECIFIED., .F., .T. ) 
 B_SPLINE_CURVE_WITH_KNOTS ( ( 3, 2, 3 ),
 ( 0.8000000000000035971, 0.8200000000000008393, 0.8266400941232673327 ),
 .UNSPECIFIED. ) 
 CURVE ( )  GEOMETRIC_REPRESENTATION_ITEM ( )  RATIONAL_B_SPLINE_CURVE ( ( 0.9999999999999913403, 0.9510565162951621909, 1.000000000000000000, 0.9837505330739607645, 0.9782908651321036153 ) ) 
 REPRESENTATION_ITEM ( '' )  );
#137125=CARTESIAN_POINT ( 'NONE',  ( -21.97054992548789087, -8.562709642470920812, 171.7904333278019351 ) ) ;
#137185=EDGE_CURVE ( 'NONE', #90049, #109599, #185741, .T. ) ;
#137326=CARTESIAN_POINT ( 'NONE',  ( -20.02446474427092937, -11.96320450740733676, 170.0134183209140133 ) ) ;
#137349=CARTESIAN_POINT ( 'NONE',  ( 23.29544513554940366, -16.92513159979222337, 146.7843446569000037 ) ) ;
#137429=CARTESIAN_POINT ( 'NONE',  ( 27.73933785331498214, 9.013057229001095294, 147.9750000027311501 ) ) ;
#137593=CARTESIAN_POINT ( 'NONE',  ( -27.73933785331498925, 9.013057229001089965, 144.7750000027311614 ) ) ;
#137606=CARTESIAN_POINT ( 'NONE',  ( 17.85839625232364014, -22.61300660583702538, 140.0884876851766876 ) ) ;
#137716=CARTESIAN_POINT ( 'NONE',  ( 26.68407921138447847, 3.932373394472265193, 171.8653659962753295 ) ) ;
#137731=CARTESIAN_POINT ( 'NONE',  ( -17.81289503416611808, 24.51734667627700404, 141.6999999999999602 ) ) ;
#137831=CARTESIAN_POINT ( 'NONE',  ( -21.93180397000192272, -7.641141194970263228, 169.8616410530808878 ) ) ;
#137956=EDGE_CURVE ( 'NONE', #101739, #172658, #106109, .T. ) ;
#137997=CARTESIAN_POINT ( 'NONE',  ( 24.07993927064490336, -13.88935938516710777, 140.0000000000000853 ) ) ;
#138080=CARTESIAN_POINT ( 'NONE',  ( 22.44159573604009594, -16.30477369853687364, 146.1750000027311671 ) ) ;
#138084=CARTESIAN_POINT ( 'NONE',  ( -22.44159573604009950, -16.30477369853688430, 145.5750000027311728 ) ) ;
#138121=CARTESIAN_POINT ( 'NONE',  ( -23.35043118190795042, -14.19381810412062883, 169.8796877288296798 ) ) ;
#138257=ORIENTED_EDGE ( 'NONE', *, *, #106636, .F. ) ;
#138322=CARTESIAN_POINT ( 'NONE',  ( -20.51334883519573182, 11.49142661404780696, 170.0774692710818101 ) ) ;
#138361=CARTESIAN_POINT ( 'NONE',  ( -24.10884208241213500, 5.471882726981272427, 173.8287385965644489 ) ) ;
#138423=CARTESIAN_POINT ( 'NONE',  ( -22.44159573604010305, 16.30477369853692338, 148.6750000027311671 ) ) ;
#138458=CARTESIAN_POINT ( 'NONE',  ( -27.18966431762779834, -4.276553394869433866, 168.7322077152509507 ) ) ;
#138580=CARTESIAN_POINT ( 'NONE',  ( 22.44159573604009594, -16.30477369853687364, 145.6750000027311671 ) ) ;
#138627=CARTESIAN_POINT ( 'NONE',  ( -24.95432927374998044, 3.806786798636383917, 190.0000000000000000 ) ) ;
#138666=VECTOR ( 'NONE', #97887, 1000.000000000000000 ) ;
#138705=ORIENTED_EDGE ( 'NONE', *, *, #114259, .F. ) ;
#138708=ORIENTED_EDGE ( 'NONE', *, *, #125504, .F. ) ;
#138719=CARTESIAN_POINT ( 'NONE',  ( -17.81289503416611097, -24.51734667627696496, 144.2999999999999829 ) ) ;
#138737=CARTESIAN_POINT ( 'NONE',  ( 19.49401214000073779, -12.39993551617566503, 169.9999999999999716 ) ) ;
#138895=CARTESIAN_POINT ( 'NONE',  ( 23.29544513554940366, -16.92513159979222337, 148.7843446569000037 ) ) ;
#138982=CARTESIAN_POINT ( 'NONE',  ( 26.33251596241889914, 8.908286433081562095, 140.0000000000000000 ) ) ;
#139035=ORIENTED_EDGE ( 'NONE', *, *, #77093, .T. ) ;
#139066=CARTESIAN_POINT ( 'NONE',  ( -22.44159573604010305, 16.30477369853692338, 143.1750000027311671 ) ) ;
#139070=CARTESIAN_POINT ( 'NONE',  ( -8.571926809382601320, -26.38167802310801591, 143.7750000027311899 ) ) ;
#139107=CARTESIAN_POINT ( 'NONE',  ( -26.57611637973506546, -7.696099174151179056, 167.9177021574075468 ) ) ;
#139124=CARTESIAN_POINT ( 'NONE',  ( -8.898068258721469448, -27.38543819252872069, 140.6656553485623817 ) ) ;
#139247=VERTEX_POINT ( 'NONE', #125045 ) ;
#139289=CARTESIAN_POINT ( 'NONE',  ( -23.84689744903970876, -10.26551614244695720, 166.0764362378396868 ) ) ;
#139316=DIRECTION ( 'NONE',  ( -1.000000000000000000, 0.000000000000000000, 0.000000000000000000 ) ) ;
#139348=CARTESIAN_POINT ( 'NONE',  ( -23.19706360625338704, 11.80427776162510689, 165.7059442611694067 ) ) ;
#139386=CARTESIAN_POINT ( 'NONE',  ( -3.573655867282028392E-15, 2.428612866367529932E-14, 165.5209445330007441 ) ) ;
#139409=CARTESIAN_POINT ( 'NONE',  ( 8.571926809382597767, 26.38167802310806209, 148.2750000027311899 ) ) ;
#139484=CARTESIAN_POINT ( 'NONE',  ( 8.898068258721464119, 27.38543819252877398, 143.3843446568999980 ) ) ;
#139569=CARTESIAN_POINT ( 'NONE',  ( -8.571926809382601320, -26.38167802310801591, 141.2750000027311899 ) ) ;
#139576=CARTESIAN_POINT ( 'NONE',  ( 22.78714015946003002, -11.73760554535578748, 167.9671921004704700 ) ) ;
#139602=CARTESIAN_POINT ( 'NONE',  ( -3.573655867282028392E-15, 2.428612866367529932E-14, 155.0000000000000000 ) ) ;
#139693=VERTEX_POINT ( 'NONE', #121237 ) ;
#139704=CARTESIAN_POINT ( 'NONE',  ( -28.82186960331499392, -9.364793116373526516, 144.0999999999999659 ) ) ;
#139716=CARTESIAN_POINT ( 'NONE',  ( 26.26139018963107219, -3.005588016160671838, 174.9127113745526287 ) ) ;
#139733=DIRECTION ( 'NONE',  ( -1.000000000000000000, 0.000000000000000000, -0.000000000000000000 ) ) ;
#140009=( BOUNDED_SURFACE ( )  B_SPLINE_SURFACE ( 3, 2, ( 
 ( #85183, #38705, #8364 ),
 ( #115545, #164060, #54865 ),
 ( #52853, #193389, #72032 ),
 ( #24549, #180240, #133705 ),
 ( #86199, #177233, #178227 ),
 ( #131708, #165052, #53871 ),
 ( #6348, #87203, #102371 ),
 ( #39691, #114524, #41709 ),
 ( #100362, #163042, #9375 ),
 ( #71040, #162041, #144865 ),
 ( #132707, #10375, #83191 ),
 ( #55863, #103374, #117537 ),
 ( #179235, #40701, #25559 ),
 ( #148884, #195397, #176225 ),
 ( #161041, #56875, #69029 ),
 ( #129679, #37694, #99358 ),
 ( #145862, #7344, #130694 ),
 ( #136679, #166049, #75014 ),
 ( #46664, #15332, #197381 ),
 ( #57873, #60823, #183199 ),
 ( #108323, #27549, #59836 ),
 ( #90176, #11378, #13350 ),
 ( #92149, #26545, #91150 ),
 ( #119545, #30498, #73048 ) ),
 .UNSPECIFIED., .F., .F., .F. ) 
 B_SPLINE_SURFACE_WITH_KNOTS ( ( 4, 2, 2, 2, 2, 2, 2, 2, 2, 2, 2, 4 ),
 ( 3, 3 ),
 ( -8.673617379884035472E-19, 0.001899702839891689908, 0.002849554259837535405, 0.003799405679783380684, 0.005699108519675071677, 0.006648959939620916956, 0.007598811359566762236, 0.008548662779512607515, 0.009498514199458452795, 0.01139821703935014335, 0.01329791987924183391, 0.01519762271913352447 ),
 ( 0.000000000000000000, 1.000000000000000000 ),
 .UNSPECIFIED. ) 
 GEOMETRIC_REPRESENTATION_ITEM ( )  RATIONAL_B_SPLINE_SURFACE ( (
 ( 1.000000000000000000, 0.7660444431189777914, 1.000000000000000000),
 ( 1.000000000000000000, 0.7753720600381861505, 1.000000000000000000),
 ( 1.000000000000000000, 0.7832595754286625356, 1.000000000000000000),
 ( 1.000000000000000000, 0.7928595458705119947, 1.000000000000000000),
 ( 1.000000000000000000, 0.7956872332516092827, 1.000000000000000000),
 ( 1.000000000000000000, 0.8005750596157589216, 1.000000000000000000),
 ( 1.000000000000000000, 0.8026302056541514407, 1.000000000000000000),
 ( 1.000000000000000000, 0.8075080643848788764, 1.000000000000000000),
 ( 1.000000000000000000, 0.8091143015810093875, 1.000000000000000000),
 ( 1.000000000000000000, 0.8093067629632906268, 1.000000000000000000),
 ( 1.000000000000000000, 0.8089952915731616345, 1.000000000000000000),
 ( 1.000000000000000000, 0.8076919994862351571, 1.000000000000000000),
 ( 1.000000000000000000, 0.8067078407648706762, 1.000000000000000000),
 ( 1.000000000000000000, 0.8041786842467621987, 1.000000000000000000),
 ( 1.000000000000000000, 0.8026334674877082520, 1.000000000000000000),
 ( 1.000000000000000000, 0.7990747329469325422, 1.000000000000000000),
 ( 1.000000000000000000, 0.7970509760941956179, 1.000000000000000000),
 ( 1.000000000000000000, 0.7904793850863031102, 1.000000000000000000),
 ( 1.000000000000000000, 0.7855040224313080133, 1.000000000000000000),
 ( 1.000000000000000000, 0.7751942650508213406, 1.000000000000000000),
 ( 1.000000000000000000, 0.7698260778211012401, 1.000000000000000000),
 ( 1.000000000000000000, 0.7598259884961471311, 1.000000000000000000),
 ( 1.000000000000000000, 0.7551428682219897270, 1.000000000000000000),
 ( 1.000000000000000000, 0.7510191126010854479, 1.000000000000000000) ) ) 
 REPRESENTATION_ITEM ( '' )  SURFACE ( )  );
#140022=ORIENTED_EDGE ( 'NONE', *, *, #61909, .T. ) ;
#140057=CARTESIAN_POINT ( 'NONE',  ( -8.571926809382608425, 26.38167802310805854, 146.9750000027311785 ) ) ;
#140183=ADVANCED_FACE ( 'NONE', ( #15061 ), #77717, .T. ) ;
#140200=CARTESIAN_POINT ( 'NONE',  ( 28.79475375365586132, 2.781246896534039337E-14, 143.2656553485623760 ) ) ;
#140232=VERTEX_POINT ( 'NONE', #95871 ) ;
#140302=CARTESIAN_POINT ( 'NONE',  ( -21.76480897080537602, 7.725232727579774306, 173.1951875983968137 ) ) ;
#140343=CARTESIAN_POINT ( 'NONE',  ( -21.51693143705273670, 9.260949364272581974, 168.7281092719940432 ) ) ;
#140369=ORIENTED_EDGE ( 'NONE', *, *, #12998, .T. ) ;
#140403=CARTESIAN_POINT ( 'NONE',  ( 21.93653645885849457, 8.192071713419744938, 172.2938920027118570 ) ) ;
#140408=CARTESIAN_POINT ( 'NONE',  ( -5.359611314223446995E-15, 29.16686587814335496, 140.3750000027311842 ) ) ;
#140689=B_SPLINE_CURVE_WITH_KNOTS ( 'NONE', 3,
 ( #58832, #163028, #23523, #55849, #85169, #24534 ),
 .UNSPECIFIED., .F., .F.,
 ( 4, 2, 4 ),
 ( 0.0003734705499802213453, 0.004296280022383715952, 0.008219089494787211805 ),
 .UNSPECIFIED. ) ;
#140708=CARTESIAN_POINT ( 'NONE',  ( 17.81289503416610742, 24.51734667627700404, 141.2999999999999829 ) ) ;
#140721=CARTESIAN_POINT ( 'NONE',  ( 26.77293948118372313, -6.014770499723137931, 169.2063755025577336 ) ) ;
#140802=CARTESIAN_POINT ( 'NONE',  ( -23.31738231874055600, 16.94106989632528837, 148.0500000054623797 ) ) ;
#140815=DIRECTION ( 'NONE',  ( 0.000000000000000000, 0.000000000000000000, -1.000000000000000000 ) ) ;
#140818=CARTESIAN_POINT ( 'NONE',  ( -17.14385361876520975, 23.59649016807275856, 147.0750000027312012 ) ) ;
#140968=DIRECTION ( 'NONE',  ( 1.000000000000000000, 0.000000000000000000, -0.000000000000000000 ) ) ;
#140971=CARTESIAN_POINT ( 'NONE',  ( 24.93761727085874469, -12.28292609113013256, 139.9999999999999716 ) ) ;
#141113=CARTESIAN_POINT ( 'NONE',  ( 23.29544513554940366, -16.92513159979222337, 141.0656553485623590 ) ) ;
#141341=CARTESIAN_POINT ( 'NONE',  ( -22.65770943308888619, 11.99324031494455589, 167.9410816520763206 ) ) ;
#141406=CARTESIAN_POINT ( 'NONE',  ( -22.44159573604010305, 16.30477369853692338, 140.6750000027311671 ) ) ;
#141421=CARTESIAN_POINT ( 'NONE',  ( 27.96813078753324078, -7.160245613315928459, 161.0900052257271966 ) ) ;
#141478=ORIENTED_EDGE ( 'NONE', *, *, #124946, .T. ) ;
#141530=CARTESIAN_POINT ( 'NONE',  ( 27.88129983271499768, 6.733757357597986548, 162.1517353552272880 ) ) ;
#141542=CARTESIAN_POINT ( 'NONE',  ( 25.63014048727049854, -6.600871414792749192, 163.2070037194164911 ) ) ;
#141591=EDGE_CURVE ( 'NONE', #88085, #163981, #17691, .T. ) ;
#141716=CARTESIAN_POINT ( 'NONE',  ( 25.75939503182788926, -8.559839547495068146, 171.7912139782359588 ) ) ;
#141720=DIRECTION ( 'NONE',  ( -0.1039620511844979306, -0.1039620511844979306, 0.9891328443778538704 ) ) ;
#141794=CARTESIAN_POINT ( 'NONE',  ( 23.31738231874054534, 16.94106989632529192, 147.4500000054623854 ) ) ;
#141856=CARTESIAN_POINT ( 'NONE',  ( -8.898068258721474777, 27.38543819252877398, 147.8656553485623704 ) ) ;
#142029=EDGE_CURVE ( 'NONE', #173841, #135262, #105841, .T. ) ;
#142063=CARTESIAN_POINT ( 'NONE',  ( -29.15849868437705439, -8.010956209263452976, 149.7909430734646890 ) ) ;
#142238=CARTESIAN_POINT ( 'NONE',  ( 27.60805440473492567, 7.718125693463445458, 162.2444234560357756 ) ) ;
#142273=ORIENTED_EDGE ( 'NONE', *, *, #176999, .T. ) ;
#142330=CARTESIAN_POINT ( 'NONE',  ( -21.84611564451296672, 8.148379233837022895, 169.4346228884802485 ) ) ;
#142397=CARTESIAN_POINT ( 'NONE',  ( -27.73933785331498925, 2.428612866367529932E-14, 149.3750000027311842 ) ) ;
#142434=CARTESIAN_POINT ( 'NONE',  ( 1.988064558232696151E-15, -30.27659582821216588, 146.7656553485623760 ) ) ;
#142623=CARTESIAN_POINT ( 'NONE',  ( 21.88033147701376890, 7.974798826777440119, 169.5716465351766260 ) ) ;
#142632=( BOUNDED_CURVE ( )  B_SPLINE_CURVE ( 2, ( #106573, #198604, #79212, #64051, #184422, #46900, #76230, #108560, #138895, #75246, #199592 ),
 .UNSPECIFIED., .F., .T. ) 
 B_SPLINE_CURVE_WITH_KNOTS ( ( 3, 2, 2, 2, 2, 3 ),
 ( 0.8000000000000007105, 0.8200000000000007283, 0.8400000000000006350, 0.8600000000000007638, 0.8800000000000007816, 0.9000000000000007994 ),
 .UNSPECIFIED. ) 
 CURVE ( )  GEOMETRIC_REPRESENTATION_ITEM ( )  RATIONAL_B_SPLINE_CURVE ( ( 0.9999999999999983347, 0.9510565162951551965, 1.000000000000000000, 0.9510565162951535312, 1.000000000000000000, 0.9510565162951535312, 1.000000000000000000, 0.9510565162951535312, 1.000000000000000000, 0.9510565162951516438, 1.000000000000001998 ) ) 
 REPRESENTATION_ITEM ( '' )  );
#142686=CARTESIAN_POINT ( 'NONE',  ( -24.93942350307309752, 7.769968609432599926, 171.2173313942149946 ) ) ;
#142707=CARTESIAN_POINT ( 'NONE',  ( 21.56952297831669441, -7.512152360717372801, 173.9007003117368697 ) ) ;
#142713=SURFACE_SIDE_STYLE ('',( #18403 ) ) ;
#142758=CARTESIAN_POINT ( 'NONE',  ( -24.81835880841865816, 6.052260367207988878, 168.4265213779230521 ) ) ;
#142786=CARTESIAN_POINT ( 'NONE',  ( -23.31738231874055245, -16.94106989632524574, 146.4500000054623854 ) ) ;
#143007=CARTESIAN_POINT ( 'NONE',  ( -23.29544513554941076, 16.92513159979227666, 140.0656553485623590 ) ) ;
#143098=ORIENTED_EDGE ( 'NONE', *, *, #121993, .F. ) ;
#143145=ORIENTED_EDGE ( 'NONE', *, *, #32058, .F. ) ;
#143225=CARTESIAN_POINT ( 'NONE',  ( 27.46944729267101337, 7.746537029272661634, 162.9576794167388130 ) ) ;
#143250=CARTESIAN_POINT ( 'NONE',  ( -23.27014359241646702, 11.64952062020055479, 165.7333947824558322 ) ) ;
#143260=CARTESIAN_POINT ( 'NONE',  ( 25.31005825231498108, 7.802036135343648482, 170.7258689498729609 ) ) ;
#143350=DIRECTION ( 'NONE',  ( 0.8437662581494472791, 0.5367108174878539861, 0.000000000000000000 ) ) ;
#143417=CARTESIAN_POINT ( 'NONE',  ( -24.93942350307309752, -7.769968609432603479, 171.2173313942149662 ) ) ;
#143509=CARTESIAN_POINT ( 'NONE',  ( -28.79475375365586487, 2.428612866367529932E-14, 149.9843446568999923 ) ) ;
#143534=EDGE_LOOP ( 'NONE', ( #183992, #57688, #43383, #120411 ) ) ;
#143545=CARTESIAN_POINT ( 'NONE',  ( -27.88129983271662837, 6.733757357602863536, 162.1517353552117982 ) ) ;
#143548=DIRECTION ( 'NONE',  ( 0.000000000000000000, 0.000000000000000000, 1.000000000000000000 ) ) ;
#143611=CARTESIAN_POINT ( 'NONE',  ( 23.03120525563286236, 11.22467059994808558, 168.0473679553712429 ) ) ;
#143619=DIRECTION ( 'NONE',  ( 0.000000000000000000, 0.000000000000000000, 1.000000000000000000 ) ) ;
#143657=CARTESIAN_POINT ( 'NONE',  ( -24.93942350307309752, 7.769968609432599926, 171.2173313942149946 ) ) ;
#143700=CARTESIAN_POINT ( 'NONE',  ( 25.76143648876522718, -7.343476467571410815, 174.8772314887141306 ) ) ;
#143722=CARTESIAN_POINT ( 'NONE',  ( -24.12203661075782790, -5.823883908176388680, 170.5995460337422855 ) ) ;
#143727=CARTESIAN_POINT ( 'NONE',  ( -17.14385361876520975, 23.59649016807275856, 144.5750000027311728 ) ) ;
#143761=ORIENTED_EDGE ( 'NONE', *, *, #94032, .F. ) ;
#143781=CARTESIAN_POINT ( 'NONE',  ( -22.44159573604009950, -16.30477369853688430, 141.5750000027311728 ) ) ;
#143782=CARTESIAN_POINT ( 'NONE',  ( -8.906447517083053711, -27.41122689804191026, 146.6500000054623740 ) ) ;
#143820=FACE_OUTER_BOUND ( 'NONE', #162693, .T. ) ;
#143910=B_SPLINE_CURVE_WITH_KNOTS ( 'NONE', 3,
 ( #192013, #53497, #115174, #21167, #38336, #99992, #23173, #141530 ),
 .UNSPECIFIED., .F., .F.,
 ( 4, 2, 2, 4 ),
 ( 2.244678719550583187E-07, 0.002115167047686612300, 0.004230109627501268954, 0.008459994787130583130 ),
 .UNSPECIFIED. ) ;
#144101=EDGE_LOOP ( 'NONE', ( #121173, #16698 ) ) ;
#144214=ORIENTED_EDGE ( 'NONE', *, *, #94032, .T. ) ;
#144228=CARTESIAN_POINT ( 'NONE',  ( 27.79720911488089641, 7.618197028328711262, 161.3616953378221410 ) ) ;
#144253=CARTESIAN_POINT ( 'NONE',  ( -24.66672740160584354, -7.254147403784508619, 167.4978451254145000 ) ) ;
#144397=ORIENTED_EDGE ( 'NONE', *, *, #19482, .T. ) ;
#144435=DIRECTION ( 'NONE',  ( -1.000000000000000000, 0.000000000000000000, 0.000000000000000000 ) ) ;
#144442=AXIS2_PLACEMENT_3D ( 'NONE', #130693, #103373, #195396 ) ;
#144449=VERTEX_POINT ( 'NONE', #33066 ) ;
#144492=FACE_BOUND ( 'NONE', #128554, .T. ) ;
#144548=CARTESIAN_POINT ( 'NONE',  ( 17.14385361876520264, -23.59649016807271238, 139.5750000027311444 ) ) ;
#144722=CARTESIAN_POINT ( 'NONE',  ( -8.571926809382608425, 26.38167802310805854, 144.4750000027312069 ) ) ;
#144781=CARTESIAN_POINT ( 'NONE',  ( 8.906447517083057264, -27.41122689804191026, 144.8500000054623911 ) ) ;
#144795=CARTESIAN_POINT ( 'NONE',  ( -8.571926809382608425, 26.38167802310805854, 140.9750000027312069 ) ) ;
#144865=CARTESIAN_POINT ( 'NONE',  ( -21.70479006154311108, 9.754118203517286645, 170.7545476126474284 ) ) ;
#144906=CARTESIAN_POINT ( 'NONE',  ( 25.55222625260933356, 11.31436996698904629, 166.3494238031456405 ) ) ;
#144934=VERTEX_POINT ( 'NONE', #2717 ) ;
#144964=VERTEX_POINT ( 'NONE', #13909 ) ;
#145128=AXIS2_PLACEMENT_3D ( 'NONE', #25517, #41669, #198320 ) ;
#145202=FACE_OUTER_BOUND ( 'NONE', #150544, .T. ) ;
#145251=CARTESIAN_POINT ( 'NONE',  ( -24.75981411741738469, -6.635778407390994893, 167.9383864321132762 ) ) ;
#145261=PLANE ( 'NONE',  #102781 ) ;
#145309=CARTESIAN_POINT ( 'NONE',  ( 24.20757866959953120, -5.698759791481386117, 172.9004493943156433 ) ) ;
#145356=CARTESIAN_POINT ( 'NONE',  ( 22.77340731150488651, 12.66915506687109350, 165.5704399981227368 ) ) ;
#145582=CARTESIAN_POINT ( 'NONE',  ( 21.87067081123542778, -5.494950430485622483, 173.7269556299024202 ) ) ;
#145614=CARTESIAN_POINT ( 'NONE',  ( 23.46037622755597951, 10.21219847193880703, 168.3031241911625386 ) ) ;
#145779=CARTESIAN_POINT ( 'NONE',  ( -8.906447517083053711, -27.41122689804191026, 138.6500000054623740 ) ) ;
#145792=CARTESIAN_POINT ( 'NONE',  ( 22.44159573604009239, 16.30477369853692693, 144.5750000027311728 ) ) ;
#145862=CARTESIAN_POINT ( 'NONE',  ( -26.78465914369783007, 5.761000505272440897, 169.4491075441771670 ) ) ;
#145904=CARTESIAN_POINT ( 'NONE',  ( 21.94905633995363559, 8.886455535323596777, 171.4390084046502523 ) ) ;
#145915=ORIENTED_EDGE ( 'NONE', *, *, #88289, .F. ) ;
#145996=EDGE_LOOP ( 'NONE', ( #35512, #51675, #39497, #185518, #29844, #31324 ) ) ;
#146003=CARTESIAN_POINT ( 'NONE',  ( -24.37407968765138833, 13.84118768211350492, 165.9040744261181430 ) ) ;
#146031=CARTESIAN_POINT ( 'NONE',  ( -21.38418241377624085, 7.427326039334300134, 174.4773576836617224 ) ) ;
#146141=VERTEX_POINT ( 'NONE', #110836 ) ;
#146187=LINE ( 'NONE', #115870, #6412 ) ;
#146217=CARTESIAN_POINT ( 'NONE',  ( 20.71617105148682469, 18.73729486426113766, 139.9999999999999716 ) ) ;
#146255=EDGE_CURVE ( 'NONE', #34840, #35595, #27646, .T. ) ;
#146262=CARTESIAN_POINT ( 'NONE',  ( 27.73933785331498925, -9.013057229001033122, 148.2750000027311330 ) ) ;
#146268=CARTESIAN_POINT ( 'NONE',  ( -21.98685479826776756, -13.98560643873834586, 165.5209445330007725 ) ) ;
#146285=ORIENTED_EDGE ( 'NONE', *, *, #136776, .F. ) ;
#146306=CARTESIAN_POINT ( 'NONE',  ( 24.86035471869044500, -4.680034064337648125, 169.8578160361101084 ) ) ;
#146408=CARTESIAN_POINT ( 'NONE',  ( 20.96339774546123635, 10.39907118706507028, 168.2889211417203228 ) ) ;
#146458=CARTESIAN_POINT ( 'NONE',  ( -3.573655867282028392E-15, 2.428612866367529932E-14, 165.5209445330007441 ) ) ;
#146461=VERTEX_POINT ( 'NONE', #53139 ) ;
#146502=( BOUNDED_CURVE ( )  B_SPLINE_CURVE ( 2, ( #154665, #167855, #29355, #16161, #139484, #44516, #185007, #125329, #59668, #61646, #168828 ),
 .UNSPECIFIED., .F., .F. ) 
 B_SPLINE_CURVE_WITH_KNOTS ( ( 3, 2, 2, 2, 2, 3 ),
 ( 0.2999999999999974909, 0.3199999999999979527, 0.3399999999999985811, 0.3599999999999991540, 0.3799999999999997824, 0.4000000000000003553 ),
 .UNSPECIFIED. ) 
 CURVE ( )  GEOMETRIC_REPRESENTATION_ITEM ( )  RATIONAL_B_SPLINE_CURVE ( ( 1.000000000000006217, 0.9510565162951473139, 1.000000000000000000, 0.9510565162951535312, 1.000000000000000000, 0.9510565162951535312, 1.000000000000000000, 0.9510565162951535312, 1.000000000000000000, 0.9510565162951527540, 1.000000000000000888 ) ) 
 REPRESENTATION_ITEM ( '' )  );
#146513=ORIENTED_EDGE ( 'NONE', *, *, #164239, .T. ) ;
#146596=AXIS2_PLACEMENT_3D ( 'NONE', #194732, #115880, #190727 ) ;
#146698=CARTESIAN_POINT ( 'NONE',  ( -25.38323934330066933, 4.814940836774129096, 166.7856488131976676 ) ) ;
#146723=CARTESIAN_POINT ( 'NONE',  ( 25.64061671795035124, 10.58440545630783269, 139.9999999999999716 ) ) ;
#146730=CIRCLE ( 'NONE', #14391, 23.10356920737165254 ) ;
#146784=CARTESIAN_POINT ( 'NONE',  ( 27.73933785331498925, -9.013057229001033122, 140.2750000027311330 ) ) ;
#146785=CARTESIAN_POINT ( 'NONE',  ( -27.73933785331498925, 2.428612866367529932E-14, 148.8750000027311842 ) ) ;
#146798=CARTESIAN_POINT ( 'NONE',  ( 17.14385361876520264, -23.59649016807270883, 146.0750000027311728 ) ) ;
#146917=EDGE_LOOP ( 'NONE', ( #29906, #162615, #77275, #92623, #84284 ) ) ;
#146919=CARTESIAN_POINT ( 'NONE',  ( 21.88033147701376890, 9.239123595177357373, 171.1226046679828983 ) ) ;
#146931=CARTESIAN_POINT ( 'NONE',  ( 17.81289503416611453, -24.51734667627695785, 148.6999999999999602 ) ) ;
#146959=CARTESIAN_POINT ( 'NONE',  ( -27.88129983271662837, 6.733757357602863536, 162.1517353552117982 ) ) ;
#146964=CARTESIAN_POINT ( 'NONE',  ( -28.79475375365586842, 2.428612866367529932E-14, 146.2656553485623760 ) ) ;
#147012=ORIENTED_EDGE ( 'NONE', *, *, #75822, .T. ) ;
#147104=FACE_OUTER_BOUND ( 'NONE', #144101, .T. ) ;
#147212=VERTEX_POINT ( 'NONE', #44920 ) ;
#147252=ORIENTED_EDGE ( 'NONE', *, *, #45518, .T. ) ;
#147286=CARTESIAN_POINT ( 'NONE',  ( -23.84827716990831803, -9.022217638662285211, 168.8513102586128412 ) ) ;
#147383=B_SPLINE_CURVE_WITH_KNOTS ( 'NONE', 3,
 ( #164651, #59439, #178826, #40296, #25153, #165647, #28149, #148482, #120123, #26146 ),
 .UNSPECIFIED., .F., .F.,
 ( 4, 2, 2, 2, 4 ),
 ( 0.000000000000000000, 0.0009193652485010883092, 0.001838730497002176618, 0.002758095745503264928, 0.003677460994004353237 ),
 .UNSPECIFIED. ) ;
#147510=DIRECTION ( 'NONE',  ( 0.000000000000000000, 0.000000000000000000, -1.000000000000000000 ) ) ;
#147580=DIRECTION ( 'NONE',  ( 1.000000000000000000, 0.000000000000000000, 0.000000000000000000 ) ) ;
#147619=CARTESIAN_POINT ( 'NONE',  ( -26.58496454516998853, -7.626754437231455519, 167.9682100371138915 ) ) ;
#147632=CARTESIAN_POINT ( 'NONE',  ( 24.14511064691323838, 7.743397529683260672, 169.7652520481095735 ) ) ;
#147647=CONICAL_SURFACE ( 'NONE', #102468, 30.82560697742735556, 0.1745329251994333364 ) ;
#147692=ORIENTED_EDGE ( 'NONE', *, *, #70540, .T. ) ;
#147746=CARTESIAN_POINT ( 'NONE',  ( -17.14385361876520264, -23.59649016807271238, 143.1750000027311671 ) ) ;
#147795=AXIS2_PLACEMENT_3D ( 'NONE', #11524, #195541, #26688 ) ;
#147805=CARTESIAN_POINT ( 'NONE',  ( -8.571926809382608425, 26.38167802310805854, 148.4750000027311785 ) ) ;
#147818=CARTESIAN_POINT ( 'NONE',  ( 22.44159573604009594, -16.30477369853687364, 144.1750000027311671 ) ) ;
#147843=ORIENTED_EDGE ( 'NONE', *, *, #61909, .F. ) ;
#147866=FACE_OUTER_BOUND ( 'NONE', #180160, .T. ) ;
#147882=CARTESIAN_POINT ( 'NONE',  ( -27.29906736325805383, 2.072701884453516521E-14, 169.9999999999999716 ) ) ;
#147940=CARTESIAN_POINT ( 'NONE',  ( -17.81289503416611808, 24.51734667627700404, 145.6999999999999886 ) ) ;
#148025=CARTESIAN_POINT ( 'NONE',  ( 27.60098488412532447, -5.861468761074972278, 164.8187539380760143 ) ) ;
#148094=CARTESIAN_POINT ( 'NONE',  ( 8.571926809382603096, -26.38167802310801235, 145.4750000027311785 ) ) ;
#148158=EDGE_CURVE ( 'NONE', #60981, #95658, #63049, .T. ) ;
#148204=CARTESIAN_POINT ( 'NONE',  ( 24.84743926645689172, -12.91388972341063202, 166.0204189386424787 ) ) ;
#148251=ADVANCED_FACE ( 'NONE', ( #158050 ), #127698, .T. ) ;
#148282=CARTESIAN_POINT ( 'NONE',  ( 17.14385361876520264, 23.59649016807275856, 148.6750000027311387 ) ) ;
#148323=CARTESIAN_POINT ( 'NONE',  ( 24.50238749460113397, -2.981321037229046400, 173.3223451563237916 ) ) ;
#148427=CARTESIAN_POINT ( 'NONE',  ( 21.44939319537015265, 9.428468639168977816, 168.6471776813584711 ) ) ;
#148482=CARTESIAN_POINT ( 'NONE',  ( 25.31021317688468031, -7.802057701675677137, 170.7256852586635318 ) ) ;
#148509=CARTESIAN_POINT ( 'NONE',  ( 24.95432927374997334, 3.806786798636384805, 190.0000000000000000 ) ) ;
#148543=VERTEX_POINT ( 'NONE', #83186 ) ;
#148564=DIRECTION ( 'NONE',  ( 0.000000000000000000, -1.000000000000000000, 0.000000000000000000 ) ) ;
#148610=CARTESIAN_POINT ( 'NONE',  ( 28.79475375365586132, 2.781246896534039337E-14, 142.9843446568999639 ) ) ;
#148616=CARTESIAN_POINT ( 'NONE',  ( -27.95742675678272704, -7.330130391662396327, 160.9071069586228191 ) ) ;
#148631=CARTESIAN_POINT ( 'NONE',  ( 24.73536985823908196, 3.645104810706905507, 171.5180696409492782 ) ) ;
#148675=CARTESIAN_POINT ( 'NONE',  ( -21.38418241377624085, 7.427326039334300134, 174.4773576836617224 ) ) ;
#148725=CARTESIAN_POINT ( 'NONE',  ( -27.96619922901617628, 7.272069078173023726, 160.9422763814154962 ) ) ;
#148762=VERTEX_POINT ( 'NONE', #8360 ) ;
#148780=ORIENTED_EDGE ( 'NONE', *, *, #2128, .T. ) ;
#148802=CARTESIAN_POINT ( 'NONE',  ( 27.73933785331498214, 9.013057229001095294, 147.9750000027311501 ) ) ;
#148814=CARTESIAN_POINT ( 'NONE',  ( 27.73933785331498569, 2.768321779492822058E-14, 142.3750000027311842 ) ) ;
#148884=CARTESIAN_POINT ( 'NONE',  ( -26.70292545465260758, 6.820347898102890660, 168.5277281069536741 ) ) ;
#148927=CARTESIAN_POINT ( 'NONE',  ( 26.45763050569054542, 3.219288925403916313, 173.6696415116524861 ) ) ;
#148930=EDGE_LOOP ( 'NONE', ( #71374, #20942, #134131 ) ) ;
#148939=CARTESIAN_POINT ( 'NONE',  ( -22.44159573604010305, 16.30477369853692338, 141.1750000027311671 ) ) ;
#149108=CARTESIAN_POINT ( 'NONE',  ( -24.13306144861384794, -5.795830589372931385, 190.0000000000000000 ) ) ;
#149322=CARTESIAN_POINT ( 'NONE',  ( 24.83221077041874736, -4.296110748028930892, 170.3917201292316292 ) ) ;
#149520=CARTESIAN_POINT ( 'NONE',  ( -21.59136165864583390, -7.527668378163608232, 173.8290135686407893 ) ) ;
#149624=CARTESIAN_POINT ( 'NONE',  ( 24.85901545656365386, 5.346793810781362843, 169.1018111888376723 ) ) ;
#149635=ORIENTED_EDGE ( 'NONE', *, *, #199141, .F. ) ;
#149691=CARTESIAN_POINT ( 'NONE',  ( 25.63014143074630269, 6.600872056147826683, 163.2069976173305292 ) ) ;
#149715=CARTESIAN_POINT ( 'NONE',  ( 23.29544513554940011, 16.92513159979228021, 141.1843446569000093 ) ) ;
#149741=ORIENTED_EDGE ( 'NONE', *, *, #175002, .F. ) ;
#149792=CARTESIAN_POINT ( 'NONE',  ( 17.81289503416611453, -24.51734667627695785, 142.9500000054623854 ) ) ;
#149824=AXIS2_PLACEMENT_3D ( 'NONE', #136930, #44930, #8858 ) ;
#149928=CARTESIAN_POINT ( 'NONE',  ( -23.31738231874055245, -16.94106989632524574, 148.1999999999999886 ) ) ;
#150332=CARTESIAN_POINT ( 'NONE',  ( -24.05407591190816063, -13.01182159662975302, 169.7785964492051960 ) ) ;
#150468=CARTESIAN_POINT ( 'NONE',  ( -21.48948823426666976, 5.485118590273159178, 173.8226827327241608 ) ) ;
#150496=CARTESIAN_POINT ( 'NONE',  ( 28.79475375365498380, -9.355982642740388044, 145.1656553485623817 ) ) ;
#150543=ADVANCED_FACE ( 'NONE', ( #77974 ), #66415, .F. ) ;
#150544=EDGE_LOOP ( 'NONE', ( #165945, #27356, #63978, #29419, #156296, #47566, #24620, #187074 ) ) ;
#150637=CARTESIAN_POINT ( 'NONE',  ( -27.73933785331498925, 2.428612866367529932E-14, 148.8750000027311842 ) ) ;
#150696=CARTESIAN_POINT ( 'NONE',  ( 8.898068258721465895, 27.38543819252877398, 141.6656553485623817 ) ) ;
#150723=CARTESIAN_POINT ( 'NONE',  ( -27.95720134624904318, 7.331398113985295062, 160.9065205403411767 ) ) ;
#150738=CARTESIAN_POINT ( 'NONE',  ( -3.573655867282028392E-15, 2.428612866367529932E-14, 169.9999999999999716 ) ) ;
#150798=DIRECTION ( 'NONE',  ( 0.000000000000000000, 0.000000000000000000, -1.000000000000000000 ) ) ;
#150799=CARTESIAN_POINT ( 'NONE',  ( 22.44159573604009594, -16.30477369853687364, 143.6750000027311671 ) ) ;
#150859=PLANE ( 'NONE',  #14510 ) ;
#150882=CARTESIAN_POINT ( 'NONE',  ( 8.004588480676682494, -26.62287193706184496, 139.9999999999999716 ) ) ;
#150939=CARTESIAN_POINT ( 'NONE',  ( -17.81289503416611097, -24.51734667627696496, 146.2999999999999829 ) ) ;
#150954=CARTESIAN_POINT ( 'NONE',  ( 19.83801684532465615, -12.12952959760455585, 169.9999999999999716 ) ) ;
#150971=CARTESIAN_POINT ( 'NONE',  ( -25.25560589046783733, 4.310829775027161581, 167.9999999999999716 ) ) ;
#151090=CARTESIAN_POINT ( 'NONE',  ( 22.44159573604009594, -16.30477369853687364, 147.6750000027311671 ) ) ;
#151131=ORIENTED_EDGE ( 'NONE', *, *, #49707, .F. ) ;
#151281=CARTESIAN_POINT ( 'NONE',  ( -22.44159573604009950, -16.30477369853688430, 143.5750000027311728 ) ) ;
#151321=CARTESIAN_POINT ( 'NONE',  ( -25.66129429279898844, -9.008087060823562808, 171.3163768196905323 ) ) ;
#151457=CARTESIAN_POINT ( 'NONE',  ( -21.93187539022925847, 6.436421874423674083, 171.3066408880984852 ) ) ;
#151508=EDGE_CURVE ( 'NONE', #37352, #162114, #82102, .T. ) ;
#151547=DIRECTION ( 'NONE',  ( 0.000000000000000000, -0.9945218953682734009, 0.1045284632676537068 ) ) ;
#151622=CARTESIAN_POINT ( 'NONE',  ( 27.73933785331498925, -9.013057229001033122, 147.7750000027311899 ) ) ;
#151661=FACE_OUTER_BOUND ( 'NONE', #10508, .T. ) ;
#151698=ORIENTED_EDGE ( 'NONE', *, *, #148158, .F. ) ;
#151780=CARTESIAN_POINT ( 'NONE',  ( 8.571926809382603096, -26.38167802310801235, 145.4750000027311785 ) ) ;
#151783=EDGE_LOOP ( 'NONE', ( #162646, #159454, #84481, #91300 ) ) ;
#151816=ORIENTED_EDGE ( 'NONE', *, *, #31673, .T. ) ;
#151859=CARTESIAN_POINT ( 'NONE',  ( -21.37649426270061426, -18.77044942199658806, 140.0000000000000568 ) ) ;
#151901=ORIENTED_EDGE ( 'NONE', *, *, #4039, .F. ) ;
#151916=CARTESIAN_POINT ( 'NONE',  ( 17.81289503416611453, -24.51734667627695785, 142.6999999999999886 ) ) ;
#151956=AXIS2_PLACEMENT_3D ( 'NONE', #196621, #179460, #100581 ) ;
#152015=CARTESIAN_POINT ( 'NONE',  ( -24.86035471869060842, -4.680034064337221800, 169.8578160361097105 ) ) ;
#152192=ORIENTED_EDGE ( 'NONE', *, *, #102808, .F. ) ;
#152205=CARTESIAN_POINT ( 'NONE',  ( 26.56065628307859683, -7.402157598701552210, 155.5832749335749270 ) ) ;
#152259=CARTESIAN_POINT ( 'NONE',  ( -22.44159573604010305, 16.30477369853692338, 145.1750000027311671 ) ) ;
#152263=CARTESIAN_POINT ( 'NONE',  ( 22.44159573604009594, -16.30477369853687364, 144.1750000027311671 ) ) ;
#152300=CARTESIAN_POINT ( 'NONE',  ( -26.68407921138531336, -3.932373394476914807, 171.8653659962664619 ) ) ;
#152461=CARTESIAN_POINT ( 'NONE',  ( -17.79613651744293890, -24.49428055684528260, 144.5656553485623874 ) ) ;
#152517=CARTESIAN_POINT ( 'NONE',  ( 24.75981654686065170, -6.635759577896797268, 167.9384007923203512 ) ) ;
#152595=CARTESIAN_POINT ( 'NONE',  ( 22.44159573604009239, 16.30477369853692693, 144.0750000027311728 ) ) ;
#152653=CARTESIAN_POINT ( 'NONE',  ( -8.898068258721474777, 27.38543819252877398, 141.8656553485623704 ) ) ;
#152669=EDGE_CURVE ( 'NONE', #135262, #9294, #192604, .T. ) ;
#152682=CARTESIAN_POINT ( 'NONE',  ( -27.96122637818069023, 7.045120623242314473, 161.2893955982185048 ) ) ;
#152722=VECTOR ( 'NONE', #31842, 1000.000000000000000 ) ;
#152755=CARTESIAN_POINT ( 'NONE',  ( -3.573655867282028392E-15, 2.428612866367529932E-14, 167.9999999999999716 ) ) ;
#152757=CARTESIAN_POINT ( 'NONE',  ( 22.44159573604009239, 16.30477369853692693, 144.0750000027311728 ) ) ;
#152807=CARTESIAN_POINT ( 'NONE',  ( -24.13306144861384084, 5.795830589372935826, 189.9999999999999716 ) ) ;
#152880=CARTESIAN_POINT ( 'NONE',  ( 25.73063820182081685, 8.702599028576305074, 171.6270364942766946 ) ) ;
#152893=CARTESIAN_POINT ( 'NONE',  ( 17.81289503416611453, -24.51734667627695785, 140.6999999999999602 ) ) ;
#152969=EDGE_LOOP ( 'NONE', ( #122545, #151901, #104232 ) ) ;
#153015=ADVANCED_FACE ( 'NONE', ( #81798 ), #31605, .F. ) ;
#153158=CARTESIAN_POINT ( 'NONE',  ( 25.64061671795035124, 10.58440545630783269, 139.9999999999999716 ) ) ;
#153179=ORIENTED_EDGE ( 'NONE', *, *, #110272, .T. ) ;
#153240=CARTESIAN_POINT ( 'NONE',  ( 27.73933785331498925, -9.013057229001033122, 142.2750000027311899 ) ) ;
#153244=CARTESIAN_POINT ( 'NONE',  ( 22.44159573604009594, -16.30477369853687364, 146.1750000027311671 ) ) ;
#153283=CARTESIAN_POINT ( 'NONE',  ( -25.41223161463591040, -11.66315983254872712, 166.2610598689585117 ) ) ;
#153453=CARTESIAN_POINT ( 'NONE',  ( 23.29544513554940366, -16.92513159979222337, 145.0656553485623590 ) ) ;
#153481=CARTESIAN_POINT ( 'NONE',  ( -3.573655867282028392E-15, 2.428612866367529932E-14, 149.6527036446661327 ) ) ;
#153488=CARTESIAN_POINT ( 'NONE',  ( -19.76513836702804738, 12.18681594171306060, 170.0000000000000000 ) ) ;
#153589=CARTESIAN_POINT ( 'NONE',  ( 1.784210473542230573E-15, -29.16686587814331588, 145.3750000027311842 ) ) ;
#153630=CARTESIAN_POINT ( 'NONE',  ( -27.88129983271673851, -6.733757357603135318, 162.1517353552107750 ) ) ;
#153682=CARTESIAN_POINT ( 'NONE',  ( -25.41627434887079673, -11.65185368830121604, 166.2643564577822985 ) ) ;
#153727=CARTESIAN_POINT ( 'NONE',  ( 27.74069374691376311, -6.311165852667638632, 163.4895129000218503 ) ) ;
#153732=LINE ( 'NONE', #187089, #56712 ) ;
#153755=CARTESIAN_POINT ( 'NONE',  ( 1.784210473542230573E-15, -29.16686587814331588, 143.3750000027311557 ) ) ;
#153769=CARTESIAN_POINT ( 'NONE',  ( -3.573655867282028392E-15, 2.428612866367529932E-14, 155.0000000000000000 ) ) ;
#153835=CARTESIAN_POINT ( 'NONE',  ( -0.2989490121399997480, -27.96601393914107803, 140.0000000000000853 ) ) ;
#153880=ORIENTED_EDGE ( 'NONE', *, *, #172144, .T. ) ;
#153895=CARTESIAN_POINT ( 'NONE',  ( 17.81289503416610742, 24.51734667627700404, 145.2999999999999829 ) ) ;
#154032=AXIS2_PLACEMENT_3D ( 'NONE', #185566, #15724, #166686 ) ;
#154054=CARTESIAN_POINT ( 'NONE',  ( -26.58496454516998853, -7.626754437231455519, 167.9682100371138915 ) ) ;
#154086=CARTESIAN_POINT ( 'NONE',  ( 28.85599147140293752, 2.428612866367529932E-14, 149.6527036446661327 ) ) ;
#154246=CARTESIAN_POINT ( 'NONE',  ( 1.784210473542230573E-15, -29.16686587814331588, 143.8750000027311557 ) ) ;
#154250=CARTESIAN_POINT ( 'NONE',  ( 1.784210473542230573E-15, -29.16686587814331588, 143.8750000027311557 ) ) ;
#154286=CARTESIAN_POINT ( 'NONE',  ( -25.93326183087831893, -10.28624940747432959, 166.6531433017871962 ) ) ;
#154314=EDGE_LOOP ( 'NONE', ( #194274, #144214, #117578, #179283, #81227, #122892 ) ) ;
#154335=CARTESIAN_POINT ( 'NONE',  ( -29.17999648465609397, -8.032454009542489004, 149.7954620931811291 ) ) ;
#154467=CARTESIAN_POINT ( 'NONE',  ( -23.27014042476074707, -11.64952740454485003, 165.7333935355015626 ) ) ;
#154525=CARTESIAN_POINT ( 'NONE',  ( -22.78714015945951132, 11.73760554535606104, 167.9671921004704132 ) ) ;
#154536=ADVANCED_FACE ( 'NONE', ( #75626 ), #182830, .T. ) ;
#154589=CARTESIAN_POINT ( 'NONE',  ( 17.14385361876520264, 23.59649016807275856, 148.1750000027311955 ) ) ;
#154661=ORIENTED_EDGE ( 'NONE', *, *, #2143, .T. ) ;
#154665=CARTESIAN_POINT ( 'NONE',  ( 28.79475375365586132, 2.781246896534039337E-14, 142.9843446568999639 ) ) ;
#154678=CARTESIAN_POINT ( 'NONE',  ( -25.25560589046783733, 2.428612866367529932E-14, 167.9999999999999716 ) ) ;
#154688=CARTESIAN_POINT ( 'NONE',  ( 22.96528548301342809, -5.795830589372932273, 190.0000000000000000 ) ) ;
#154753=CARTESIAN_POINT ( 'NONE',  ( -5.359611314223446995E-15, 29.16686587814335496, 142.3750000027311557 ) ) ;
#154881=CARTESIAN_POINT ( 'NONE',  ( -21.54612633733209748, -7.439814990120659388, 174.3585332542294566 ) ) ;
#154890=CARTESIAN_POINT ( 'NONE',  ( -23.31738231874055600, 16.94106989632528837, 143.7999999999999829 ) ) ;
#154902=CARTESIAN_POINT ( 'NONE',  ( 25.80209238092669466, -7.370998251474716767, 174.5109820657625050 ) ) ;
#154908=( NAMED_UNIT ( * ) PLANE_ANGLE_UNIT ( ) SI_UNIT ( $, .RADIAN. ) );
#154956=CARTESIAN_POINT ( 'NONE',  ( -25.22509938781154304, 6.326560822155829378, 165.8168946714179128 ) ) ;
#154986=CARTESIAN_POINT ( 'NONE',  ( -24.06756124613667680, -8.142616467496756272, 169.4332804344566057 ) ) ;
#155025=CARTESIAN_POINT ( 'NONE',  ( -24.93942350307309752, -7.769968609432603479, 171.2173313942149662 ) ) ;
#155178=EDGE_CURVE ( 'NONE', #79565, #75891, #66583, .T. ) ;
#155192=DIRECTION ( 'NONE',  ( -0.5367108174878557625, 0.8437662581494461689, 1.463701136248949969E-16 ) ) ;
#155243=CARTESIAN_POINT ( 'NONE',  ( -8.571926809382608425, 26.38167802310805854, 144.9750000027312069 ) ) ;
#155416=VERTEX_POINT ( 'NONE', #112919 ) ;
#155432=CARTESIAN_POINT ( 'NONE',  ( -12.72656435003161235, 25.68303923411528800, 139.9999999999999432 ) ) ;
#155481=CARTESIAN_POINT ( 'NONE',  ( -21.97181142354054018, 8.379174292515184419, 172.0076905927031419 ) ) ;
#155519=CARTESIAN_POINT ( 'NONE',  ( -21.04946095171203169, 10.24435024061036437, 168.3368280404225459 ) ) ;
#155583=CARTESIAN_POINT ( 'NONE',  ( 1.784210473542230573E-15, -29.16686587814331588, 141.3750000027311557 ) ) ;
#155605=AXIS2_PLACEMENT_3D ( 'NONE', #103293, #44603, #10294 ) ;
#155621=CARTESIAN_POINT ( 'NONE',  ( 24.93942350307308686, 7.769968609432599926, 171.2173313942149946 ) ) ;
#155738=EDGE_CURVE ( 'NONE', #144934, #146461, #163323, .T. ) ;
#155880=CARTESIAN_POINT ( 'NONE',  ( -28.82186960331499392, -9.364793116373526516, 140.0999999999999943 ) ) ;
#155893=CARTESIAN_POINT ( 'NONE',  ( 25.66129429279841290, -9.008087060820539449, 171.3163768196949945 ) ) ;
#155900=CARTESIAN_POINT ( 'NONE',  ( 21.49230329115315286, -7.461674882483882776, 174.1505502713556837 ) ) ;
#155976=CARTESIAN_POINT ( 'NONE',  ( -28.82186960331499037, 2.428612866367529932E-14, 146.2500000054623683 ) ) ;
#155993=CARTESIAN_POINT ( 'NONE',  ( -27.73933785331498925, 9.013057229001088189, 147.2750000027311614 ) ) ;
#156014=CARTESIAN_POINT ( 'NONE',  ( 26.58496454516998142, -7.626754437231455519, 167.9682100371138915 ) ) ;
#156267=CARTESIAN_POINT ( 'NONE',  ( -25.76143648877098968, -7.343476467573589517, 174.8772314887148696 ) ) ;
#156285=ADVANCED_FACE ( 'NONE', ( #98387 ), #68575, .T. ) ;
#156296=ORIENTED_EDGE ( 'NONE', *, *, #193877, .T. ) ;
#156409=EDGE_LOOP ( 'NONE', ( #72623, #25657, #86298, #85776, #35330, #179652, #175746, #119127 ) ) ;
#156464=CARTESIAN_POINT ( 'NONE',  ( 26.11842041226233846, 7.699311778675188123, 169.4341694154020956 ) ) ;
#156516=CARTESIAN_POINT ( 'NONE',  ( -24.02130208663010791, 8.352503713166791854, 169.2769999910313174 ) ) ;
#156538=ORIENTED_EDGE ( 'NONE', *, *, #122945, .F. ) ;
#156558=DIRECTION ( 'NONE',  ( 0.000000000000000000, 0.000000000000000000, -1.000000000000000000 ) ) ;
#156587=CARTESIAN_POINT ( 'NONE',  ( -5.359611314223446995E-15, 29.16686587814335496, 142.3750000027311557 ) ) ;
#156602=CARTESIAN_POINT ( 'NONE',  ( -26.03370437638690049, -6.875205692009850544, 160.5968874236872637 ) ) ;
#156624=CARTESIAN_POINT ( 'NONE',  ( 23.58953014017657779, 7.613468834709956390, 172.7063272879298950 ) ) ;
#156724=CARTESIAN_POINT ( 'NONE',  ( 26.03370437638690049, -6.875205692009868308, 160.5968874236871784 ) ) ;
#156818=CARTESIAN_POINT ( 'NONE',  ( 22.78714015945950422, 11.73760554535660638, 167.9671921004704416 ) ) ;
#156877=CARTESIAN_POINT ( 'NONE',  ( -26.45595770381631340, 7.620359626981985990, 168.5711898564603359 ) ) ;
#156900=CARTESIAN_POINT ( 'NONE',  ( 20.93662873023657411, -11.00447265502299388, 170.1964094900432372 ) ) ;
#156906=CARTESIAN_POINT ( 'NONE',  ( 21.16427095311446038, -10.71512246325695550, 170.2843762835011319 ) ) ;
#156917=DIRECTION ( 'NONE',  ( -0.5367108174878556515, 0.8437662581494462799, -7.967771471296434353E-17 ) ) ;
#156978=CARTESIAN_POINT ( 'NONE',  ( -5.429308488886486681E-15, 30.30510711980690175, 145.7500000054623115 ) ) ;
#156991=CARTESIAN_POINT ( 'NONE',  ( -5.359611314223446995E-15, 29.16686587814335851, 146.8750000027311557 ) ) ;
#157069=CIRCLE ( 'NONE', #73104, 3.000000000000001332 ) ;
#157145=CARTESIAN_POINT ( 'NONE',  ( -19.30190589895974185, 21.36759865781276346, 139.9999999999999716 ) ) ;
#157379=DIRECTION ( 'NONE',  ( -1.000000000000000000, 0.000000000000000000, 0.000000000000000000 ) ) ;
#157458=ORIENTED_EDGE ( 'NONE', *, *, #38420, .T. ) ;
#157463=CARTESIAN_POINT ( 'NONE',  ( 25.66012929990208136, 7.783344152590474962, 170.2244316400881701 ) ) ;
#157514=CARTESIAN_POINT ( 'NONE',  ( -23.62199046085639864, 10.84149981712537603, 165.9137635136253266 ) ) ;
#157579=CARTESIAN_POINT ( 'NONE',  ( 8.571926809382597767, 26.38167802310806209, 140.2750000027311899 ) ) ;
#157745=CARTESIAN_POINT ( 'NONE',  ( -22.44159573604010305, 16.30477369853692338, 140.6750000027311671 ) ) ;
#157809=CARTESIAN_POINT ( 'NONE',  ( 24.02130208662955013, 8.352503713167605426, 169.2769999910313174 ) ) ;
#157893=CARTESIAN_POINT ( 'NONE',  ( 26.68407921138530625, -3.932373394476913919, 171.8653659962664619 ) ) ;
#157969=CARTESIAN_POINT ( 'NONE',  ( -8.906447517083060816, 27.41122689804195645, 147.8500000054623627 ) ) ;
#157975=VECTOR ( 'NONE', #63663, 1000.000000000000000 ) ;
#158050=FACE_OUTER_BOUND ( 'NONE', #81231, .T. ) ;
#158057=CARTESIAN_POINT ( 'NONE',  ( 28.79475375365494116, -9.355982642740455546, 143.1656553485623533 ) ) ;
#158124=CARTESIAN_POINT ( 'NONE',  ( 21.38418241377623019, -5.438282248597753110, 174.2683007571264113 ) ) ;
#158217=DIRECTION ( 'NONE',  ( -0.000000000000000000, -0.000000000000000000, -1.000000000000000000 ) ) ;
#158273=LINE ( 'NONE', #19762, #106632 ) ;
#158282=VERTEX_POINT ( 'NONE', #129726 ) ;
#158362=CARTESIAN_POINT ( 'NONE',  ( -3.573655867282028392E-15, 2.428612866367529932E-14, 155.0000000000000000 ) ) ;
#158392=ORIENTED_EDGE ( 'NONE', *, *, #77698, .T. ) ;
#158497=CARTESIAN_POINT ( 'NONE',  ( -24.20757866959954541, 5.698759791480812353, 172.9004493943157570 ) ) ;
#158534=CARTESIAN_POINT ( 'NONE',  ( -3.573655867282028392E-15, 2.428612866367529932E-14, 150.0000000000000000 ) ) ;
#158573=CARTESIAN_POINT ( 'NONE',  ( 27.79722099587822370, -7.618187661584347126, 161.3616444162216226 ) ) ;
#158667=FACE_OUTER_BOUND ( 'NONE', #82001, .T. ) ;
#158719=CARTESIAN_POINT ( 'NONE',  ( 27.73933785331498569, 2.768321779492822058E-14, 139.8750000027311842 ) ) ;
#158723=B_SPLINE_CURVE_WITH_KNOTS ( 'NONE', 3,
 ( #134720, #198361, #196403, #121505, #150882, #44681, #181228, #42704, #142, #58846, #153835, #104365, #122497, #106334, #12377, #74039, #135710, #168020, #29516, #120513, #182205, #199358, #43689, #105351, #167038, #168994, #28540, #151859, #164632, #54449, #179816, #39278, #118128, #84763, #70622, #26127, #41286, #83766, #132288, #161624 ),
 .UNSPECIFIED., .F., .F.,
 ( 4, 2, 2, 2, 2, 2, 2, 2, 2, 2, 2, 2, 2, 2, 2, 2, 2, 2, 2, 4 ),
 ( 0.000000000000000000, 0.001704564650157686578, 0.003409129300315373156, 0.006818258600630746312, 0.01022738790094612077, 0.01193195255110380756, 0.01363651720126149262, 0.02045477580189224154, 0.02215934045204992833, 0.02386390510220762207, 0.02727303440252299219, 0.03068216370283836578, 0.03238672835299604563, 0.03409129300315372202, 0.03750042230346907479, 0.04090955160378442756, 0.04772781020441514005, 0.04943237485457282337, 0.05113693950473050670, 0.05454606880504585253 ),
 .UNSPECIFIED. ) ;
#158784=CARTESIAN_POINT ( 'NONE',  ( 23.19706360625337993, 11.80427776162510156, 165.7059442611694067 ) ) ;
#158869=CARTESIAN_POINT ( 'NONE',  ( 21.84611564451294541, -9.363109600221314111, 171.0247306346274172 ) ) ;
#158893=CARTESIAN_POINT ( 'NONE',  ( -8.571926809382601320, -26.38167802310801591, 141.2750000027311899 ) ) ;
#158915=( BOUNDED_CURVE ( )  B_SPLINE_CURVE ( 3, ( #167988, #152807, #90143, #138627 ),
 .UNSPECIFIED., .F., .F. ) 
 B_SPLINE_CURVE_WITH_KNOTS ( ( 4, 4 ),
 ( 5.503250352303675541, 7.063120262055497811 ),
 .UNSPECIFIED. ) 
 CURVE ( )  GEOMETRIC_REPRESENTATION_ITEM ( )  RATIONAL_B_SPLINE_CURVE ( ( 1.000000000000000000, 0.8073061876036302653, 0.8073061876036302653, 1.000000000000000000 ) ) 
 REPRESENTATION_ITEM ( '' )  );
#158948=CARTESIAN_POINT ( 'NONE',  ( -27.73933785331498925, -9.013057229001049109, 147.4750000027311785 ) ) ;
#158949=CARTESIAN_POINT ( 'NONE',  ( 28.82186960331499392, -9.364793116373510529, 147.1500000054623456 ) ) ;
#159009=LINE ( 'NONE', #81166, #198543 ) ;
#159029=DIRECTION ( 'NONE',  ( -1.000000000000000000, -0.000000000000000000, 0.000000000000000000 ) ) ;
#159261=EDGE_LOOP ( 'NONE', ( #116818, #43071, #3499, #184892 ) ) ;
#159341=EDGE_CURVE ( 'NONE', #181921, #146141, #56185, .T. ) ;
#159352=CARTESIAN_POINT ( 'NONE',  ( 25.41560487745633168, -11.65347601360406848, 166.2639678467665760 ) ) ;
#159393=CARTESIAN_POINT ( 'NONE',  ( 27.91252812236343317, 7.473505457733358170, 160.9450913315119180 ) ) ;
#159439=CARTESIAN_POINT ( 'NONE',  ( -22.24685556490157623, -12.75834802357607600, 167.9013491530738520 ) ) ;
#159454=ORIENTED_EDGE ( 'NONE', *, *, #13191, .T. ) ;
#159784=CARTESIAN_POINT ( 'NONE',  ( 23.62199046085638088, 10.84149981712535471, 165.9137635136254119 ) ) ;
#159901=CARTESIAN_POINT ( 'NONE',  ( 1.784210473542230573E-15, -29.16686587814331588, 143.3750000027311557 ) ) ;
#159955=CARTESIAN_POINT ( 'NONE',  ( -27.73933785331498925, -9.013057229001049109, 141.4750000027311785 ) ) ;
#159956=EDGE_CURVE ( 'NONE', #2773, #135939, #193717, .T. ) ;
#159957=CARTESIAN_POINT ( 'NONE',  ( 28.82186960331498327, 9.364793116373570925, 145.3500000054623627 ) ) ;
#159959=CARTESIAN_POINT ( 'NONE',  ( -27.05641397906351742, 3.631740835637567333, 169.9999999999999716 ) ) ;
#159970=CARTESIAN_POINT ( 'NONE',  ( 8.571926809382597767, 26.38167802310806209, 140.7750000027311899 ) ) ;
#160045=CARTESIAN_POINT ( 'NONE',  ( 8.898068258721473001, -27.38543819252872069, 142.8656553485623704 ) ) ;
#160210=DIRECTION ( 'NONE',  ( -1.000000000000000000, 0.000000000000000000, 0.000000000000000000 ) ) ;
#160230=AXIS2_PLACEMENT_3D ( 'NONE', #170111, #199466, #93255 ) ;
#160380=ORIENTED_EDGE ( 'NONE', *, *, #171523, .T. ) ;
#160431=CARTESIAN_POINT ( 'NONE',  ( -24.79445957992282601, 6.337972767934357599, 168.1743082258863353 ) ) ;
#160451=CARTESIAN_POINT ( 'NONE',  ( -23.62199046085637733, -10.84149981712538136, 165.9137635136253266 ) ) ;
#160531=DIRECTION ( 'NONE',  ( -1.000000000000000000, 0.000000000000000000, 0.000000000000000000 ) ) ;
#160573=CARTESIAN_POINT ( 'NONE',  ( 26.70613957415102035, -7.662257527287521519, 167.2521143936660906 ) ) ;
#160594=CARTESIAN_POINT ( 'NONE',  ( 21.70980307670622267, 7.452553642297959691, 174.2373330747591638 ) ) ;
#160638=CARTESIAN_POINT ( 'NONE',  ( 22.87925077421024511, 5.621762139875928099, 172.5226062014847059 ) ) ;
#160693=DIRECTION ( 'NONE',  ( -1.000000000000000000, 0.000000000000000000, 0.000000000000000000 ) ) ;
#160794=CARTESIAN_POINT ( 'NONE',  ( 21.70479006154310397, 8.695791278452436046, 169.0563666577073150 ) ) ;
#160855=ORIENTED_EDGE ( 'NONE', *, *, #24918, .F. ) ;
#160903=CARTESIAN_POINT ( 'NONE',  ( -22.44159573604010305, 16.30477369853692338, 142.6750000027311671 ) ) ;
#160927=EDGE_CURVE ( 'NONE', #107606, #148762, #131019, .T. ) ;
#160957=CARTESIAN_POINT ( 'NONE',  ( 22.44159573604009239, 16.30477369853692693, 140.5750000027311728 ) ) ;
#160958=CARTESIAN_POINT ( 'NONE',  ( 28.82186960331498327, 9.364793116373570925, 139.3500000054623911 ) ) ;
#160971=CARTESIAN_POINT ( 'NONE',  ( 27.73933785331498569, 9.013057229001093518, 140.4750000027312069 ) ) ;
#160998=EDGE_CURVE ( 'NONE', #37352, #31966, #66207, .T. ) ;
#161018=CARTESIAN_POINT ( 'NONE',  ( 26.79475375365586132, 2.756753960551091991E-14, 155.0000000000000000 ) ) ;
#161041=CARTESIAN_POINT ( 'NONE',  ( -26.73207562759454703, 6.543912086049501475, 168.7462576975894422 ) ) ;
#161083=CARTESIAN_POINT ( 'NONE',  ( 26.45594755429568323, 8.318738267476192050, 167.5492909577866385 ) ) ;
#161173=ORIENTED_EDGE ( 'NONE', *, *, #1535, .F. ) ;
#161181=CARTESIAN_POINT ( 'NONE',  ( -24.84743926645693080, 12.91388972341062136, 166.0204189386425639 ) ) ;
#161272=EDGE_LOOP ( 'NONE', ( #33365, #55965, #71325, #31870 ) ) ;
#161382=PLANE ( 'NONE',  #146596 ) ;
#161451=CARTESIAN_POINT ( 'NONE',  ( -20.93662873023658122, -10.44628751056252369, 168.2749732860604013 ) ) ;
#161491=CARTESIAN_POINT ( 'NONE',  ( 24.27995301597375288, -6.552671593954494611, 171.1165850637241874 ) ) ;
#161535=CARTESIAN_POINT ( 'NONE',  ( 23.84689744903973008, 10.26551614244696076, 166.0764362378396868 ) ) ;
#161571=CARTESIAN_POINT ( 'NONE',  ( 27.20489923017583322, -7.754340368643432235, 164.3890803562161977 ) ) ;
#161591=CARTESIAN_POINT ( 'NONE',  ( 21.93208748025632104, 6.437649280788581230, 171.3046185016227696 ) ) ;
#161616=AXIS2_PLACEMENT_3D ( 'NONE', #87360, #38866, #37863 ) ;
#161624=CARTESIAN_POINT ( 'NONE',  ( -28.75808110634262604, -1.452795517301058048, 139.9999999999999716 ) ) ;
#161702=ORIENTED_EDGE ( 'NONE', *, *, #194670, .T. ) ;
#161777=DIRECTION ( 'NONE',  ( 1.000000000000000000, 0.000000000000000000, 0.000000000000000000 ) ) ;
#161852=ORIENTED_EDGE ( 'NONE', *, *, #36961, .F. ) ;
#161901=CARTESIAN_POINT ( 'NONE',  ( -5.359611314223446995E-15, 29.16686587814335851, 142.3750000027311557 ) ) ;
#161907=ORIENTED_EDGE ( 'NONE', *, *, #17982, .T. ) ;
#161936=ORIENTED_EDGE ( 'NONE', *, *, #123538, .T. ) ;
#161956=CARTESIAN_POINT ( 'NONE',  ( -28.82186960331499037, 2.428612866367529932E-14, 142.2500000054623683 ) ) ;
#161969=CARTESIAN_POINT ( 'NONE',  ( -22.44159573604010305, 16.30477369853692338, 145.1750000027311671 ) ) ;
#162027=DIRECTION ( 'NONE',  ( 1.000000000000000000, 0.000000000000000000, 0.000000000000000000 ) ) ;
#162040=FACE_OUTER_BOUND ( 'NONE', #173632, .T. ) ;
#162041=CARTESIAN_POINT ( 'NONE',  ( -25.27727188472089637, 10.29814791481115321, 170.4127952078933390 ) ) ;
#162076=ADVANCED_FACE ( 'NONE', ( #89176 ), #134541, .F. ) ;
#162084=VERTEX_POINT ( 'NONE', #135695 ) ;
#162086=CARTESIAN_POINT ( 'NONE',  ( 25.04733094907663116, 10.92720321514006621, 170.1247377027656853 ) ) ;
#162097=CARTESIAN_POINT ( 'NONE',  ( -17.14385361876520619, 23.59649016807275856, 141.0750000027311728 ) ) ;
#162114=VERTEX_POINT ( 'NONE', #131694 ) ;
#162124=CARTESIAN_POINT ( 'NONE',  ( -19.49401214000077687, 12.39993551617566681, 164.9999999999999716 ) ) ;
#162141=EDGE_CURVE ( 'NONE', #35378, #131506, #197367, .T. ) ;
#162174=ORIENTED_EDGE ( 'NONE', *, *, #35192, .F. ) ;
#162246=EDGE_CURVE ( 'NONE', #135144, #158282, #140689, .T. ) ;
#162444=CARTESIAN_POINT ( 'NONE',  ( -21.51693143705271893, -9.260949364272990536, 168.7281092719938442 ) ) ;
#162480=CARTESIAN_POINT ( 'NONE',  ( 24.24385185424179667, -7.025880200331696024, 170.5073520790474788 ) ) ;
#162569=TOROIDAL_SURFACE ( 'NONE', #75405, 23.10356920737165254, 5.000000000000000000 ) ;
#162585=CARTESIAN_POINT ( 'NONE',  ( 20.09068217638368736, 11.70722341973408120, 168.0245402885401518 ) ) ;
#162615=ORIENTED_EDGE ( 'NONE', *, *, #33729, .T. ) ;
#162646=ORIENTED_EDGE ( 'NONE', *, *, #121993, .T. ) ;
#162665=FACE_OUTER_BOUND ( 'NONE', #37826, .T. ) ;
#162693=EDGE_LOOP ( 'NONE', ( #197302, #167080, #48705, #110965 ) ) ;
#162721=CIRCLE ( 'NONE', #130361, 30.82560697742735556 ) ;
#162772=CARTESIAN_POINT ( 'NONE',  ( -26.82869043059639225, -7.693057566823084947, 166.5358880480777941 ) ) ;
#162845=ORIENTED_EDGE ( 'NONE', *, *, #48174, .T. ) ;
#162958=CARTESIAN_POINT ( 'NONE',  ( 28.82186960331498327, 2.781578969918950771E-14, 139.2500000054623683 ) ) ;
#162972=CARTESIAN_POINT ( 'NONE',  ( 8.571926809382597767, 26.38167802310806209, 144.7750000027311899 ) ) ;
#163028=CARTESIAN_POINT ( 'NONE',  ( -25.38276140623241162, -4.833717845876328134, 166.7901960806511852 ) ) ;
#163042=CARTESIAN_POINT ( 'NONE',  ( -25.04733094907774316, 10.92720321514004489, 170.1247377027656569 ) ) ;
#163087=CARTESIAN_POINT ( 'NONE',  ( 25.34721418589430186, 10.09305078451787629, 170.5222919391072764 ) ) ;
#163100=CARTESIAN_POINT ( 'NONE',  ( -28.82186960331499037, 2.428612866367529932E-14, 146.0000000000000000 ) ) ;
#163154=CARTESIAN_POINT ( 'NONE',  ( 24.13306144861383729, -5.795830589372934050, 189.9999999999999716 ) ) ;
#163225=VECTOR ( 'NONE', #110400, 1000.000000000000000 ) ;
#163247=CARTESIAN_POINT ( 'NONE',  ( -19.80313217313587160, -12.05975691044382359, 167.9999999999999716 ) ) ;
#163260=CARTESIAN_POINT ( 'NONE',  ( -27.73933785331498925, 9.013057229001088189, 146.7750000027311899 ) ) ;
#163323=B_SPLINE_CURVE_WITH_KNOTS ( 'NONE', 3,
 ( #128084, #160431, #192772, #6732, #100741, #54256, #98738, #19922, #81564, #97728, #143250, #4734, #68410, #82572 ),
 .UNSPECIFIED., .F., .F.,
 ( 4, 2, 2, 2, 2, 2, 4 ),
 ( 0.1559601203333475239, 0.1570958510570476530, 0.1582315817807478098, 0.1605030432281480957, 0.1616387739518482247, 0.1627745046755483815, 0.1650459661229486397 ),
 .UNSPECIFIED. ) ;
#163400=EDGE_CURVE ( 'NONE', #184349, #177366, #34462, .T. ) ;
#163401=CARTESIAN_POINT ( 'NONE',  ( -5.427562675786936573E-15, 30.27659582821221207, 147.4843446568999923 ) ) ;
#163454=CARTESIAN_POINT ( 'NONE',  ( -17.14385361876520619, 23.59649016807275856, 147.0750000027311728 ) ) ;
#163464=ADVANCED_FACE ( 'NONE', ( #190136 ), #183744, .F. ) ;
#163476=ORIENTED_EDGE ( 'NONE', *, *, #7692, .T. ) ;
#163498=CARTESIAN_POINT ( 'NONE',  ( 21.81230582904620618, -5.969922009378142214, 172.1979875755925775 ) ) ;
#163599=CARTESIAN_POINT ( 'NONE',  ( 21.82220748998222959, 8.288476145941624296, 169.3167957967150414 ) ) ;
#163724=CARTESIAN_POINT ( 'NONE',  ( -17.79613651744293890, -24.49428055684527550, 146.2843446568999752 ) ) ;
#163738=FACE_OUTER_BOUND ( 'NONE', #170283, .T. ) ;
#163803=CARTESIAN_POINT ( 'NONE',  ( 24.20757866959953120, 5.698759791481088577, 172.9004493943157570 ) ) ;
#163852=CIRCLE ( 'NONE', #134844, 28.02760797243269408 ) ;
#163902=CARTESIAN_POINT ( 'NONE',  ( -27.96779038917889793, 7.241162895362913687, 160.9774814432332164 ) ) ;
#163978=CARTESIAN_POINT ( 'NONE',  ( -17.81289503416611097, -24.51734667627696496, 138.5500000054623229 ) ) ;
#163981=VERTEX_POINT ( 'NONE', #13109 ) ;
#163990=CARTESIAN_POINT ( 'NONE',  ( -5.359611314223446995E-15, 29.16686587814335851, 144.8750000027311842 ) ) ;
#164012=CARTESIAN_POINT ( 'NONE',  ( 25.25560589046783022, 4.310829775027161581, 167.9999999999999716 ) ) ;
#164021=PLANE ( 'NONE',  #187160 ) ;
#164060=CARTESIAN_POINT ( 'NONE',  ( -23.35043118190705869, 14.19381810411928235, 169.8796877288295946 ) ) ;
#164100=ORIENTED_EDGE ( 'NONE', *, *, #133168, .F. ) ;
#164112=CARTESIAN_POINT ( 'NONE',  ( -27.73933785331498925, 2.428612866367529932E-14, 139.3750000027311842 ) ) ;
#164239=EDGE_CURVE ( 'NONE', #60981, #163981, #133164, .T. ) ;
#164252=CARTESIAN_POINT ( 'NONE',  ( -24.40828949532295056, 2.848420800297980726, 173.9378174459542947 ) ) ;
#164257=CARTESIAN_POINT ( 'NONE',  ( -20.09068217638366960, -11.70722341973408476, 168.0245402885401234 ) ) ;
#164270=CARTESIAN_POINT ( 'NONE',  ( -22.44159573604010305, 16.30477369853692338, 144.6750000027311671 ) ) ;
#164372=APPLICATION_CONTEXT ( 'automotive_design' ) ;
#164395=ORIENTED_EDGE ( 'NONE', *, *, #126480, .F. ) ;
#164500=CARTESIAN_POINT ( 'NONE',  ( 24.04614410381781653, -5.408324479810879382, 174.2944578187869240 ) ) ;
#164600=CARTESIAN_POINT ( 'NONE',  ( 21.96449396329681392, 6.689387493872144930, 170.9254202302468570 ) ) ;
#164632=CARTESIAN_POINT ( 'NONE',  ( -22.11591546058419766, -17.92733262806552474, 140.0000000000000853 ) ) ;
#164634=CARTESIAN_POINT ( 'NONE',  ( -21.65431292632188942, 8.856125861401146437, 168.9593721673316793 ) ) ;
#164651=CARTESIAN_POINT ( 'NONE',  ( 26.58496454516998142, -7.626754437231455519, 167.9682100371138915 ) ) ;
#164699=CARTESIAN_POINT ( 'NONE',  ( -21.92644707618962485, 9.078916001213697129, 171.2473621415418847 ) ) ;
#164705=LINE ( 'NONE', #179891, #105784 ) ;
#164787=CARTESIAN_POINT ( 'NONE',  ( -27.96625882250065942, -7.271219613218503852, 160.9431592986335318 ) ) ;
#164896=CARTESIAN_POINT ( 'NONE',  ( -27.77694149905213905, 7.633451960439542106, 161.4496143021112857 ) ) ;
#164971=CARTESIAN_POINT ( 'NONE',  ( -8.906447517083053711, -27.41122689804191026, 142.6500000054623740 ) ) ;
#165052=CARTESIAN_POINT ( 'NONE',  ( -24.42783677680704102, 12.30119602009721014, 169.8172178118632587 ) ) ;
#165094=CARTESIAN_POINT ( 'NONE',  ( 25.85392304583292145, 7.514126903508385524, 173.7688241862488212 ) ) ;
#165107=CARTESIAN_POINT ( 'NONE',  ( 22.44159573604009239, 16.30477369853692693, 140.5750000027311728 ) ) ;
#165122=LINE ( 'NONE', #92222, #166990 ) ;
#165138=EDGE_CURVE ( 'NONE', #147212, #148543, #189351, .T. ) ;
#165250=CARTESIAN_POINT ( 'NONE',  ( -20.48593134815242323, -11.15862823513540825, 168.1084560298344854 ) ) ;
#165263=CARTESIAN_POINT ( 'NONE',  ( -8.571926809382601320, -26.38167802310801591, 147.2750000027311899 ) ) ;
#165274=CARTESIAN_POINT ( 'NONE',  ( 26.53515902489025535, 7.921333329385870314, 167.7790254135049111 ) ) ;
#165459=( BOUNDED_SURFACE ( )  B_SPLINE_SURFACE ( 3, 2, ( 
 ( #121950, #196838, #76444 ),
 ( #11827, #138121, #45125 ),
 ( #183643, #26991, #43138 ),
 ( #136142, #150332, #73492 ),
 ( #104807, #198812, #60277 ),
 ( #44136, #581, #153283 ),
 ( #47110, #135165, #59284 ),
 ( #14784, #166496, #154286 ),
 ( #77435, #106783, #27994 ),
 ( #197818, #46108, #89633 ),
 ( #169447, #15776, #30949 ),
 ( #119973, #199802, #139107 ),
 ( #168458, #61269, #62252 ),
 ( #165495, #29955, #88636 ),
 ( #122939, #151321, #90618 ),
 ( #12810, #184626, #105795 ),
 ( #137125, #120953, #91593 ),
 ( #123921, #13784, #107762 ),
 ( #185620, #74477, #182652 ),
 ( #167481, #28976, #152300 ),
 ( #75451, #79424, #93592 ),
 ( #128891, #35900, #124938 ),
 ( #48106, #156267, #190591 ),
 ( #19743, #65245, #31938 ) ),
 .UNSPECIFIED., .F., .F., .F. ) 
 B_SPLINE_SURFACE_WITH_KNOTS ( ( 4, 2, 2, 2, 2, 2, 2, 2, 2, 2, 2, 4 ),
 ( 3, 3 ),
 ( 0.000000000000000000, 0.001899702839891690993, 0.002849554259837536706, 0.003799405679783381985, 0.005699108519675073412, 0.006648959939620918691, 0.007598811359566763970, 0.008548662779512609250, 0.009498514199458456264, 0.01139821703935014682, 0.01329791987924183738, 0.01519762271913352794 ),
 ( 0.000000000000000000, 1.000000000000000000 ),
 .UNSPECIFIED. ) 
 GEOMETRIC_REPRESENTATION_ITEM ( )  RATIONAL_B_SPLINE_SURFACE ( (
 ( 1.000000000000000000, 0.7660444431189779024, 1.000000000000000000),
 ( 1.000000000000000000, 0.7753720600382123518, 1.000000000000000000),
 ( 1.000000000000000000, 0.7832595754286273415, 1.000000000000000000),
 ( 1.000000000000000000, 0.7928595458705296473, 1.000000000000000000),
 ( 1.000000000000000000, 0.7956872332516093937, 1.000000000000000000),
 ( 1.000000000000000000, 0.8005750596157590326, 1.000000000000000000),
 ( 1.000000000000000000, 0.8026302056541515517, 1.000000000000000000),
 ( 1.000000000000000000, 0.8075080643848789874, 1.000000000000000000),
 ( 1.000000000000000000, 0.8091143015809036942, 1.000000000000000000),
 ( 1.000000000000000000, 0.8093067629633434734, 1.000000000000000000),
 ( 1.000000000000000000, 0.8089952915731429828, 1.000000000000000000),
 ( 1.000000000000000000, 0.8076919994862520324, 1.000000000000000000),
 ( 1.000000000000000000, 0.8067078407649239669, 1.000000000000000000),
 ( 1.000000000000000000, 0.8041786842467097962, 1.000000000000000000),
 ( 1.000000000000000000, 0.8026334674877428910, 1.000000000000000000),
 ( 1.000000000000000000, 0.7990747329468967930, 1.000000000000000000),
 ( 1.000000000000000000, 0.7970509760942138255, 1.000000000000000000),
 ( 1.000000000000000000, 0.7904793850862680271, 1.000000000000000000),
 ( 1.000000000000000000, 0.7855040224314145947, 1.000000000000000000),
 ( 1.000000000000000000, 0.7751942650507163135, 1.000000000000000000),
 ( 1.000000000000000000, 0.7698260778211021282, 1.000000000000000000),
 ( 1.000000000000000000, 0.7598259884961480193, 1.000000000000000000),
 ( 1.000000000000000000, 0.7551428682219901711, 1.000000000000000000),
 ( 1.000000000000000000, 0.7510191126010862250, 1.000000000000000000) ) ) 
 REPRESENTATION_ITEM ( '' )  SURFACE ( )  );
#165495=CARTESIAN_POINT ( 'NONE',  ( -21.93180397000192272, -9.000796715313676088, 171.3297436093443196 ) ) ;
#165578=ADVANCED_FACE ( 'NONE', ( #4511 ), #190555, .T. ) ;
#165614=DIRECTION ( 'NONE',  ( 0.000000000000000000, 0.000000000000000000, -1.000000000000000000 ) ) ;
#165630=CARTESIAN_POINT ( 'NONE',  ( -21.75476783670602288, 5.835674035550357353, 172.5278397751181387 ) ) ;
#165647=CARTESIAN_POINT ( 'NONE',  ( 25.82634036940374855, -7.758313425001082564, 169.9660385289634235 ) ) ;
#165797=CARTESIAN_POINT ( 'NONE',  ( 24.85114155361847565, 5.582993631601034679, 168.8590791472286412 ) ) ;
#165903=CARTESIAN_POINT ( 'NONE',  ( -25.25560589046783733, -4.310829775027113620, 167.9999999999999716 ) ) ;
#165945=ORIENTED_EDGE ( 'NONE', *, *, #42863, .F. ) ;
#165965=CARTESIAN_POINT ( 'NONE',  ( -17.14385361876520619, 23.59649016807275856, 146.5750000027311444 ) ) ;
#165968=EDGE_LOOP ( 'NONE', ( #59129, #31212 ) ) ;
#166026=DIRECTION ( 'NONE',  ( 0.000000000000000000, -0.9945218953682734009, 0.1045284632676537068 ) ) ;
#166049=CARTESIAN_POINT ( 'NONE',  ( -25.82893184620927229, 8.167111171438236283, 172.3011985515803417 ) ) ;
#166105=CARTESIAN_POINT ( 'NONE',  ( -28.82186960331499392, 9.364793116373565596, 147.8999999999999488 ) ) ;
#166121=CARTESIAN_POINT ( 'NONE',  ( 24.06609220500530100, -14.38661408136896114, 165.8682408874383896 ) ) ;
#166259=CARTESIAN_POINT ( 'NONE',  ( 27.73933785331498569, 9.013057229001093518, 147.9750000027311501 ) ) ;
#166266=( GEOMETRIC_REPRESENTATION_CONTEXT ( 3 ) GLOBAL_UNCERTAINTY_ASSIGNED_CONTEXT ( ( #51963 ) ) GLOBAL_UNIT_ASSIGNED_CONTEXT ( ( #93038, #1025, #174872 ) ) REPRESENTATION_CONTEXT ( 'NONE', 'WORKASPACE' ) );
#166456=CARTESIAN_POINT ( 'NONE',  ( 22.44159573604009239, 16.30477369853692693, 142.5750000027311728 ) ) ;
#166496=CARTESIAN_POINT ( 'NONE',  ( -24.86475712555574802, -11.37215039200969890, 169.9824823118008226 ) ) ;
#166648=( BOUNDED_SURFACE ( )  B_SPLINE_SURFACE ( 3, 2, ( 
 ( #20971, #170925, #113963 ),
 ( #52306, #108252, #125421 ),
 ( #31423, #93076, #175662 ),
 ( #37136, #98796, #109245 ),
 ( #16258, #139576, #1061 ),
 ( #186111, #84628, #180679 ),
 ( #69478, #103815, #114982 ),
 ( #85638, #57320, #178669 ),
 ( #38151, #71479, #192832 ),
 ( #133144, #118996, #134159 ),
 ( #21980, #194835, #193841 ),
 ( #55305, #130126, #54313 ),
 ( #56308, #195847, #42155 ),
 ( #83632, #24996, #22979 ),
 ( #116977, #25993, #40132 ),
 ( #10816, #191823, #117990 ),
 ( #86640, #162480, #99805 ),
 ( #146306, #161491, #9818 ),
 ( #149322, #179680, #72486 ),
 ( #100797, #101810, #163498 ),
 ( #39142, #145309, #6792 ),
 ( #148323, #41152, #23982 ),
 ( #102815, #164500, #68471 ),
 ( #115985, #87636, #53303 ) ),
 .UNSPECIFIED., .F., .F., .T. ) 
 B_SPLINE_SURFACE_WITH_KNOTS ( ( 4, 2, 2, 2, 2, 2, 2, 2, 2, 2, 2, 4 ),
 ( 3, 3 ),
 ( -1.040834085586084257E-17, 0.001899702839891682536, 0.002849554259837528900, 0.003799405679783375480, 0.005699108519675068207, 0.006648959939620915222, 0.007598811359566761368, 0.008548662779512607515, 0.009498514199458454529, 0.01139821703935014682, 0.01329791987924184085, 0.01519762271913353315 ),
 ( 0.000000000000000000, 1.000000000000000000 ),
 .UNSPECIFIED. ) 
 GEOMETRIC_REPRESENTATION_ITEM ( )  RATIONAL_B_SPLINE_SURFACE ( (
 ( 1.000000000000000000, 0.7660444431189795678, 1.000000000000000000),
 ( 1.000000000000000000, 0.7753720600381870387, 1.000000000000000000),
 ( 1.000000000000000000, 0.7832595754286640899, 1.000000000000000000),
 ( 1.000000000000000000, 0.7928595458705136600, 1.000000000000000000),
 ( 1.000000000000000000, 0.7956872332516109481, 1.000000000000000000),
 ( 1.000000000000000000, 0.8005750596157605870, 1.000000000000000000),
 ( 1.000000000000000000, 0.8026302056541708696, 1.000000000000000000),
 ( 1.000000000000000000, 0.8075080643848453477, 1.000000000000000000),
 ( 1.000000000000000000, 0.8091143015810815520, 1.000000000000000000),
 ( 1.000000000000000000, 0.8093067629632570981, 1.000000000000000000),
 ( 1.000000000000000000, 0.8089952915731098981, 1.000000000000000000),
 ( 1.000000000000000000, 0.8076919994862900021, 1.000000000000000000),
 ( 1.000000000000000000, 0.8067078407648371474, 1.000000000000000000),
 ( 1.000000000000000000, 0.8041786842467988361, 1.000000000000000000),
 ( 1.000000000000000000, 0.8026334674876747233, 1.000000000000000000),
 ( 1.000000000000000000, 0.7990747329469696236, 1.000000000000000000),
 ( 1.000000000000000000, 0.7970509760941616451, 1.000000000000000000),
 ( 1.000000000000000000, 0.7904793850863758298, 1.000000000000000000),
 ( 1.000000000000000000, 0.7855040224314863151, 1.000000000000000000),
 ( 1.000000000000000000, 0.7751942650506468135, 1.000000000000000000),
 ( 1.000000000000000000, 0.7698260778211376554, 1.000000000000000000),
 ( 1.000000000000000000, 0.7598259884961129362, 1.000000000000000000),
 ( 1.000000000000000000, 0.7551428682220174826, 1.000000000000000000),
 ( 1.000000000000000000, 0.7510191126010865581, 1.000000000000000000) ) ) 
 REPRESENTATION_ITEM ( '' )  SURFACE ( )  );
#166659=CARTESIAN_POINT ( 'NONE',  ( -22.94331271462294808, -3.784814030245898575, 190.0000000000000000 ) ) ;
#166686=DIRECTION ( 'NONE',  ( -1.000000000000000000, 0.000000000000000000, 0.000000000000000000 ) ) ;
#166693=CARTESIAN_POINT ( 'NONE',  ( -21.76075944043963872, -9.615265036675765487, 170.8440536485302061 ) ) ;
#166733=CARTESIAN_POINT ( 'NONE',  ( -21.98685479826780309, 13.98560643873834231, 165.5209445330007725 ) ) ;
#166765=VECTOR ( 'NONE', #178341, 1000.000000000000114 ) ;
#166800=CARTESIAN_POINT ( 'NONE',  ( 22.44159573604009594, -16.30477369853687364, 143.6750000027311671 ) ) ;
#166843=FACE_OUTER_BOUND ( 'NONE', #12053, .T. ) ;
#166900=CARTESIAN_POINT ( 'NONE',  ( 19.49401214000073779, -12.39993551617566503, 164.9999999999999716 ) ) ;
#166960=CARTESIAN_POINT ( 'NONE',  ( -17.14385361876520619, 23.59649016807275856, 144.5750000027312012 ) ) ;
#166972=CARTESIAN_POINT ( 'NONE',  ( 27.73933785331498925, -9.013057229001034898, 140.2750000027311614 ) ) ;
#166990=VECTOR ( 'NONE', #122568, 1000.000000000000000 ) ;
#166996=CARTESIAN_POINT ( 'NONE',  ( -27.91311885011354121, 2.086775749827418075E-14, 155.0000000000000000 ) ) ;
#167038=CARTESIAN_POINT ( 'NONE',  ( -18.94301819075103310, -21.11311916587052906, 139.9999999999999716 ) ) ;
#167080=ORIENTED_EDGE ( 'NONE', *, *, #27827, .F. ) ;
#167094=CARTESIAN_POINT ( 'NONE',  ( 8.906447517083057264, -27.41122689804191026, 144.5999999999999943 ) ) ;
#167119=CARTESIAN_POINT ( 'NONE',  ( -24.04960827311053606, 5.809912860844014482, 170.7323280178997891 ) ) ;
#167197=CARTESIAN_POINT ( 'NONE',  ( -21.94905633995418270, -7.481063542987935300, 170.0146117665048848 ) ) ;
#167237=CARTESIAN_POINT ( 'NONE',  ( -3.573655867282028392E-15, 2.428612866367529932E-14, 169.9999999999999716 ) ) ;
#167369=EDGE_CURVE ( 'NONE', #101974, #67859, #191206, .T. ) ;
#167387=CARTESIAN_POINT ( 'NONE',  ( 20.48541513753860954, -11.15937153969631979, 168.1083253156164119 ) ) ;
#167440=CARTESIAN_POINT ( 'NONE',  ( 27.73933785331498569, 2.768321779492822058E-14, 144.3750000027311842 ) ) ;
#167444=CARTESIAN_POINT ( 'NONE',  ( 27.73933785331498925, -9.013057229001033122, 144.2750000027311899 ) ) ;
#167449=DIRECTION ( 'NONE',  ( 1.000000000000000000, 0.000000000000000000, 0.000000000000000000 ) ) ;
#167481=CARTESIAN_POINT ( 'NONE',  ( -21.81230582904511550, -7.807068725607987147, 172.9985625539908085 ) ) ;
#167692=CARTESIAN_POINT ( 'NONE',  ( 28.79475375365573697, 9.355982642739409272, 145.0843446569000434 ) ) ;
#167756=CARTESIAN_POINT ( 'NONE',  ( -17.79613651744293890, -24.49428055684527550, 142.2843446568999752 ) ) ;
#167780=CARTESIAN_POINT ( 'NONE',  ( -8.571926809382601320, -26.38167802310801591, 147.2750000027311899 ) ) ;
#167836=CARTESIAN_POINT ( 'NONE',  ( 25.22510128165246002, 6.326562104755751648, 165.8168824682948070 ) ) ;
#167855=CARTESIAN_POINT ( 'NONE',  ( 28.79475375365660028, 9.355982642738212007, 143.0843446568999582 ) ) ;
#167934=PRODUCT_DEFINITION_SHAPE ( 'NONE', 'NONE',  #183372 ) ;
#167938=DIRECTION ( 'NONE',  ( 0.000000000000000000, 0.000000000000000000, 1.000000000000000000 ) ) ;
#167939=CARTESIAN_POINT ( 'NONE',  ( 27.73933785331498569, 2.768321779492822058E-14, 145.8750000027311842 ) ) ;
#167988=CARTESIAN_POINT ( 'NONE',  ( -22.96528548301343520, 5.795830589372932273, 190.0000000000000000 ) ) ;
#168020=CARTESIAN_POINT ( 'NONE',  ( -11.30073351558003480, -25.82347143560497926, 139.9999999999999716 ) ) ;
#168231=DIRECTION ( 'NONE',  ( 0.000000000000000000, 0.000000000000000000, -1.000000000000000000 ) ) ;
#168348=ORIENTED_EDGE ( 'NONE', *, *, #58299, .F. ) ;
#168410=EDGE_CURVE ( 'NONE', #193436, #162084, #118500, .T. ) ;
#168418=CARTESIAN_POINT ( 'NONE',  ( 1.784210473542230573E-15, -29.16686587814331588, 141.8750000027311842 ) ) ;
#168422=CARTESIAN_POINT ( 'NONE',  ( 17.14385361876520264, -23.59649016807271238, 146.0750000027311728 ) ) ;
#168458=CARTESIAN_POINT ( 'NONE',  ( -21.88033147701211689, -9.239123595180315007, 171.1226046679803403 ) ) ;
#168752=CARTESIAN_POINT ( 'NONE',  ( -22.44159573604009950, -16.30477369853688430, 143.0750000027311728 ) ) ;
#168823=ORIENTED_EDGE ( 'NONE', *, *, #70540, .F. ) ;
#168828=CARTESIAN_POINT ( 'NONE',  ( -28.79475375365586842, 2.428612866367529932E-14, 143.9843446568999923 ) ) ;
#168836=DIRECTION ( 'NONE',  ( -0.000000000000000000, -0.000000000000000000, -1.000000000000000000 ) ) ;
#168887=EDGE_LOOP ( 'NONE', ( #99658, #176176, #83992, #63156 ) ) ;
#168891=CARTESIAN_POINT ( 'NONE',  ( 29.15849868437704728, -10.00000000000000000, 150.0000000000000000 ) ) ;
#168914=CARTESIAN_POINT ( 'NONE',  ( -27.73933785331498925, 9.013057229001089965, 142.7750000027311899 ) ) ;
#168994=CARTESIAN_POINT ( 'NONE',  ( -19.78400068765821374, -20.35809916000442499, 140.0000000000000000 ) ) ;
#169154=CARTESIAN_POINT ( 'NONE',  ( -24.40828949532285463, -2.848420800298675282, 173.9378174459543516 ) ) ;
#169191=CARTESIAN_POINT ( 'NONE',  ( -26.45564479744090036, -7.620358626195407936, 168.5728521449592279 ) ) ;
#169344=CARTESIAN_POINT ( 'NONE',  ( 20.09035150276018555, -11.70762861043687053, 168.0245124264526453 ) ) ;
#169404=CARTESIAN_POINT ( 'NONE',  ( -27.73933785331498925, -9.013057229001049109, 145.4750000027311501 ) ) ;
#169408=CARTESIAN_POINT ( 'NONE',  ( 8.571926809382597767, 26.38167802310806209, 146.7750000027311899 ) ) ;
#169410=LINE ( 'NONE', #2548, #98019 ) ;
#169447=CARTESIAN_POINT ( 'NONE',  ( -21.75836449082842705, -9.620754668594841519, 170.8405250346321509 ) ) ;
#169603=CARTESIAN_POINT ( 'NONE',  ( 14.78475781823265756, 23.88375075827561034, 139.9999999999999716 ) ) ;
#169694=CARTESIAN_POINT ( 'NONE',  ( -19.83802472612592993, 12.02135855755751059, 167.9999999999999716 ) ) ;
#169758=CARTESIAN_POINT ( 'NONE',  ( 27.73933785331498925, -9.013057229001033122, 143.7750000027311614 ) ) ;
#169847=CARTESIAN_POINT ( 'NONE',  ( -3.573655867282028392E-15, 2.428612866367529932E-14, 169.9999999999999716 ) ) ;
#169923=CARTESIAN_POINT ( 'NONE',  ( -27.73933785331498925, 9.013057229001089965, 146.7750000027312183 ) ) ;
#170063=CARTESIAN_POINT ( 'NONE',  ( -23.31738231874055600, 16.94106989632528837, 141.7999999999999829 ) ) ;
#170075=CARTESIAN_POINT ( 'NONE',  ( 25.62062145120188816, -9.171473787276744005, 171.1688781158082691 ) ) ;
#170091=CARTESIAN_POINT ( 'NONE',  ( 0.000000000000000000, 5.795830589372932273, 190.0000000000000000 ) ) ;
#170103=ORIENTED_EDGE ( 'NONE', *, *, #167369, .F. ) ;
#170111=CARTESIAN_POINT ( 'NONE',  ( -3.573655867282028392E-15, 12.39993551617566681, 175.0000000000000000 ) ) ;
#170129=ADVANCED_FACE ( 'NONE', ( #162040 ), #101352, .T. ) ;
#170158=CARTESIAN_POINT ( 'NONE',  ( -21.47377332592085963, -5.474134792251713399, 173.8918256800992594 ) ) ;
#170162=AXIS2_PLACEMENT_3D ( 'NONE', #174775, #95933, #126275 ) ;
#170283=EDGE_LOOP ( 'NONE', ( #148780, #126801, #164395, #194463 ) ) ;
#170318=COLOUR_RGB ( '', 0.72549020, 0.75294118, 0.79215686) ;
#170322=CARTESIAN_POINT ( 'NONE',  ( -3.573655867282028392E-15, 2.428612866367529932E-14, 167.9999999999999716 ) ) ;
#170325=CARTESIAN_POINT ( 'NONE',  ( 27.56318840656206248, 3.609252070617571473, 139.9999999999999716 ) ) ;
#170350=CARTESIAN_POINT ( 'NONE',  ( 21.93187539022923715, -6.436421874423670531, 171.3066408880984852 ) ) ;
#170361=DIRECTION ( 'NONE',  ( 0.000000000000000000, 0.000000000000000000, 1.000000000000000000 ) ) ;
#170412=CARTESIAN_POINT ( 'NONE',  ( -27.73933785331498925, 9.013057229001089965, 145.2750000027311899 ) ) ;
#170694=CARTESIAN_POINT ( 'NONE',  ( -22.37486833544148368, 13.37560805684316101, 165.5209445320982695 ) ) ;
#170738=( BOUNDED_CURVE ( )  B_SPLINE_CURVE ( 2, ( #5700, #40037, #101710, #176577, #38051, #163401, #52210, #175564, #192736, #83533, #67377 ),
 .UNSPECIFIED., .F., .T. ) 
 B_SPLINE_CURVE_WITH_KNOTS ( ( 3, 2, 2, 2, 2, 3 ),
 ( 0.7000000000000006217, 0.7200000000000006395, 0.7400000000000006573, 0.7600000000000006750, 0.7800000000000006928, 0.8000000000000007105 ),
 .UNSPECIFIED. ) 
 CURVE ( )  GEOMETRIC_REPRESENTATION_ITEM ( )  RATIONAL_B_SPLINE_CURVE ( ( 0.9999999999999983347, 0.9510565162951551965, 1.000000000000000000, 0.9510565162951535312, 1.000000000000000000, 0.9510565162951535312, 1.000000000000000000, 0.9510565162951535312, 1.000000000000000000, 0.9510565162951518658, 1.000000000000001554 ) ) 
 REPRESENTATION_ITEM ( '' )  );
#170758=CARTESIAN_POINT ( 'NONE',  ( -17.14385361876520619, 23.59649016807275856, 148.5750000027311444 ) ) ;
#170795=CARTESIAN_POINT ( 'NONE',  ( -27.60098488412539908, -5.861468761075184553, 164.8187539380755311 ) ) ;
#170917=CARTESIAN_POINT ( 'NONE',  ( 8.571926809382597767, 26.38167802310806209, 140.2750000027311899 ) ) ;
#170925=CARTESIAN_POINT ( 'NONE',  ( 21.61802400803982849, -13.75099706318440873, 167.9999999999999432 ) ) ;
#170953=CARTESIAN_POINT ( 'NONE',  ( 23.29544513554940366, -16.92513159979222337, 140.7843446568999752 ) ) ;
#171007=EDGE_CURVE ( 'NONE', #9294, #33383, #185847, .T. ) ;
#171048=CARTESIAN_POINT ( 'NONE',  ( -24.93942350307309752, -7.769968609432603479, 171.2173313942149662 ) ) ;
#171057=CARTESIAN_POINT ( 'NONE',  ( 28.82186960331499392, -9.364793116373510529, 140.9000000000000057 ) ) ;
#171070=CARTESIAN_POINT ( 'NONE',  ( 25.70602947687970641, -7.354137148287276382, 175.2376750527030254 ) ) ;
#171107=EDGE_CURVE ( 'NONE', #61621, #48040, #89266, .T. ) ;
#171156=CARTESIAN_POINT ( 'NONE',  ( -24.27957997113618305, -6.290849861786781183, 171.5443985711290793 ) ) ;
#171324=CARTESIAN_POINT ( 'NONE',  ( 20.91330281277714676, -18.31365339088606348, 140.0000000000000568 ) ) ;
#171404=ORIENTED_EDGE ( 'NONE', *, *, #136656, .F. ) ;
#171523=EDGE_CURVE ( 'NONE', #35595, #112207, #165122, .T. ) ;
#171600=CARTESIAN_POINT ( 'NONE',  ( 2.107141108080088809, 28.27445460515380304, 140.0000000000000284 ) ) ;
#171663=CARTESIAN_POINT ( 'NONE',  ( -17.79613651744294600, 24.49428055684532524, 145.6843446568999809 ) ) ;
#171689=CARTESIAN_POINT ( 'NONE',  ( -21.95653654802609722, 6.613221094984321979, 171.0358100525039902 ) ) ;
#171751=CARTESIAN_POINT ( 'NONE',  ( 21.57728377622143512, 10.02787190051641453, 170.5958156194642186 ) ) ;
#171756=CARTESIAN_POINT ( 'NONE',  ( -8.571926809382608425, 26.38167802310805854, 140.4750000027312069 ) ) ;
#171837=DIRECTION ( 'NONE',  ( 0.000000000000000000, 0.000000000000000000, 1.000000000000000000 ) ) ;
#171841=CARTESIAN_POINT ( 'NONE',  ( -24.84792715949104291, -12.91290060751520130, 166.0205615092969822 ) ) ;
#171965=ADVANCED_FACE ( 'NONE', ( #13418 ), #121718, .T. ) ;
#171982=CARTESIAN_POINT ( 'NONE',  ( 24.57691432906749540, 7.727872488968289488, 167.2019946024467743 ) ) ;
#172042=CARTESIAN_POINT ( 'NONE',  ( -26.53317239408749373, 7.611579847057692305, 168.2742808015845526 ) ) ;
#172065=CARTESIAN_POINT ( 'NONE',  ( 21.70479006154364043, -9.754118203517492702, 170.7545476126473147 ) ) ;
#172071=CARTESIAN_POINT ( 'NONE',  ( 21.38418241377623019, -7.427326039334300134, 174.4773576836617224 ) ) ;
#172144=EDGE_CURVE ( 'NONE', #93307, #122542, #118714, .T. ) ;
#172146=CARTESIAN_POINT ( 'NONE',  ( -28.82186960331499392, -9.364793116373526516, 144.3500000054623627 ) ) ;
#172161=CARTESIAN_POINT ( 'NONE',  ( -5.359611314223446995E-15, 29.16686587814335851, 148.8750000027311842 ) ) ;
#172204=PLANE ( 'NONE',  #18510 ) ;
#172268=ORIENTED_EDGE ( 'NONE', *, *, #17592, .F. ) ;
#172271=ORIENTED_EDGE ( 'NONE', *, *, #162246, .F. ) ;
#172273=ORIENTED_EDGE ( 'NONE', *, *, #88289, .T. ) ;
#172330=ORIENTED_EDGE ( 'NONE', *, *, #76057, .T. ) ;
#172435=B_SPLINE_CURVE_WITH_KNOTS ( 'NONE', 3,
 ( #190107, #95098, #50601, #145582, #52575, #98054, #83899, #33439, #66750, #128411, #172954, #189129, #188128, #111263 ),
 .UNSPECIFIED., .F., .F.,
 ( 4, 2, 2, 2, 2, 2, 4 ),
 ( 0.000000000000000000, 0.05072380597786523698, 0.1014476119557304740, 0.2028952239114615863, 0.4057904478229238943, 0.6086856717343860357, 0.8115808956458483436 ),
 .UNSPECIFIED. ) ;
#172455=CARTESIAN_POINT ( 'NONE',  ( 28.79475375365586132, 2.781246896534039337E-14, 141.2656553485623760 ) ) ;
#172649=ORIENTED_EDGE ( 'NONE', *, *, #19336, .T. ) ;
#172658=VERTEX_POINT ( 'NONE', #136110 ) ;
#172668=ADVANCED_FACE ( 'NONE', ( #72450 ), #41115, .F. ) ;
#172684=CARTESIAN_POINT ( 'NONE',  ( -24.06756124613724168, 8.142616467497040489, 169.4332804344609542 ) ) ;
#172730=CARTESIAN_POINT ( 'NONE',  ( 0.000000000000000000, 0.000000000000000000, 190.0000000000000000 ) ) ;
#172735=AXIS2_PLACEMENT_3D ( 'NONE', #162124, #98427, #82258 ) ;
#172753=CARTESIAN_POINT ( 'NONE',  ( 27.73933785331498569, 2.768321779492822058E-14, 139.8750000027311842 ) ) ;
#172791=CARTESIAN_POINT ( 'NONE',  ( 23.88378066561468316, 7.642901331109205998, 172.4262957903898723 ) ) ;
#172920=CARTESIAN_POINT ( 'NONE',  ( 27.73933785331498214, 9.013057229001095294, 139.9750000027311501 ) ) ;
#172954=CARTESIAN_POINT ( 'NONE',  ( 24.27707668318813816, -5.858708095980206920, 170.2635530474734367 ) ) ;
#172965=CARTESIAN_POINT ( 'NONE',  ( -24.95432927374998044, 3.806786798636383917, 190.0000000000000000 ) ) ;
#172984=CARTESIAN_POINT ( 'NONE',  ( 21.75836449082842705, 8.509082329563685931, 169.1767350484841472 ) ) ;
#173068=CARTESIAN_POINT ( 'NONE',  ( 25.52568752982154265, -9.519068727184667011, 170.8917780290425412 ) ) ;
#173074=CARTESIAN_POINT ( 'NONE',  ( 21.59135963187072349, -7.527667041516026281, 173.8290201207856285 ) ) ;
#173089=AXIS2_PLACEMENT_3D ( 'NONE', #104984, #45306, #13959 ) ;
#173096=EDGE_CURVE ( 'NONE', #25364, #11205, #24984, .T. ) ;
#173115=( BOUNDED_CURVE ( )  B_SPLINE_CURVE ( 2, ( #181432, #87411, #57087, #86409, #133925, #116746, #25765, #195615, #196608, #166259, #89401, #103588, #151090, #11594, #24762, #10586, #165263, #193604, #27758, #39904, #118761, #163260, #197586, #88397, #41922, #26757, #12581, #73262, #74246, #135915, #55076, #102586, #56074, #71251, #148094, #9585, #132915, #194602, #117755, #72247, #179447, #40913, #164270, #143727, #144722, #37552, #194256, #190245, #84046, #68890, #116394, #115404, #21389, #99215, #36541, #159901, #193248, #147746, #83048, #66887, #9233, #20383, #160903, #24408, #82030, #161901, #70900, #177092, #51722, #38564, #85042, #132567, #55723, #7206, #114379, #100220, #158893, #175075, #6208, #174090, #69896, #35559, #97207, #67888, #176083, #129541, #54721, #8220, #5206, #191241, #146723 ),
 .UNSPECIFIED., .F., .F. ) 
 B_SPLINE_CURVE_WITH_KNOTS ( ( 3, 2, 2, 2, 2, 2, 2, 2, 2, 2, 2, 2, 2, 2, 2, 2, 2, 2, 2, 2, 2, 2, 2, 2, 2, 2, 2, 2, 2, 2, 2, 2, 2, 2, 2, 2, 2, 2, 2, 2, 2, 2, 2, 2, 2, 3 ),
 ( 0.000000000000000000, 0.02000000000000000042, 0.04000000000000000083, 0.06000000000000000472, 0.08000000000000000167, 0.1000000000000000056, 0.1200000000000000094, 0.1400000000000000133, 0.1600000000000000033, 0.1799999999999999933, 0.2000000000000000111, 0.2200000000000000011, 0.2400000000000000189, 0.2600000000000000089, 0.2800000000000000266, 0.2999999999999999889, 0.3200000000000000067, 0.3400000000000000244, 0.3599999999999999867, 0.3800000000000000044, 0.4000000000000000222, 0.4199999999999999845, 0.4400000000000000022, 0.4600000000000000200, 0.4800000000000000377, 0.5000000000000000000, 0.5200000000000000178, 0.5400000000000000355, 0.5600000000000000533, 0.5799999999999999600, 0.5999999999999999778, 0.6199999999999999956, 0.6400000000000000133, 0.6600000000000000311, 0.6800000000000000488, 0.6999999999999999556, 0.7199999999999999734, 0.7399999999999999911, 0.7600000000000000089, 0.7800000000000000266, 0.8000000000000000444, 0.8199999999999999512, 0.8399999999999999689, 0.8599999999999999867, 0.8800000000000000044, 0.8875575298689686310 ),
 .UNSPECIFIED. ) 
 CURVE ( )  GEOMETRIC_REPRESENTATION_ITEM ( )  RATIONAL_B_SPLINE_CURVE ( ( 1.000000000000000000, 0.9510565162951535312, 1.000000000000000000, 0.9510565162951535312, 1.000000000000000000, 0.9510565162951535312, 1.000000000000000000, 0.9510565162951535312, 1.000000000000000000, 0.9510565162951535312, 1.000000000000000000, 0.9510565162951535312, 1.000000000000000000, 0.9510565162951535312, 1.000000000000000000, 0.9510565162951535312, 1.000000000000000000, 0.9510565162951535312, 1.000000000000000000, 0.9510565162951535312, 1.000000000000000000, 0.9510565162951535312, 1.000000000000000000, 0.9510565162951535312, 1.000000000000000000, 0.9510565162951535312, 1.000000000000000000, 0.9510565162951535312, 1.000000000000000000, 0.9510565162951535312, 1.000000000000000000, 0.9510565162951535312, 1.000000000000000000, 0.9510565162951535312, 1.000000000000000000, 0.9510565162951535312, 1.000000000000000000, 0.9510565162951535312, 1.000000000000000000, 0.9510565162951535312, 1.000000000000000000, 0.9510565162951535312, 1.000000000000000000, 0.9510565162951535312, 1.000000000000000000, 0.9510565162951535312, 1.000000000000000000, 0.9510565162951535312, 1.000000000000000000, 0.9510565162951535312, 1.000000000000000000, 0.9510565162951535312, 1.000000000000000000, 0.9510565162951535312, 1.000000000000000000, 0.9510565162951535312, 1.000000000000000000, 0.9510565162951535312, 1.000000000000000000, 0.9510565162951535312, 1.000000000000000000, 0.9510565162951535312, 1.000000000000000000, 0.9510565162951535312, 1.000000000000000000, 0.9510565162951535312, 1.000000000000000000, 0.9510565162951535312, 1.000000000000000000, 0.9510565162951535312, 1.000000000000000000, 0.9510565162951535312, 1.000000000000000000, 0.9510565162951535312, 1.000000000000000000, 0.9510565162951535312, 1.000000000000000000, 0.9510565162951535312, 1.000000000000000000, 0.9510565162951535312, 1.000000000000000000, 0.9510565162951535312, 1.000000000000000000, 0.9510565162951535312, 1.000000000000000000, 0.9510565162951535312, 1.000000000000000000, 0.9510565162951535312, 1.000000000000000000, 0.9815054080004621540, 0.9769881591460138903 ) ) 
 REPRESENTATION_ITEM ( '' )  );
#173149=CARTESIAN_POINT ( 'NONE',  ( -17.81289503416611808, 24.51734667627700404, 145.9500000054623854 ) ) ;
#173181=AXIS2_PLACEMENT_3D ( 'NONE', #74025, #195384, #162027 ) ;
#173275=ORIENTED_EDGE ( 'NONE', *, *, #68275, .F. ) ;
#173337=ORIENTED_EDGE ( 'NONE', *, *, #77698, .F. ) ;
#173440=CARTESIAN_POINT ( 'NONE',  ( -3.573655867282028392E-15, 2.428612866367529932E-14, 155.0000000000000000 ) ) ;
#173526=AXIS2_PLACEMENT_3D ( 'NONE', #189965, #82755, #144435 ) ;
#173536=ORIENTED_EDGE ( 'NONE', *, *, #101580, .T. ) ;
#173632=EDGE_LOOP ( 'NONE', ( #94804, #143761, #156538, #67922, #126148 ) ) ;
#173635=DIRECTION ( 'NONE',  ( 0.000000000000000000, 0.000000000000000000, 1.000000000000000000 ) ) ;
#173652=ADVANCED_FACE ( 'NONE', ( #183611 ), #147647, .T. ) ;
#173664=ORIENTED_EDGE ( 'NONE', *, *, #24864, .T. ) ;
#173689=CARTESIAN_POINT ( 'NONE',  ( -21.35462415990441087, 9.648971641164905577, 168.5494316893069140 ) ) ;
#173749=CARTESIAN_POINT ( 'NONE',  ( 20.51359854606069177, 11.49117151696134442, 170.0775129446642495 ) ) ;
#173754=CARTESIAN_POINT ( 'NONE',  ( 17.14385361876520264, 23.59649016807275856, 140.1750000027311955 ) ) ;
#173767=TOROIDAL_SURFACE ( 'NONE', #70422, 23.10356920737165254, 3.000000000000000000 ) ;
#173829=CARTESIAN_POINT ( 'NONE',  ( 27.05641397906351386, -3.631740835637518927, 169.9999999999999716 ) ) ;
#173841=VERTEX_POINT ( 'NONE', #124908 ) ;
#173876=DIRECTION ( 'NONE',  ( 0.9945218953682734009, 0.000000000000000000, 0.1045284632676537068 ) ) ;
#173885=B_SPLINE_CURVE_WITH_KNOTS ( 'NONE', 3,
 ( #138737, #218, #110389, #49721, #93223, #156906, #1210, #62888, #111388, #46745, #4193, #3212, #124568, #47743, #77066, #173074, #155900, #172071 ),
 .UNSPECIFIED., .F., .F.,
 ( 4, 2, 2, 2, 2, 2, 2, 2, 4 ),
 ( 0.000000000000000000, 0.001023866006848666178, 0.002047732013697332355, 0.003071598020545998533, 0.004095464027394664711, 0.005119330034243330455, 0.006143196041091997066, 0.007167062047940663677, 0.008190928054789329421 ),
 .UNSPECIFIED. ) ;
#173931=TOROIDAL_SURFACE ( 'NONE', #161616, 23.10356920737165254, 5.000000000000000000 ) ;
#174067=CARTESIAN_POINT ( 'NONE',  ( 20.56371838171487809, -11.43208494587337043, 170.0924998638764976 ) ) ;
#174090=CARTESIAN_POINT ( 'NONE',  ( -27.73933785331498925, -9.013057229001049109, 140.9750000027311785 ) ) ;
#174143=CARTESIAN_POINT ( 'NONE',  ( -5.359611314223446995E-15, 29.16686587814335496, 144.8750000027311557 ) ) ;
#174144=CARTESIAN_POINT ( 'NONE',  ( 28.82186960331498327, 2.781578969918950771E-14, 145.2500000054623683 ) ) ;
#174207=CARTESIAN_POINT ( 'NONE',  ( 28.79475375365588619, 9.355982642739197885, 147.3656553485623704 ) ) ;
#174329=ORIENTED_EDGE ( 'NONE', *, *, #152669, .T. ) ;
#174388=EDGE_LOOP ( 'NONE', ( #133075, #68495, #162845, #111019 ) ) ;
#174448=CARTESIAN_POINT ( 'NONE',  ( -19.49401214000077331, 12.39993551617566681, 169.9999999999999716 ) ) ;
#174634=FACE_OUTER_BOUND ( 'NONE', #63403, .T. ) ;
#174642=ORIENTED_EDGE ( 'NONE', *, *, #99297, .F. ) ;
#174735=CARTESIAN_POINT ( 'NONE',  ( 21.91636330721480874, 8.102911641865347292, 172.4379571683062409 ) ) ;
#174752=CARTESIAN_POINT ( 'NONE',  ( 26.58496454516998142, -7.626754437231455519, 167.9682100371138915 ) ) ;
#174775=CARTESIAN_POINT ( 'NONE',  ( -26.97479053218977896, 7.816291847812730786, 151.6430507545553894 ) ) ;
#174872=( NAMED_UNIT ( * ) SI_UNIT ( $, .STERADIAN. ) SOLID_ANGLE_UNIT ( ) );
#174941=B_SPLINE_CURVE_WITH_KNOTS ( 'NONE', 3,
 ( #132901, #194590, #27745, #43885, #56060, #8565, #70240, #131908, #39888, #42897, #180437, #104562, #117739, #89388, #101555, #12567, #165250, #164257, #163247, #118748 ),
 .UNSPECIFIED., .F., .F.,
 ( 4, 2, 2, 2, 2, 2, 2, 2, 2, 4 ),
 ( 0.000000000000000000, 0.001368201656092175042, 0.002736403312184350085, 0.004104604968276525344, 0.005472806624368700169, 0.006841008280460872393, 0.008209209936553043749, 0.008893310764599119886, 0.009577411592645196023, 0.01094561324873732922 ),
 .UNSPECIFIED. ) ;
#174967=CARTESIAN_POINT ( 'NONE',  ( 23.34492853952160374, 11.48509598731698667, 165.7658222004386062 ) ) ;
#175002=EDGE_CURVE ( 'NONE', #101974, #15498, #137091, .T. ) ;
#175018=EDGE_CURVE ( 'NONE', #2773, #63582, #115808, .T. ) ;
#175032=CARTESIAN_POINT ( 'NONE',  ( -22.67087683854552793, -7.530304285672279718, 173.4975851171454053 ) ) ;
#175058=DIRECTION ( 'NONE',  ( -0.1736481776669307198, -2.126576849575776229E-17, -0.9848077530122080203 ) ) ;
#175063=CARTESIAN_POINT ( 'NONE',  ( 24.69864643647408187, -7.736333414721475954, 171.5373488951853176 ) ) ;
#175067=CARTESIAN_POINT ( 'NONE',  ( -26.58496454517000629, 7.626754437231443084, 167.9682100371138915 ) ) ;
#175075=CARTESIAN_POINT ( 'NONE',  ( -17.14385361876520264, -23.59649016807271238, 141.1750000027311671 ) ) ;
#175080=EDGE_LOOP ( 'NONE', ( #195259, #26181, #161173, #76153, #105023, #49743 ) ) ;
#175131=CARTESIAN_POINT ( 'NONE',  ( -17.81289503416611097, -24.51734667627696496, 146.5500000054623229 ) ) ;
#175144=CARTESIAN_POINT ( 'NONE',  ( 8.571926809382603096, -26.38167802310801235, 147.9750000027311785 ) ) ;
#175304=CARTESIAN_POINT ( 'NONE',  ( 28.79475375365586132, 2.781246896534039337E-14, 145.2656553485623760 ) ) ;
#175356=CARTESIAN_POINT ( 'NONE',  ( -23.64874990377915509, 15.04272038711346049, 165.8682408883346397 ) ) ;
#175387=VECTOR ( 'NONE', #60183, 1000.000000000000114 ) ;
#175528=EDGE_CURVE ( 'NONE', #144964, #199519, #54252, .T. ) ;
#175564=CARTESIAN_POINT ( 'NONE',  ( -17.79613651744294600, 24.49428055684532524, 147.6843446569000093 ) ) ;
#175575=CARTESIAN_POINT ( 'NONE',  ( -3.573655867282028392E-15, -12.39993551617566503, 169.9999999999999716 ) ) ;
#175605=EDGE_CURVE ( 'NONE', #34941, #193436, #7265, .T. ) ;
#175613=CARTESIAN_POINT ( 'NONE',  ( 26.45564479744089326, 7.620358626195402607, 168.5728521449592847 ) ) ;
#175625=CARTESIAN_POINT ( 'NONE',  ( -22.78714015945949356, -11.73760554535633105, 167.9671921004704416 ) ) ;
#175662=CARTESIAN_POINT ( 'NONE',  ( 20.14845677604719043, -11.63499142542172571, 168.0304984204096286 ) ) ;
#175746=ORIENTED_EDGE ( 'NONE', *, *, #36547, .F. ) ;
#175768=CARTESIAN_POINT ( 'NONE',  ( 22.19348515620995954, 7.491027558428855038, 173.8712782147084965 ) ) ;
#175973=CARTESIAN_POINT ( 'NONE',  ( 23.91168844458708875, 8.792376985860574479, 168.9858545422794691 ) ) ;
#176079=CARTESIAN_POINT ( 'NONE',  ( -24.45434260692611517, -5.907237110200219021, 169.8064932912610914 ) ) ;
#176083=CARTESIAN_POINT ( 'NONE',  ( -8.571926809382608425, 26.38167802310805854, 140.4750000027312069 ) ) ;
#176138=CARTESIAN_POINT ( 'NONE',  ( -8.571926809382601320, -26.38167802310801591, 141.7750000027311899 ) ) ;
#176152=CARTESIAN_POINT ( 'NONE',  ( 27.73933785331498925, -9.013057229001034898, 146.2750000027311899 ) ) ;
#176176=ORIENTED_EDGE ( 'NONE', *, *, #4069, .F. ) ;
#176182=DIRECTION ( 'NONE',  ( 0.000000000000000000, 0.000000000000000000, 1.000000000000000000 ) ) ;
#176225=CARTESIAN_POINT ( 'NONE',  ( -21.93180397000028492, 9.000796715316637275, 171.3297436093417900 ) ) ;
#176267=CARTESIAN_POINT ( 'NONE',  ( 20.56371838171434874, 11.43208494587337043, 170.0924998638764976 ) ) ;
#176367=CARTESIAN_POINT ( 'NONE',  ( -26.26083487095749902, 9.141127703660897552, 167.1337248662267996 ) ) ;
#176519=EDGE_CURVE ( 'NONE', #86852, #110081, #9826, .T. ) ;
#176577=CARTESIAN_POINT ( 'NONE',  ( 17.79613651744293534, 24.49428055684532524, 147.2843446568999752 ) ) ;
#176588=CARTESIAN_POINT ( 'NONE',  ( 27.86188877291512611, 7.554847477543872536, 161.1024127393341132 ) ) ;
#176758=CARTESIAN_POINT ( 'NONE',  ( 27.95720134624915687, -7.331398113984718634, 160.9065205403411198 ) ) ;
#176833=( GEOMETRIC_REPRESENTATION_CONTEXT ( 3 ) GLOBAL_UNCERTAINTY_ASSIGNED_CONTEXT ( ( #68125 ) ) GLOBAL_UNIT_ASSIGNED_CONTEXT ( ( #63898, #154908, #185252 ) ) REPRESENTATION_CONTEXT ( 'NONE', 'WORKASPACE' ) );
#176916=DIRECTION ( 'NONE',  ( 0.000000000000000000, 0.000000000000000000, -1.000000000000000000 ) ) ;
#176927=EDGE_CURVE ( 'NONE', #147212, #51307, #164705, .T. ) ;
#176946=CARTESIAN_POINT ( 'NONE',  ( 26.79475375365586132, 2.756753960551091991E-14, 139.9999999999999716 ) ) ;
#176967=CARTESIAN_POINT ( 'NONE',  ( -27.40250423668980417, -7.751724348666604314, 163.3149731962997748 ) ) ;
#176999=EDGE_CURVE ( 'NONE', #116956, #155416, #83239, .T. ) ;
#177002=ORIENTED_EDGE ( 'NONE', *, *, #168410, .T. ) ;
#177088=CARTESIAN_POINT ( 'NONE',  ( -24.81835718235489097, -6.052279806424480491, 168.4265042179603427 ) ) ;
#177092=CARTESIAN_POINT ( 'NONE',  ( 17.14385361876520264, 23.59649016807275856, 142.1750000027311671 ) ) ;
#177128=ORIENTED_EDGE ( 'NONE', *, *, #190970, .F. ) ;
#177148=CARTESIAN_POINT ( 'NONE',  ( 17.81289503416611453, -24.51734667627695785, 140.9500000054623285 ) ) ;
#177161=CARTESIAN_POINT ( 'NONE',  ( 1.784210473542230573E-15, -29.16686587814331588, 141.8750000027311842 ) ) ;
#177190=EDGE_CURVE ( 'NONE', #33758, #163981, #103022, .T. ) ;
#177233=CARTESIAN_POINT ( 'NONE',  ( -24.18299921989881440, 12.77492350451764125, 169.7822198539310250 ) ) ;
#177287=B_SPLINE_CURVE_WITH_KNOTS ( 'NONE', 3,
 ( #42375, #104038, #152517, #58526, #178899, #43361, #14005, #40367, #73716, #181882, #199029, #102041, #119215, #118217 ),
 .UNSPECIFIED., .F., .F.,
 ( 4, 2, 2, 2, 2, 2, 4 ),
 ( 0.1559601203333471908, 0.1570958510570473199, 0.1582315817807474767, 0.1605030432281477348, 0.1616387739518478917, 0.1627745046755480207, 0.1650459661229483066 ),
 .UNSPECIFIED. ) ;
#177313=FACE_OUTER_BOUND ( 'NONE', #154314, .T. ) ;
#177366=VERTEX_POINT ( 'NONE', #100007 ) ;
#177590=CARTESIAN_POINT ( 'NONE',  ( 27.40250423669326096, 7.751724348666389375, 163.3149731962813860 ) ) ;
#177604=VERTEX_POINT ( 'NONE', #194054 ) ;
#177632=CARTESIAN_POINT ( 'NONE',  ( 1.784210473542230573E-15, -29.16686587814331588, 147.8750000027311273 ) ) ;
#177755=CARTESIAN_POINT ( 'NONE',  ( 27.96779038917892279, -7.241162895362543317, 160.9774814432333869 ) ) ;
#177775=CARTESIAN_POINT ( 'NONE',  ( 21.94566984220702466, 7.593969325705130835, 169.8906363267649056 ) ) ;
#177844=CARTESIAN_POINT ( 'NONE',  ( 30.82560697742735201, 2.428612866367529932E-14, 150.0000000000000000 ) ) ;
#177902=EDGE_CURVE ( 'NONE', #82312, #67859, #57450, .T. ) ;
#177972=CARTESIAN_POINT ( 'NONE',  ( 24.17640770809979855, 7.553848413212524981, 169.9412368235690565 ) ) ;
#178143=CARTESIAN_POINT ( 'NONE',  ( -17.81289503416611808, 24.51734667627700404, 139.9500000054623285 ) ) ;
#178157=CARTESIAN_POINT ( 'NONE',  ( 8.571926809382603096, -26.38167802310801235, 145.9750000027311785 ) ) ;
#178227=CARTESIAN_POINT ( 'NONE',  ( -20.69372460268670011, 11.29034304323151794, 170.1224388339879567 ) ) ;
#178270=CARTESIAN_POINT ( 'NONE',  ( 25.41223161463591396, 11.66315983254869693, 166.2610598689586254 ) ) ;
#178281=CARTESIAN_POINT ( 'NONE',  ( -28.82186960331499392, -9.364793116373526516, 148.0999999999999943 ) ) ;
#178341=DIRECTION ( 'NONE',  ( 0.1039620511844979306, -0.1039620511844979306, 0.9891328443778538704 ) ) ;
#178366=CARTESIAN_POINT ( 'NONE',  ( -26.33854305698159592, 8.833284547248199559, 167.2806188263833747 ) ) ;
#178384=ORIENTED_EDGE ( 'NONE', *, *, #34091, .T. ) ;
#178449=CARTESIAN_POINT ( 'NONE',  ( -22.96528548301343520, -5.795830589372932273, 190.0000000000000000 ) ) ;
#178481=EDGE_CURVE ( 'NONE', #148543, #51216, #37829, .T. ) ;
#178669=CARTESIAN_POINT ( 'NONE',  ( 21.35462415990328111, -9.648971641164415303, 168.5494316893070845 ) ) ;
#178826=CARTESIAN_POINT ( 'NONE',  ( 26.45595770381629563, -7.620359626981993983, 168.5711898564603359 ) ) ;
#178899=CARTESIAN_POINT ( 'NONE',  ( 24.60782808046175774, -7.576750539519846228, 167.2921137806583829 ) ) ;
#178964=CARTESIAN_POINT ( 'NONE',  ( -27.93407901760531686, -7.419329114331087993, 160.9060561962049860 ) ) ;
#179071=CARTESIAN_POINT ( 'NONE',  ( -28.79475375365593592, 9.355982642739137489, 141.8843446568999980 ) ) ;
#179150=CARTESIAN_POINT ( 'NONE',  ( 1.784210473542230573E-15, -29.16686587814331588, 139.8750000027311842 ) ) ;
#179151=CARTESIAN_POINT ( 'NONE',  ( -28.82186960331499392, -9.364793116373526516, 138.3500000054623911 ) ) ;
#179164=CARTESIAN_POINT ( 'NONE',  ( 1.784210473542230573E-15, -29.16686587814331588, 143.8750000027311842 ) ) ;
#179235=CARTESIAN_POINT ( 'NONE',  ( -26.62494319856312686, 7.396441074661496806, 168.1134502243650104 ) ) ;
#179279=CARTESIAN_POINT ( 'NONE',  ( 21.35462415990330243, 10.43496131973800090, 170.3924512066482748 ) ) ;
#179283=ORIENTED_EDGE ( 'NONE', *, *, #47103, .T. ) ;
#179292=CARTESIAN_POINT ( 'NONE',  ( -23.31738231874055600, 16.94106989632528837, 147.7999999999999829 ) ) ;
#179325=CARTESIAN_POINT ( 'NONE',  ( -8.898068258721474777, 27.38543819252877398, 145.8656553485623704 ) ) ;
#179359=DIRECTION ( 'NONE',  ( -1.000000000000000000, 0.000000000000000000, 0.000000000000000000 ) ) ;
#179447=CARTESIAN_POINT ( 'NONE',  ( -27.73933785331498925, 2.428612866367529932E-14, 144.8750000027311842 ) ) ;
#179460=DIRECTION ( 'NONE',  ( 0.000000000000000000, 0.000000000000000000, 1.000000000000000000 ) ) ;
#179582=EDGE_LOOP ( 'NONE', ( #197710, #300, #147692, #179659 ) ) ;
#179638=CARTESIAN_POINT ( 'NONE',  ( -22.44159573604010305, 16.30477369853692338, 147.1750000027311671 ) ) ;
#179642=( BOUNDED_CURVE ( )  B_SPLINE_CURVE ( 3, ( #148509, #9999, #121139, #10997 ),
 .UNSPECIFIED., .F., .F. ) 
 B_SPLINE_CURVE_WITH_KNOTS ( ( 4, 4 ),
 ( 5.503250352303675541, 7.063120262055496923 ),
 .UNSPECIFIED. ) 
 CURVE ( )  GEOMETRIC_REPRESENTATION_ITEM ( )  RATIONAL_B_SPLINE_CURVE ( ( 1.000000000000000000, 0.8073061876036304874, 0.8073061876036304874, 1.000000000000000000 ) ) 
 REPRESENTATION_ITEM ( '' )  );
#179652=ORIENTED_EDGE ( 'NONE', *, *, #134205, .F. ) ;
#179659=ORIENTED_EDGE ( 'NONE', *, *, #61925, .T. ) ;
#179680=CARTESIAN_POINT ( 'NONE',  ( 24.27957997113507815, -6.290849861785656749, 171.5443985711291361 ) ) ;
#179708=CARTESIAN_POINT ( 'NONE',  ( 24.95432927374997334, -3.806786798636382141, 190.0000000000000000 ) ) ;
#179724=DIRECTION ( 'NONE',  ( -0.1039620511844979306, 0.1039620511844979306, 0.9891328443778538704 ) ) ;
#179816=CARTESIAN_POINT ( 'NONE',  ( -24.13384886353222214, -15.22194871136943206, 140.0000000000000000 ) ) ;
#179818=CARTESIAN_POINT ( 'NONE',  ( -20.09035150276022463, 11.70762861043687764, 168.0245124264526453 ) ) ;
#179884=CARTESIAN_POINT ( 'NONE',  ( -21.34799762026588255, 10.44447989802408827, 170.3878604776606096 ) ) ;
#179891=CARTESIAN_POINT ( 'NONE',  ( -28.79475375365586842, 2.428612866367529932E-14, 155.0000000000000000 ) ) ;
#179968=CARTESIAN_POINT ( 'NONE',  ( 25.25560589046783022, 2.428612866367529932E-14, 167.9999999999999716 ) ) ;
#179973=CARTESIAN_POINT ( 'NONE',  ( -27.96111904526444292, -7.044650443050448629, 161.2906300811048368 ) ) ;
#179987=CARTESIAN_POINT ( 'NONE',  ( 21.81230582904511550, 5.969922009377570227, 172.1979875755936860 ) ) ;
#180003=VECTOR ( 'NONE', #124148, 1000.000000000000000 ) ;
#180082=CARTESIAN_POINT ( 'NONE',  ( -27.86147134968503991, 7.555459793078377118, 161.1037931155424303 ) ) ;
#180097=DIRECTION ( 'NONE',  ( 0.8437662581494459468, -0.5367108174878556515, 0.000000000000000000 ) ) ;
#180158=CARTESIAN_POINT ( 'NONE',  ( 8.571926809382603096, -26.38167802310801235, 147.4750000027311785 ) ) ;
#180160=EDGE_LOOP ( 'NONE', ( #172268, #134882, #95295, #48246, #161907, #114441 ) ) ;
#180194=ORIENTED_EDGE ( 'NONE', *, *, #176519, .F. ) ;
#180240=CARTESIAN_POINT ( 'NONE',  ( -24.05407591190764549, 13.01182159662891635, 169.7785964492052244 ) ) ;
#180282=CARTESIAN_POINT ( 'NONE',  ( 21.96844466259091533, 8.667631922777363940, 171.6690673070886533 ) ) ;
#180284=ORIENTED_EDGE ( 'NONE', *, *, #97731, .T. ) ;
#180295=CARTESIAN_POINT ( 'NONE',  ( -5.429308488886486681E-15, 30.30510711980690175, 149.5000000000000000 ) ) ;
#180367=EDGE_LOOP ( 'NONE', ( #177002, #182312, #47767 ) ) ;
#180380=CARTESIAN_POINT ( 'NONE',  ( 27.88129983271663903, -6.733757357602863536, 162.1517353552116560 ) ) ;
#180437=CARTESIAN_POINT ( 'NONE',  ( -21.72193145969974992, -8.667250440200811923, 169.0624054586918987 ) ) ;
#180461=CARTESIAN_POINT ( 'NONE',  ( 25.79025989231048399, 10.69883710965548929, 166.5180000355202310 ) ) ;
#180547=AXIS2_PLACEMENT_3D ( 'NONE', #69766, #100093, #161777 ) ;
#180603=ADVANCED_FACE ( 'NONE', ( #166843 ), #173767, .F. ) ;
#180679=CARTESIAN_POINT ( 'NONE',  ( 20.93662873023546211, -10.44628751056279015, 168.2749732860603444 ) ) ;
#180830=( BOUNDED_CURVE ( )  B_SPLINE_CURVE ( 2, ( #13090, #41434, #56603, #167756, #90886, #75729, #199085, #73773, #118277, #25285, #148610 ),
 .UNSPECIFIED., .F., .T. ) 
 B_SPLINE_CURVE_WITH_KNOTS ( ( 3, 2, 2, 2, 2, 3 ),
 ( 0.2000000000000001776, 0.2199999999999996403, 0.2399999999999991029, 0.2599999999999985656, 0.2799999999999980282, 0.2999999999999974909 ),
 .UNSPECIFIED. ) 
 CURVE ( )  GEOMETRIC_REPRESENTATION_ITEM ( )  RATIONAL_B_SPLINE_CURVE ( ( 0.9999999999999994449, 0.9510565162951540863, 1.000000000000000000, 0.9510565162951535312, 1.000000000000000000, 0.9510565162951535312, 1.000000000000000000, 0.9510565162951535312, 1.000000000000000000, 0.9510565162951597484, 0.9999999999999937828 ) ) 
 REPRESENTATION_ITEM ( '' )  );
#180986=ORIENTED_EDGE ( 'NONE', *, *, #124720, .F. ) ;
#181043=CARTESIAN_POINT ( 'NONE',  ( -5.427562675786936573E-15, 30.27659582821221207, 141.7656553485623760 ) ) ;
#181145=CARTESIAN_POINT ( 'NONE',  ( -27.73933785331498925, -9.013057229001049109, 140.9750000027311501 ) ) ;
#181181=ORIENTED_EDGE ( 'NONE', *, *, #75553, .F. ) ;
#181228=CARTESIAN_POINT ( 'NONE',  ( 5.281959635518922447, -27.36706763425078748, 140.0000000000000000 ) ) ;
#181282=CARTESIAN_POINT ( 'NONE',  ( -8.906447517083053711, -27.41122689804191026, 148.4000000000000057 ) ) ;
#181297=CARTESIAN_POINT ( 'NONE',  ( 19.49401214000073779, -12.39993551617566503, 169.9999999999999716 ) ) ;
#181356=CARTESIAN_POINT ( 'NONE',  ( 28.79475375365586132, 2.781246896534039337E-14, 155.0000000000000000 ) ) ;
#181432=CARTESIAN_POINT ( 'NONE',  ( -27.73933785331498925, 2.428612866367529932E-14, 148.8750000027311842 ) ) ;
#181568=CARTESIAN_POINT ( 'NONE',  ( 20.61108013404306405, -10.97331748574078780, 168.1441487092657781 ) ) ;
#181620=CARTESIAN_POINT ( 'NONE',  ( 8.571926809382597767, 26.38167802310806209, 142.7750000027311899 ) ) ;
#181717=ADVANCED_FACE ( 'NONE', ( #3915 ), #113083, .T. ) ;
#181854=DIRECTION ( 'NONE',  ( 1.000000000000000000, 0.000000000000000000, 0.000000000000000000 ) ) ;
#181860=CARTESIAN_POINT ( 'NONE',  ( -21.91636330721479808, -8.102911641865347292, 172.4379571683061556 ) ) ;
#181866=VERTEX_POINT ( 'NONE', #127255 ) ;
#181882=CARTESIAN_POINT ( 'NONE',  ( 23.42531737588076979, -11.30614151570997272, 165.8025732123263936 ) ) ;
#181921=VERTEX_POINT ( 'NONE', #143417 ) ;
#181963=CARTESIAN_POINT ( 'NONE',  ( -27.73933785331498925, 2.428612866367529932E-14, 146.8750000027311842 ) ) ;
#182049=CARTESIAN_POINT ( 'NONE',  ( -28.79475375365586842, 2.428612866367529932E-14, 141.9843446568999923 ) ) ;
#182088=DIRECTION ( 'NONE',  ( 1.000000000000000000, 0.000000000000000000, 0.000000000000000000 ) ) ;
#182124=CARTESIAN_POINT ( 'NONE',  ( -27.73933785331498925, 2.428612866367529932E-14, 146.8750000027311842 ) ) ;
#182161=DIRECTION ( 'NONE',  ( 0.000000000000000000, 0.000000000000000000, -1.000000000000000000 ) ) ;
#182205=CARTESIAN_POINT ( 'NONE',  ( -14.34215988523096286, -24.36250104427641006, 140.0000000000000000 ) ) ;
#182248=CARTESIAN_POINT ( 'NONE',  ( 25.80209238092448487, 7.370998251475543661, 174.5109820657625619 ) ) ;
#182249=AXIS2_PLACEMENT_3D ( 'NONE', #47460, #125289, #44479 ) ;
#182262=CARTESIAN_POINT ( 'NONE',  ( 17.81289503416610742, 24.51734667627700404, 149.2999999999999545 ) ) ;
#182290=CARTESIAN_POINT ( 'NONE',  ( -21.98831087263039308, 5.509728484239381885, 173.5901369092266577 ) ) ;
#182305=LINE ( 'NONE', #75107, #49618 ) ;
#182312=ORIENTED_EDGE ( 'NONE', *, *, #7758, .T. ) ;
#182368=CIRCLE ( 'NONE', #198521, 23.10356920737165254 ) ;
#182369=CARTESIAN_POINT ( 'NONE',  ( -24.02130208662955013, -8.352503713167614308, 169.2769999910357512 ) ) ;
#182557=LINE ( 'NONE', #62159, #152722 ) ;
#182611=CARTESIAN_POINT ( 'NONE',  ( -17.14385361876520264, -23.59649016807271593, 143.6750000027311671 ) ) ;
#182615=CARTESIAN_POINT ( 'NONE',  ( 22.44159573604009239, 16.30477369853692693, 144.5750000027311728 ) ) ;
#182652=CARTESIAN_POINT ( 'NONE',  ( -26.77313074627600997, -4.631999166350019514, 170.7390164845734546 ) ) ;
#182830=CYLINDRICAL_SURFACE ( 'NONE', #173089, 2.000000000000001776 ) ;
#182859=DIRECTION ( 'NONE',  ( 0.000000000000000000, 0.000000000000000000, -1.000000000000000000 ) ) ;
#182957=CARTESIAN_POINT ( 'NONE',  ( 22.44159573604009239, 16.30477369853692693, 148.0750000027312012 ) ) ;
#183008=ORIENTED_EDGE ( 'NONE', *, *, #172144, .F. ) ;
#183014=CARTESIAN_POINT ( 'NONE',  ( 23.29544513554940011, 16.92513159979228021, 141.4656553485623931 ) ) ;
#183043=CARTESIAN_POINT ( 'NONE',  ( -27.60788766665604399, 7.718175339870851026, 162.2452582881568617 ) ) ;
#183099=ORIENTED_EDGE ( 'NONE', *, *, #196970, .F. ) ;
#183118=CARTESIAN_POINT ( 'NONE',  ( 8.571926809382603096, -26.38167802310801235, 141.4750000027312069 ) ) ;
#183199=CARTESIAN_POINT ( 'NONE',  ( -21.81230582904512261, 7.807068725604178638, 172.9985625539982550 ) ) ;
#183242=CARTESIAN_POINT ( 'NONE',  ( 21.97054992548844865, 8.562709642470919036, 171.7904333278019351 ) ) ;
#183256=CARTESIAN_POINT ( 'NONE',  ( 28.82186960331498327, 2.781578969918950771E-14, 141.0000000000000000 ) ) ;
#183355=CARTESIAN_POINT ( 'NONE',  ( -23.97133246043718557, -5.390759101651049434, 174.7603932261090733 ) ) ;
#183372=PRODUCT_DEFINITION ( 'UNKNOWN', '', #75881, #64589 ) ;
#183602=CARTESIAN_POINT ( 'NONE',  ( 27.73933785331498214, 9.013057229001095294, 144.4750000027311501 ) ) ;
#183606=CARTESIAN_POINT ( 'NONE',  ( 8.571926809382597767, 26.38167802310806209, 142.7750000027311899 ) ) ;
#183611=FACE_OUTER_BOUND ( 'NONE', #56530, .T. ) ;
#183623=EDGE_CURVE ( 'NONE', #112207, #42860, #15164, .T. ) ;
#183640=DIRECTION ( 'NONE',  ( 0.000000000000000000, 0.000000000000000000, -1.000000000000000000 ) ) ;
#183643=CARTESIAN_POINT ( 'NONE',  ( -20.14845677604829888, -11.85354687992341205, 170.0217845860067598 ) ) ;
#183744=( BOUNDED_SURFACE ( )  B_SPLINE_SURFACE ( 3, 2, ( 
 ( #22282, #37442, #64800 ),
 ( #83933, #49632, #35448 ),
 ( #99102, #110300, #126461 ),
 ( #127450, #80948, #158784 ),
 ( #128439, #156818, #174967 ),
 ( #18310, #143611, #159784 ),
 ( #98086, #113275, #191133 ),
 ( #111295, #145614, #21279 ),
 ( #67778, #114269, #5095 ),
 ( #160794, #7093, #187177 ),
 ( #172984, #175973, #171982 ),
 ( #96121, #157809, #19300 ),
 ( #142623, #4102, #189156 ),
 ( #50629, #147632, #23285 ),
 ( #133451, #177972, #131448 ),
 ( #11122, #88941, #165797 ),
 ( #119292, #130432, #149624 ),
 ( #53612, #118296, #195141 ),
 ( #41455, #104115, #42451 ),
 ( #179987, #84929, #148631 ),
 ( #100106, #163803, #72797 ),
 ( #9120, #10121, #86947 ),
 ( #193135, #71781, #70787 ),
 ( #115288, #56622, #39440 ) ),
 .UNSPECIFIED., .F., .F., .T. ) 
 B_SPLINE_SURFACE_WITH_KNOTS ( ( 4, 2, 2, 2, 2, 2, 2, 2, 2, 2, 2, 4 ),
 ( 3, 3 ),
 ( -8.673617379884035472E-19, 0.001899702839891689908, 0.002849554259837535405, 0.003799405679783380684, 0.005699108519675071677, 0.006648959939620916956, 0.007598811359566762236, 0.008548662779512607515, 0.009498514199458452795, 0.01139821703935014335, 0.01329791987924183391, 0.01519762271913352621 ),
 ( 0.000000000000000000, 1.000000000000000000 ),
 .UNSPECIFIED. ) 
 GEOMETRIC_REPRESENTATION_ITEM ( )  RATIONAL_B_SPLINE_SURFACE ( (
 ( 1.000000000000000000, 0.7660444431189795678, 1.000000000000000000),
 ( 1.000000000000000000, 0.7753720600382404404, 1.000000000000000000),
 ( 1.000000000000000000, 0.7832595754285938128, 1.000000000000000000),
 ( 1.000000000000000000, 0.7928595458705487431, 1.000000000000000000),
 ( 1.000000000000000000, 0.7956872332516284896, 1.000000000000000000),
 ( 1.000000000000000000, 0.8005750596157428234, 1.000000000000000000),
 ( 1.000000000000000000, 0.8026302056541881891, 1.000000000000000000),
 ( 1.000000000000000000, 0.8075080643848097095, 1.000000000000000000),
 ( 1.000000000000000000, 0.8091143015810103867, 1.000000000000000000),
 ( 1.000000000000000000, 0.8093067629632916260, 1.000000000000000000),
 ( 1.000000000000000000, 0.8089952915732693262, 1.000000000000000000),
 ( 1.000000000000000000, 0.8076919994861299079, 1.000000000000000000),
 ( 1.000000000000000000, 0.8067078407648542449, 1.000000000000000000),
 ( 1.000000000000000000, 0.8041786842467808505, 1.000000000000000000),
 ( 1.000000000000000000, 0.8026334674876917097, 1.000000000000000000),
 ( 1.000000000000000000, 0.7990747329469513049, 1.000000000000000000),
 ( 1.000000000000000000, 0.7970509760942319222, 1.000000000000000000),
 ( 1.000000000000000000, 0.7904793850862328330, 1.000000000000000000),
 ( 1.000000000000000000, 0.7855040224315206210, 1.000000000000000000),
 ( 1.000000000000000000, 0.7751942650506107313, 1.000000000000000000),
 ( 1.000000000000000000, 0.7698260778212773214, 1.000000000000000000),
 ( 1.000000000000000000, 0.7598259884959708277, 1.000000000000000000),
 ( 1.000000000000000000, 0.7551428682221226207, 1.000000000000000000),
 ( 1.000000000000000000, 0.7510191126010858920, 1.000000000000000000) ) ) 
 REPRESENTATION_ITEM ( '' )  SURFACE ( )  );
#183790=CARTESIAN_POINT ( 'NONE',  ( 14.30785154961629857, 24.18559174397515577, 140.0000000000000853 ) ) ;
#183942=CARTESIAN_POINT ( 'NONE',  ( 27.73933785331498214, 9.013057229001095294, 143.9750000027312069 ) ) ;
#183979=CARTESIAN_POINT ( 'NONE',  ( -27.39399371936811534, -5.109217719441272010, 166.7881433183803210 ) ) ;
#183983=DIRECTION ( 'NONE',  ( 0.000000000000000000, 0.000000000000000000, 1.000000000000000000 ) ) ;
#183992=ORIENTED_EDGE ( 'NONE', *, *, #35192, .T. ) ;
#184108=CARTESIAN_POINT ( 'NONE',  ( 8.571926809382603096, -26.38167802310801235, 143.4750000027312069 ) ) ;
#184121=CYLINDRICAL_SURFACE ( 'NONE', #1479, 28.79475375365586487 ) ;
#184145=CARTESIAN_POINT ( 'NONE',  ( -8.898068258721467672, -27.38543819252872069, 140.3843446568999696 ) ) ;
#184343=CARTESIAN_POINT ( 'NONE',  ( -24.20757866959952764, -5.698759791480821235, 172.9004493943157001 ) ) ;
#184349=VERTEX_POINT ( 'NONE', #140200 ) ;
#184405=CARTESIAN_POINT ( 'NONE',  ( -26.79475375365586842, 2.428612866367529932E-14, 155.0000000000000000 ) ) ;
#184422=CARTESIAN_POINT ( 'NONE',  ( -8.898068258721467672, -27.38543819252872069, 148.3843446568999980 ) ) ;
#184481=ADVANCED_FACE ( 'NONE', ( #4658 ), #96674, .F. ) ;
#184588=CARTESIAN_POINT ( 'NONE',  ( 27.73933785331498214, 9.013057229001095294, 146.4750000027311501 ) ) ;
#184592=CARTESIAN_POINT ( 'NONE',  ( 8.571926809382603096, -26.38167802310801235, 143.9750000027312069 ) ) ;
#184626=CARTESIAN_POINT ( 'NONE',  ( -25.73063820182027328, -8.702599028573553497, 171.6270364942855053 ) ) ;
#184777=CARTESIAN_POINT ( 'NONE',  ( 1.542446121169174900, 28.32207039655730085, 140.0000000000000568 ) ) ;
#184804=CARTESIAN_POINT ( 'NONE',  ( -22.77340731150486874, -12.66915506687109527, 165.5704399981227937 ) ) ;
#184857=FACE_OUTER_BOUND ( 'NONE', #156409, .T. ) ;
#184869=CARTESIAN_POINT ( 'NONE',  ( -24.14511064691435749, 7.743397529680777325, 169.7652520481140641 ) ) ;
#184892=ORIENTED_EDGE ( 'NONE', *, *, #189014, .T. ) ;
#184931=CARTESIAN_POINT ( 'NONE',  ( 27.73933785331498925, -9.013057229001033122, 145.7750000027311899 ) ) ;
#184944=CARTESIAN_POINT ( 'NONE',  ( 27.89965394715913405, -6.788920637341042230, 161.9771076211712000 ) ) ;
#184968=CARTESIAN_POINT ( 'NONE',  ( -27.05641397906351742, -3.631740835637518927, 169.9999999999999716 ) ) ;
#185007=CARTESIAN_POINT ( 'NONE',  ( -8.898068258721474777, 27.38543819252877043, 143.5843446569000150 ) ) ;
#185094=CARTESIAN_POINT ( 'NONE',  ( 17.14385361876520264, 23.59649016807275856, 146.1750000027311387 ) ) ;
#185232=CARTESIAN_POINT ( 'NONE',  ( -23.31738231874055245, -16.94106989632524574, 142.1999999999999886 ) ) ;
#185250=CARTESIAN_POINT ( 'NONE',  ( 28.79475375365586132, 2.781246896534039337E-14, 143.2656553485623760 ) ) ;
#185252=( NAMED_UNIT ( * ) SI_UNIT ( $, .STERADIAN. ) SOLID_ANGLE_UNIT ( ) );
#185330=CARTESIAN_POINT ( 'NONE',  ( -24.24385185424069533, -7.025880200331405590, 170.5073520790474788 ) ) ;
#185419=LINE ( 'NONE', #28782, #49486 ) ;
#185421=DIRECTION ( 'NONE',  ( 0.1736481776669307198, 0.000000000000000000, -0.9848077530122080203 ) ) ;
#185518=ORIENTED_EDGE ( 'NONE', *, *, #2128, .F. ) ;
#185521=CARTESIAN_POINT ( 'NONE',  ( 21.85375568585899586, -8.111533062293291962, 169.4628294566284126 ) ) ;
#185566=CARTESIAN_POINT ( 'NONE',  ( -3.573655867282028392E-15, 2.428612866367529932E-14, 155.0000000000000000 ) ) ;
#185581=CARTESIAN_POINT ( 'NONE',  ( -27.73933785331498925, 2.428612866367529932E-14, 145.3750000027311842 ) ) ;
#185585=CARTESIAN_POINT ( 'NONE',  ( -27.73933785331498925, 2.428612866367529932E-14, 143.3750000027311842 ) ) ;
#185620=CARTESIAN_POINT ( 'NONE',  ( -21.92083080610932200, -8.096106818373623781, 172.4353877980944674 ) ) ;
#185741=( BOUNDED_CURVE ( )  B_SPLINE_CURVE ( 2, ( #52411, #113081, #33280, #187970, #5903, #142434, #111101, #127253, #37244, #128249, #190934 ),
 .UNSPECIFIED., .F., .F. ) 
 B_SPLINE_CURVE_WITH_KNOTS ( ( 3, 2, 2, 2, 2, 3 ),
 ( 0.1000000000000000888, 0.1200000000000006478, 0.1400000000000012346, 0.1600000000000018074, 0.1800000000000023526, 0.2000000000000029532 ),
 .UNSPECIFIED. ) 
 CURVE ( )  GEOMETRIC_REPRESENTATION_ITEM ( )  RATIONAL_B_SPLINE_CURVE ( ( 0.9999999999999997780, 0.9510565162951537532, 1.000000000000000000, 0.9510565162951535312, 1.000000000000000000, 0.9510565162951535312, 1.000000000000000000, 0.9510565162951535312, 1.000000000000000000, 0.9510565162951463147, 1.000000000000007105 ) ) 
 REPRESENTATION_ITEM ( '' )  );
#185841=ORIENTED_EDGE ( 'NONE', *, *, #45518, .F. ) ;
#185847=LINE ( 'NONE', #79644, #180003 ) ;
#185874=CARTESIAN_POINT ( 'NONE',  ( -24.73536985823982803, 3.645104810711965460, 171.5180696409406380 ) ) ;
#185938=CARTESIAN_POINT ( 'NONE',  ( 22.44159573604009239, 16.30477369853692693, 146.0750000027311728 ) ) ;
#185976=DIRECTION ( 'NONE',  ( 0.000000000000000000, 0.000000000000000000, -1.000000000000000000 ) ) ;
#186051=DIRECTION ( 'NONE',  ( 1.000000000000000000, 0.000000000000000000, -0.000000000000000000 ) ) ;
#186058=VERTEX_POINT ( 'NONE', #158124 ) ;
#186081=DIRECTION ( 'NONE',  ( -0.8660254037844410391, 0.000000000000000000, 0.4999999999999958367 ) ) ;
#186111=CARTESIAN_POINT ( 'NONE',  ( 23.62199046085592613, -10.84149981712626065, 165.9137635136254403 ) ) ;
#186237=CARTESIAN_POINT ( 'NONE',  ( -23.88378066561469382, -7.642901331109204222, 172.4262957903898155 ) ) ;
#186246=CARTESIAN_POINT ( 'NONE',  ( 1.993301997531345292E-15, -30.30510711980685912, 142.4999999999999716 ) ) ;
#186259=CARTESIAN_POINT ( 'NONE',  ( 26.38458505201419513, -8.641005086744103281, 167.3773361139121789 ) ) ;
#186271=CARTESIAN_POINT ( 'NONE',  ( 21.38418241377623019, 5.438282248597753110, 174.2683007571264113 ) ) ;
#186276=DIRECTION ( 'NONE',  ( -1.000000000000000000, 0.000000000000000000, 0.000000000000000000 ) ) ;
#186340=CARTESIAN_POINT ( 'NONE',  ( -21.81230582904511550, -5.969922009378025862, 172.1979875755928049 ) ) ;
#186383=DIRECTION ( 'NONE',  ( -0.1736481776669307198, -2.126576849575776229E-17, -0.9848077530122080203 ) ) ;
#186407=CYLINDRICAL_SURFACE ( 'NONE', #116444, 5.000000000000004441 ) ;
#186792=CARTESIAN_POINT ( 'NONE',  ( -9.572641798195965279, 26.93160034404219161, 140.0000000000000000 ) ) ;
#186859=CARTESIAN_POINT ( 'NONE',  ( 28.79475375365586132, 2.781246896534039337E-14, 144.9843446568999923 ) ) ;
#186884=CARTESIAN_POINT ( 'NONE',  ( -21.97054992548900998, 7.027819292989580191, 170.5066066589220100 ) ) ;
#186949=CARTESIAN_POINT ( 'NONE',  ( -22.44159573604009950, -16.30477369853688430, 141.0750000027311728 ) ) ;
#187038=CARTESIAN_POINT ( 'NONE',  ( -23.64874990377911956, -15.04272038711346582, 165.8682408883346397 ) ) ;
#187074=ORIENTED_EDGE ( 'NONE', *, *, #199705, .F. ) ;
#187089=CARTESIAN_POINT ( 'NONE',  ( -28.28060372831499336, 2.428612866367529932E-14, 149.6875000013656063 ) ) ;
#187111=CARTESIAN_POINT ( 'NONE',  ( -27.73933785331498925, 2.428612866367529932E-14, 138.8750000027311842 ) ) ;
#187160=AXIS2_PLACEMENT_3D ( 'NONE', #128649, #176182, #116499 ) ;
#187177=CARTESIAN_POINT ( 'NONE',  ( 24.51266705573306481, 8.027923408435615471, 167.0300397585818644 ) ) ;
#187260=CARTESIAN_POINT ( 'NONE',  ( 25.85231681326417785, -7.957828899752770191, 172.6576833274880300 ) ) ;
#187264=CARTESIAN_POINT ( 'NONE',  ( -8.898068258721474777, 27.38543819252877398, 143.8656553485623704 ) ) ;
#187340=CARTESIAN_POINT ( 'NONE',  ( 8.906447517083057264, -27.41122689804191026, 146.8500000054623627 ) ) ;
#187430=CARTESIAN_POINT ( 'NONE',  ( -28.79475375365683831, -9.355982642737862065, 142.3656553485623704 ) ) ;
#187507=CARTESIAN_POINT ( 'NONE',  ( 27.69393237830212939, -1.826213041496827616, 140.0000000000000000 ) ) ;
#187645=CARTESIAN_POINT ( 'NONE',  ( 24.95432927374997334, 3.806786798636384805, 190.0000000000000000 ) ) ;
#187780=CARTESIAN_POINT ( 'NONE',  ( 10.31603103613401373, 26.32579789674820958, 139.9999999999999716 ) ) ;
#187788=B_SPLINE_CURVE_WITH_KNOTS ( 'NONE', 3,
 ( #187038, #48508, #110162, #171841, #91987, #978, #153682, #62654, #15178, #76837, #33329, #200191, #61659, #4950 ),
 .UNSPECIFIED., .F., .F.,
 ( 4, 2, 2, 2, 2, 2, 4 ),
 ( 0.000000000000000000, 0.002096066633256099630, 0.003144099949884144891, 0.004192133266512189718, 0.006288199899768280240, 0.007336233216396328104, 0.008384266533024375967 ),
 .UNSPECIFIED. ) ;
#187868=CARTESIAN_POINT ( 'NONE',  ( -24.85114155361848276, 5.582993631601033790, 168.8590791472286412 ) ) ;
#187933=CARTESIAN_POINT ( 'NONE',  ( 27.73933785331498925, -9.013057229001033122, 141.7750000027311899 ) ) ;
#187970=CARTESIAN_POINT ( 'NONE',  ( 17.79613651744294245, -24.49428055684527550, 146.9656553485623931 ) ) ;
#188040=CARTESIAN_POINT ( 'NONE',  ( -3.573655867282028392E-15, 2.428612866367529932E-14, 169.9999999999999716 ) ) ;
#188060=CARTESIAN_POINT ( 'NONE',  ( -28.79475375365586842, 2.428612866367529932E-14, 145.9843446568999923 ) ) ;
#188071=DIRECTION ( 'NONE',  ( -0.1045284632676537068, 0.000000000000000000, 0.9945218953682734009 ) ) ;
#188128=CARTESIAN_POINT ( 'NONE',  ( 24.74823625077140932, -6.005039613785480235, 168.8763313249075395 ) ) ;
#188240=CARTESIAN_POINT ( 'NONE',  ( 21.92083080610931489, -8.096106818373623781, 172.4353877980944674 ) ) ;
#188247=SURFACE_STYLE_USAGE ( .BOTH. , #142713 ) ;
#188320=CARTESIAN_POINT ( 'NONE',  ( 17.81289503416610742, 24.51734667627700404, 147.5500000054623229 ) ) ;
#188382=CARTESIAN_POINT ( 'NONE',  ( 28.79475375365586132, 2.781246896534039337E-14, 147.2656553485624045 ) ) ;
#188487=CARTESIAN_POINT ( 'NONE',  ( 13.91092067181850922, -24.01619779967536417, 139.9999999999999716 ) ) ;
#188600=CARTESIAN_POINT ( 'NONE',  ( 25.38323934330066578, -4.814940836774085575, 166.7856488131975539 ) ) ;
#188768=CARTESIAN_POINT ( 'NONE',  ( 26.70615770596319649, 7.662262839729889308, 167.2520072419550559 ) ) ;
#188858=CARTESIAN_POINT ( 'NONE',  ( -24.50238749460114462, 2.981321037229033521, 173.3223451563238200 ) ) ;
#188928=CARTESIAN_POINT ( 'NONE',  ( 8.571926809382603096, -26.38167802310801235, 141.4750000027312069 ) ) ;
#189014=EDGE_CURVE ( 'NONE', #119499, #103252, #132248, .T. ) ;
#189038=CARTESIAN_POINT ( 'NONE',  ( -28.79475375365586842, 2.428612866367529932E-14, 140.2656553485623760 ) ) ;
#189051=PLANE ( 'NONE',  #51768 ) ;
#189064=AXIS2_PLACEMENT_3D ( 'NONE', #95231, #156917, #81048 ) ;
#189129=CARTESIAN_POINT ( 'NONE',  ( 24.62642639703176073, -5.957135776930575943, 169.3344962860537350 ) ) ;
#189156=CARTESIAN_POINT ( 'NONE',  ( 24.72709851008551496, 6.869189314501217503, 167.7661538690258567 ) ) ;
#189239=CARTESIAN_POINT ( 'NONE',  ( 21.96844466259035400, -8.667631922777625064, 171.6690673070883690 ) ) ;
#189318=CARTESIAN_POINT ( 'NONE',  ( 17.14385361876520264, -23.59649016807271238, 148.0750000027311728 ) ) ;
#189319=CARTESIAN_POINT ( 'NONE',  ( -17.81289503416611808, 24.51734667627700404, 143.9500000054623854 ) ) ;
#189351=CIRCLE ( 'NONE', #15010, 28.79475375365586487 ) ;
#189370=FACE_OUTER_BOUND ( 'NONE', #107900, .T. ) ;
#189405=CARTESIAN_POINT ( 'NONE',  ( 17.79613651744294245, -24.49428055684527550, 142.9656553485623931 ) ) ;
#189407=CIRCLE ( 'NONE', #95719, 26.79475375365586487 ) ;
#189536=VERTEX_POINT ( 'NONE', #61408 ) ;
#189586=PLANE ( 'NONE',  #124495 ) ;
#189722=CARTESIAN_POINT ( 'NONE',  ( 26.33854305698156395, -8.833284547248206664, 167.2806188263833747 ) ) ;
#189761=CARTESIAN_POINT ( 'NONE',  ( 27.77709992218785828, 7.633332386730715236, 161.4489275245684041 ) ) ;
#189884=DIRECTION ( 'NONE',  ( -0.000000000000000000, -0.000000000000000000, -1.000000000000000000 ) ) ;
#189907=CARTESIAN_POINT ( 'NONE',  ( 21.92716348790884240, 9.076607822308496054, 171.2490935175191282 ) ) ;
#189965=CARTESIAN_POINT ( 'NONE',  ( -3.573655867282028392E-15, 2.428612866367529932E-14, 155.0000000000000000 ) ) ;
#190107=CARTESIAN_POINT ( 'NONE',  ( 21.38418241377623019, -5.438282248597753110, 174.2683007571264113 ) ) ;
#190136=FACE_OUTER_BOUND ( 'NONE', #66383, .T. ) ;
#190143=DIRECTION ( 'NONE',  ( 1.000000000000000000, 0.000000000000000000, 0.000000000000000000 ) ) ;
#190200=CARTESIAN_POINT ( 'NONE',  ( -25.66098555633789857, 7.783268508282411346, 170.2231668181882753 ) ) ;
#190220=CARTESIAN_POINT ( 'NONE',  ( 21.75836449082841284, -9.620754668593853864, 170.8405250346328046 ) ) ;
#190245=CARTESIAN_POINT ( 'NONE',  ( 17.14385361876520264, 23.59649016807275856, 144.1750000027311671 ) ) ;
#190301=CARTESIAN_POINT ( 'NONE',  ( 28.82186960331498327, 9.364793116373570925, 143.3500000054623342 ) ) ;
#190315=CARTESIAN_POINT ( 'NONE',  ( 27.73933785331498925, -9.013057229001034898, 148.2750000027311614 ) ) ;
#190364=CARTESIAN_POINT ( 'NONE',  ( 27.88129983271663903, -6.733757357602863536, 162.1517353552116560 ) ) ;
#190430=CARTESIAN_POINT ( 'NONE',  ( 20.69372460268669300, 11.29034304323151794, 170.1224388339879567 ) ) ;
#190457=CIRCLE ( 'NONE', #109772, 26.79475375365586487 ) ;
#190461=ORIENTED_EDGE ( 'NONE', *, *, #199705, .T. ) ;
#190477=CARTESIAN_POINT ( 'NONE',  ( -23.29544513554941076, 16.92513159979227666, 146.0656553485623590 ) ) ;
#190555=CYLINDRICAL_SURFACE ( 'NONE', #53819, 28.79475375365586487 ) ;
#190591=CARTESIAN_POINT ( 'NONE',  ( -26.36463166569307859, -3.076743934663885405, 174.2851114983685932 ) ) ;
#190668=ORIENTED_EDGE ( 'NONE', *, *, #101580, .F. ) ;
#190727=DIRECTION ( 'NONE',  ( 0.000000000000000000, -0.1045284632676537068, 0.9945218953682734009 ) ) ;
#190747=CARTESIAN_POINT ( 'NONE',  ( 27.67912082740223312, 7.698001346386336152, 161.8872396492157577 ) ) ;
#190783=CARTESIAN_POINT ( 'NONE',  ( -3.573655867282028392E-15, 2.428612866367529932E-14, 167.9999999999999716 ) ) ;
#190793=CARTESIAN_POINT ( 'NONE',  ( -22.72581825106521336, -12.75361973299659368, 165.5645137041830708 ) ) ;
#190914=ORIENTED_EDGE ( 'NONE', *, *, #162246, .T. ) ;
#190934=CARTESIAN_POINT ( 'NONE',  ( -28.79475375365586842, 2.428612866367529932E-14, 146.2656553485623760 ) ) ;
#190970=EDGE_CURVE ( 'NONE', #177604, #181866, #170738, .T. ) ;
#191119=CARTESIAN_POINT ( 'NONE',  ( -27.60805440473040662, -7.718125693464772397, 162.2444234560585130 ) ) ;
#191133=CARTESIAN_POINT ( 'NONE',  ( 23.75112013235324326, 10.51683317207912971, 166.0021274478077089 ) ) ;
#191206=LINE ( 'NONE', #41532, #66792 ) ;
#191241=CARTESIAN_POINT ( 'NONE',  ( 24.38138396336205815, 13.63488425290815620, 140.0383846261352403 ) ) ;
#191306=CARTESIAN_POINT ( 'NONE',  ( -22.44159573604010305, 16.30477369853692338, 141.1750000027311671 ) ) ;
#191364=ADVANCED_FACE ( 'NONE', ( #32732 ), #94384, .T. ) ;
#191419=CARTESIAN_POINT ( 'NONE',  ( 24.06609220500514468, 14.38661408136930753, 165.8682408874382475 ) ) ;
#191502=ORIENTED_EDGE ( 'NONE', *, *, #49707, .T. ) ;
#191657=ORIENTED_EDGE ( 'NONE', *, *, #7758, .F. ) ;
#191734=LINE ( 'NONE', #175575, #46910 ) ;
#191823=CARTESIAN_POINT ( 'NONE',  ( 24.22576942085219542, -7.195495839727257703, 170.3116806589272301 ) ) ;
#191868=CARTESIAN_POINT ( 'NONE',  ( 24.79445753310783829, 6.337991946471497329, 168.1742925226654108 ) ) ;
#191903=CARTESIAN_POINT ( 'NONE',  ( 27.91261209101638840, -7.473227146837556845, 160.9450349587941957 ) ) ;
#191910=ADVANCED_FACE ( 'NONE', ( #84182 ), #140009, .T. ) ;
#191977=LINE ( 'NONE', #111152, #195567 ) ;
#192011=B_SPLINE_CURVE_WITH_KNOTS ( 'NONE', 3,
 ( #142758, #154956, #94268, #34596 ),
 .UNSPECIFIED., .F., .F.,
 ( 4, 4 ),
 ( 0.000000000000000000, 0.007966019813518861181 ),
 .UNSPECIFIED. ) ;
#192013=CARTESIAN_POINT ( 'NONE',  ( 27.05641397906351386, 3.631740835637567333, 169.9999999999999716 ) ) ;
#192028=SURFACE_STYLE_USAGE ( .BOTH. , #51520 ) ;
#192069=( GEOMETRIC_REPRESENTATION_CONTEXT ( 3 ) GLOBAL_UNCERTAINTY_ASSIGNED_CONTEXT ( ( #35798 ) ) GLOBAL_UNIT_ASSIGNED_CONTEXT ( ( #127353, #116191, #21182 ) ) REPRESENTATION_CONTEXT ( 'NONE', 'WORKASPACE' ) );
#192109=EDGE_CURVE ( 'NONE', #144449, #82312, #158723, .T. ) ;
#192116=CARTESIAN_POINT ( 'NONE',  ( -27.83962847747548608, -7.578403945695542987, 161.1890875224084709 ) ) ;
#192195=ORIENTED_EDGE ( 'NONE', *, *, #16394, .F. ) ;
#192303=CARTESIAN_POINT ( 'NONE',  ( -8.571926809382601320, -26.38167802310801591, 139.7750000027311899 ) ) ;
#192304=CARTESIAN_POINT ( 'NONE',  ( 8.571926809382597767, 26.38167802310806209, 148.2750000027311899 ) ) ;
#192317=CARTESIAN_POINT ( 'NONE',  ( -27.73933785331498925, 2.428612866367529932E-14, 145.3750000027311842 ) ) ;
#192431=CARTESIAN_POINT ( 'NONE',  ( 24.05407591190764194, 13.01182159662919346, 169.7785964492052244 ) ) ;
#192508=CARTESIAN_POINT ( 'NONE',  ( -3.573655867282028392E-15, 2.428612866367529932E-14, 155.0000000000000000 ) ) ;
#192604=( BOUNDED_CURVE ( )  B_SPLINE_CURVE ( 3, ( #25665, #163154, #24657, #86306 ),
 .UNSPECIFIED., .F., .T. ) 
 B_SPLINE_CURVE_WITH_KNOTS ( ( 4, 4 ),
 ( 5.503250352303675541, 7.063120262055497811 ),
 .UNSPECIFIED. ) 
 CURVE ( )  GEOMETRIC_REPRESENTATION_ITEM ( )  RATIONAL_B_SPLINE_CURVE ( ( 1.000000000000000000, 0.8073061876036302653, 0.8073061876036302653, 1.000000000000000000 ) ) 
 REPRESENTATION_ITEM ( '' )  );
#192736=CARTESIAN_POINT ( 'NONE',  ( -23.29544513554941076, 16.92513159979227666, 147.7843446569000037 ) ) ;
#192746=CARTESIAN_POINT ( 'NONE',  ( 27.96809023454798648, 7.159247544362251858, 161.0916313341443811 ) ) ;
#192772=CARTESIAN_POINT ( 'NONE',  ( -24.75981654686067657, 6.635759577896799932, 167.9384007923203797 ) ) ;
#192788=CARTESIAN_POINT ( 'NONE',  ( -5.359611314223446995E-15, 29.16686587814335496, 148.8750000027311842 ) ) ;
#192832=CARTESIAN_POINT ( 'NONE',  ( 21.51693143705270828, -9.260949364272995865, 168.7281092719938442 ) ) ;
#192849=EDGE_CURVE ( 'NONE', #177366, #83996, #146502, .T. ) ;
#192880=CARTESIAN_POINT ( 'NONE',  ( 24.20533859822809930, 9.236745700548663507, 166.4300890397317971 ) ) ;
#192985=CARTESIAN_POINT ( 'NONE',  ( 24.12203661075783501, 5.823883908176390456, 170.5995460337422571 ) ) ;
#193101=VECTOR ( 'NONE', #70694, 1000.000000000000000 ) ;
#193121=CARTESIAN_POINT ( 'NONE',  ( -26.70615770596270622, -7.662262839729761410, 167.2520072419578980 ) ) ;
#193135=CARTESIAN_POINT ( 'NONE',  ( 21.47377332591981514, 5.474134792251744486, 173.8918256800989468 ) ) ;
#193218=EDGE_LOOP ( 'NONE', ( #73856, #30850, #45432, #70267 ) ) ;
#193227=CARTESIAN_POINT ( 'NONE',  ( 28.79475375365583290, 9.355982642739277821, 141.0843446569000150 ) ) ;
#193248=CARTESIAN_POINT ( 'NONE',  ( -8.571926809382601320, -26.38167802310801591, 143.2750000027311899 ) ) ;
#193306=CARTESIAN_POINT ( 'NONE',  ( -17.81289503416611097, -24.51734667627696496, 142.5500000054623513 ) ) ;
#193319=CARTESIAN_POINT ( 'NONE',  ( 17.14385361876520264, 23.59649016807275856, 144.6750000027311671 ) ) ;
#193389=CARTESIAN_POINT ( 'NONE',  ( -23.64729612845683349, 13.72274676820478412, 169.8070494178799663 ) ) ;
#193432=CARTESIAN_POINT ( 'NONE',  ( 24.42783677680703391, 12.30119602009721014, 169.8172178118632587 ) ) ;
#193436=VERTEX_POINT ( 'NONE', #173829 ) ;
#193444=CARTESIAN_POINT ( 'NONE',  ( -28.82186960331499037, 2.428612866367529932E-14, 150.0000000000000000 ) ) ;
#193503=CIRCLE ( 'NONE', #15832, 28.02760797243269408 ) ;
#193604=CARTESIAN_POINT ( 'NONE',  ( -17.14385361876520264, -23.59649016807271238, 147.1750000027311671 ) ) ;
#193676=EDGE_CURVE ( 'NONE', #136214, #107664, #17917, .T. ) ;
#193717=B_SPLINE_CURVE_WITH_KNOTS ( 'NONE', 3,
 ( #128505, #172042, #156877, #95191, #35515, #18374, #190200, #51678, #80026, #142686 ),
 .UNSPECIFIED., .F., .F.,
 ( 4, 2, 2, 2, 4 ),
 ( 0.000000000000000000, 0.0009193652485011039217, 0.001838730497002207843, 0.002758095745503311765, 0.003677460994004415687 ),
 .UNSPECIFIED. ) ;
#193796=CARTESIAN_POINT ( 'NONE',  ( 27.73933785331498569, 2.768321779492822058E-14, 148.3750000027311842 ) ) ;
#193841=CARTESIAN_POINT ( 'NONE',  ( 21.75836449082896706, -8.509082329561300284, 169.1767350484858810 ) ) ;
#193877=EDGE_CURVE ( 'NONE', #107606, #45770, #185419, .T. ) ;
#193946=CARTESIAN_POINT ( 'NONE',  ( 21.82787714368445009, 6.011549001344959287, 172.1028946673681048 ) ) ;
#193971=AXIS2_PLACEMENT_3D ( 'NONE', #172730, #78709, #18060 ) ;
#194054=CARTESIAN_POINT ( 'NONE',  ( 28.79475375365586132, 2.781246896534039337E-14, 146.9843446568999923 ) ) ;
#194096=CARTESIAN_POINT ( 'NONE',  ( -27.73933785331498925, 2.428612866367529932E-14, 149.3750000027311842 ) ) ;
#194133=CARTESIAN_POINT ( 'NONE',  ( -27.91695578976807823, -6.846979738067211940, 161.8037495850383607 ) ) ;
#194235=CARTESIAN_POINT ( 'NONE',  ( -5.427562675786936573E-15, 30.27659582821221207, 141.4843446568999923 ) ) ;
#194256=CARTESIAN_POINT ( 'NONE',  ( 8.571926809382597767, 26.38167802310806209, 144.2750000027311899 ) ) ;
#194274=ORIENTED_EDGE ( 'NONE', *, *, #136776, .T. ) ;
#194312=CARTESIAN_POINT ( 'NONE',  ( -22.44159573604010305, 16.30477369853692338, 141.1750000027311671 ) ) ;
#194313=CARTESIAN_POINT ( 'NONE',  ( 28.82186960331498327, 9.364793116373570925, 141.3500000054623627 ) ) ;
#194326=CARTESIAN_POINT ( 'NONE',  ( 17.14385361876520264, -23.59649016807270883, 144.0750000027311444 ) ) ;
#194347=CARTESIAN_POINT ( 'NONE',  ( 24.81835880841864039, -6.052260367207979996, 168.4265213779230521 ) ) ;
#194435=CARTESIAN_POINT ( 'NONE',  ( 21.70479006154310397, 9.754118203517286645, 170.7545476126474284 ) ) ;
#194445=CARTESIAN_POINT ( 'NONE',  ( -23.31738231874055600, 16.94106989632528837, 149.7999999999999829 ) ) ;
#194463=ORIENTED_EDGE ( 'NONE', *, *, #162141, .F. ) ;
#194590=CARTESIAN_POINT ( 'NONE',  ( -21.48956683882228091, -5.485153550827159386, 173.8223501052718802 ) ) ;
#194602=CARTESIAN_POINT ( 'NONE',  ( -17.14385361876520264, -23.59649016807271238, 145.1750000027311387 ) ) ;
#194613=CARTESIAN_POINT ( 'NONE',  ( 24.02723517065434322, 14.44770145514793214, 165.8682408883346966 ) ) ;
#194670=EDGE_CURVE ( 'NONE', #184349, #37352, #106364, .T. ) ;
#194732=CARTESIAN_POINT ( 'NONE',  ( -29.15849868437705439, 8.010956209263452976, 149.7909430734646890 ) ) ;
#194799=CARTESIAN_POINT ( 'NONE',  ( -27.16945489364050559, -10.00000000000000000, 149.7909430734646890 ) ) ;
#194835=CARTESIAN_POINT ( 'NONE',  ( 23.91168844458706033, -8.792376985857295324, 168.9858545422794123 ) ) ;
#194972=CARTESIAN_POINT ( 'NONE',  ( -21.44820451018248875, 9.431764332217083435, 168.6453917704523633 ) ) ;
#194989=AXIS2_PLACEMENT_3D ( 'NONE', #150738, #10230, #118405 ) ;
#195013=ADVANCED_FACE ( 'NONE', ( #145202 ), #161382, .F. ) ;
#195141=CARTESIAN_POINT ( 'NONE',  ( 24.86035471869053382, 4.680034064337423416, 169.8578160361099094 ) ) ;
#195223=EDGE_LOOP ( 'NONE', ( #94617, #8271, #52516, #20353, #158392 ) ) ;
#195233=CARTESIAN_POINT ( 'NONE',  ( -27.93385843979426397, 7.419916809875860331, 160.9064084702653190 ) ) ;
#195259=ORIENTED_EDGE ( 'NONE', *, *, #105010, .T. ) ;
#195273=CARTESIAN_POINT ( 'NONE',  ( 28.79475375365586132, 2.781246896534039337E-14, 144.9843446568999923 ) ) ;
#195313=CARTESIAN_POINT ( 'NONE',  ( -23.31738231874055600, 16.94106989632528837, 142.0500000054623513 ) ) ;
#195316=ORIENTED_EDGE ( 'NONE', *, *, #175002, .T. ) ;
#195326=CARTESIAN_POINT ( 'NONE',  ( -17.14385361876520975, 23.59649016807275856, 143.0750000027311444 ) ) ;
#195384=DIRECTION ( 'NONE',  ( -0.000000000000000000, -0.000000000000000000, -1.000000000000000000 ) ) ;
#195396=DIRECTION ( 'NONE',  ( -0.9945218953682734009, 0.000000000000000000, 0.1045284632676528741 ) ) ;
#195397=CARTESIAN_POINT ( 'NONE',  ( -25.62062145120080814, 9.171473787276466894, 171.1688781158127028 ) ) ;
#195442=CARTESIAN_POINT ( 'NONE',  ( 25.75939503182846479, 8.559839547494778600, 171.7912139782359304 ) ) ;
#195456=CARTESIAN_POINT ( 'NONE',  ( -8.571926809382608425, 26.38167802310805854, 140.9750000027312069 ) ) ;
#195541=DIRECTION ( 'NONE',  ( 0.000000000000000000, 0.000000000000000000, 1.000000000000000000 ) ) ;
#195567=VECTOR ( 'NONE', #127304, 1000.000000000000000 ) ;
#195615=CARTESIAN_POINT ( 'NONE',  ( 17.14385361876520264, 23.59649016807275856, 148.1750000027311671 ) ) ;
#195807=CARTESIAN_POINT ( 'NONE',  ( -22.44159573604010305, 16.30477369853692338, 149.1750000027311671 ) ) ;
#195847=CARTESIAN_POINT ( 'NONE',  ( 24.06756124613666614, -8.142616467493763110, 169.4332804344608974 ) ) ;
#196049=CARTESIAN_POINT ( 'NONE',  ( -21.38418241377623374, -7.427326039334300134, 174.4773576836617224 ) ) ;
#196248=CARTESIAN_POINT ( 'NONE',  ( 29.17999648465608686, -8.032454009542489004, 149.7954620931811291 ) ) ;
#196262=DIRECTION ( 'NONE',  ( -0.5367108174878558735, -0.8437662581494460579, 0.000000000000000000 ) ) ;
#196321=DIRECTION ( 'NONE',  ( 1.000000000000000000, 0.000000000000000000, 0.000000000000000000 ) ) ;
#196323=CARTESIAN_POINT ( 'NONE',  ( -28.82186960331499392, 9.364793116373565596, 142.1500000054623740 ) ) ;
#196403=CARTESIAN_POINT ( 'NONE',  ( 9.611906137939470796, -26.05071838941950801, 139.9999999999999716 ) ) ;
#196458=CARTESIAN_POINT ( 'NONE',  ( 1.993301997531345292E-15, -30.30510711980685912, 146.5000000000000000 ) ) ;
#196591=CARTESIAN_POINT ( 'NONE',  ( -24.30454888808800717, 2.781629622375083599, 174.5654150192188183 ) ) ;
#196608=CARTESIAN_POINT ( 'NONE',  ( 22.44159573604009239, 16.30477369853692693, 148.0750000027312012 ) ) ;
#196621=CARTESIAN_POINT ( 'NONE',  ( -3.573655867282028392E-15, 2.428612866367529932E-14, 150.0000000000000000 ) ) ;
#196747=CARTESIAN_POINT ( 'NONE',  ( 20.96276500525451070, -10.40013546722648030, 168.2886347277376160 ) ) ;
#196838=CARTESIAN_POINT ( 'NONE',  ( -23.03403192006591382, -14.65170476119024556, 170.0000000000000000 ) ) ;
#196970=EDGE_CURVE ( 'NONE', #90049, #177604, #182305, .T. ) ;
#196998=( BOUNDED_CURVE ( )  B_SPLINE_CURVE ( 2, ( #129759, #67114, #96445, #6426, #36764, #50959, #114608, #8447, #53951, #115627, #38787 ),
 .UNSPECIFIED., .F., .T. ) 
 B_SPLINE_CURVE_WITH_KNOTS ( ( 3, 2, 2, 2, 2, 3 ),
 ( 0.4000000000000003553, 0.4200000000000003730, 0.4400000000000003353, 0.4600000000000003531, 0.4800000000000004263, 0.5000000000000004441 ),
 .UNSPECIFIED. ) 
 CURVE ( )  GEOMETRIC_REPRESENTATION_ITEM ( )  RATIONAL_B_SPLINE_CURVE ( ( 0.9999999999999992228, 0.9510565162951543083, 1.000000000000000000, 0.9510565162951535312, 1.000000000000000000, 0.9510565162951535312, 1.000000000000000000, 0.9510565162951535312, 1.000000000000000000, 0.9510565162951524210, 1.000000000000001110 ) ) 
 REPRESENTATION_ITEM ( '' )  );
#197010=AXIS2_PLACEMENT_3D ( 'NONE', #198328, #123446, #91118 ) ;
#197036=CARTESIAN_POINT ( 'NONE',  ( -21.57728377622141380, -10.02787190051640742, 170.5958156194641617 ) ) ;
#197138=CARTESIAN_POINT ( 'NONE',  ( -8.571926809382608425, 26.38167802310805854, 146.4750000027311785 ) ) ;
#197225=CARTESIAN_POINT ( 'NONE',  ( 17.79613651744293534, 24.49428055684532524, 141.2843446568999752 ) ) ;
#197227=CARTESIAN_POINT ( 'NONE',  ( -27.20489923017578704, 7.754340368643402925, 164.3890803562166809 ) ) ;
#197298=CARTESIAN_POINT ( 'NONE',  ( -3.573655867282028392E-15, 2.428612866367529932E-14, 155.0000000000000000 ) ) ;
#197299=CARTESIAN_POINT ( 'NONE',  ( 27.73933785331498569, 2.768321779492822058E-14, 143.8750000027311842 ) ) ;
#197302=ORIENTED_EDGE ( 'NONE', *, *, #134775, .T. ) ;
#197367=LINE ( 'NONE', #70025, #40849 ) ;
#197381=CARTESIAN_POINT ( 'NONE',  ( -21.92083080610932910, 8.096106818377439396, 172.4353877980870493 ) ) ;
#197423=CARTESIAN_POINT ( 'NONE',  ( 26.61723430050332340, 3.645106422946821301, 172.4622069319858895 ) ) ;
#197436=CARTESIAN_POINT ( 'NONE',  ( -8.571926809382601320, -26.38167802310801591, 139.7750000027311899 ) ) ;
#197535=CARTESIAN_POINT ( 'NONE',  ( -24.72709851008508508, -6.869189314505666388, 167.7661538690216787 ) ) ;
#197586=CARTESIAN_POINT ( 'NONE',  ( -22.44159573604010305, 16.30477369853692338, 146.6750000027311671 ) ) ;
#197710=ORIENTED_EDGE ( 'NONE', *, *, #171523, .F. ) ;
#197722=CARTESIAN_POINT ( 'NONE',  ( 21.44820451018246388, -9.431764332217083435, 168.6453917704523633 ) ) ;
#197777=CARTESIAN_POINT ( 'NONE',  ( 22.44159573604009594, -16.30477369853687364, 144.1750000027311671 ) ) ;
#197781=CARTESIAN_POINT ( 'NONE',  ( 17.14385361876520264, 23.59649016807275856, 146.6750000027311671 ) ) ;
#197818=CARTESIAN_POINT ( 'NONE',  ( -21.70479006154309687, -9.754118203517077035, 170.7545476126475421 ) ) ;
#197889=ORIENTED_EDGE ( 'NONE', *, *, #168410, .F. ) ;
#197994=ADVANCED_FACE ( 'NONE', ( #13216 ), #136541, .T. ) ;
#198122=CARTESIAN_POINT ( 'NONE',  ( -27.73933785331498925, -9.013057229001049109, 142.9750000027312069 ) ) ;
#198207=CARTESIAN_POINT ( 'NONE',  ( -27.91261209101616458, 7.473227146837950308, 160.9450349587949063 ) ) ;
#198230=ORIENTED_EDGE ( 'NONE', *, *, #66504, .F. ) ;
#198278=DIRECTION ( 'NONE',  ( 0.000000000000000000, 0.000000000000000000, -1.000000000000000000 ) ) ;
#198279=CARTESIAN_POINT ( 'NONE',  ( 27.73933785331498214, 9.013057229001095294, 141.9750000027311501 ) ) ;
#198311=CARTESIAN_POINT ( 'NONE',  ( 25.51181203389338137, 5.285008086477808398, 165.5623613760384956 ) ) ;
#198315=ORIENTED_EDGE ( 'NONE', *, *, #49797, .F. ) ;
#198320=DIRECTION ( 'NONE',  ( 1.000000000000000000, 0.000000000000000000, -0.000000000000000000 ) ) ;
#198328=CARTESIAN_POINT ( 'NONE',  ( 19.49401214000076976, 12.39993551617566681, 164.9999999999999716 ) ) ;
#198361=CARTESIAN_POINT ( 'NONE',  ( 10.13896110635529446, -25.83826727361345021, 139.9999999999999716 ) ) ;
#198417=CARTESIAN_POINT ( 'NONE',  ( 1.993301997531345292E-15, -30.30510711980685912, 144.4999999999999432 ) ) ;
#198436=CARTESIAN_POINT ( 'NONE',  ( -23.29544513554941076, 16.92513159979227666, 144.0656553485623874 ) ) ;
#198444=DIRECTION ( 'NONE',  ( 1.000000000000000000, -0.000000000000000000, -0.000000000000000000 ) ) ;
#198521=AXIS2_PLACEMENT_3D ( 'NONE', #39390, #99044, #83875 ) ;
#198522=CARTESIAN_POINT ( 'NONE',  ( -24.50238749460122989, -2.981321037228370052, 173.3223451563238200 ) ) ;
#198543=VECTOR ( 'NONE', #67009, 1000.000000000000000 ) ;
#198563=CARTESIAN_POINT ( 'NONE',  ( -25.12471020271278732, -7.795852113654130555, 170.9710663016989258 ) ) ;
#198604=CARTESIAN_POINT ( 'NONE',  ( -28.79475375365568013, -9.355982642739451904, 148.0843446568999866 ) ) ;
#198716=CARTESIAN_POINT ( 'NONE',  ( -27.19095269391954517, 10.02149780027903780, 149.7954620931811291 ) ) ;
#198724=CARTESIAN_POINT ( 'NONE',  ( -3.573655867282028392E-15, 2.428612866367529932E-14, 150.0000000000000000 ) ) ;
#198734=VECTOR ( 'NONE', #139733, 1000.000000000000000 ) ;
#198772=CARTESIAN_POINT ( 'NONE',  ( -22.44159573604009950, -16.30477369853688430, 145.5750000027311728 ) ) ;
#198776=CARTESIAN_POINT ( 'NONE',  ( -17.14385361876520619, 23.59649016807275856, 143.0750000027311444 ) ) ;
#198809=LINE ( 'NONE', #60274, #37044 ) ;
#198812=CARTESIAN_POINT ( 'NONE',  ( -24.18299921989768109, -12.77492350451736947, 169.7822198539309966 ) ) ;
#198948=CARTESIAN_POINT ( 'NONE',  ( -21.85375568585902428, 8.111533062293290186, 169.4628294566284410 ) ) ;
#198959=CARTESIAN_POINT ( 'NONE',  ( -14.71622889490178920, 24.64770729138309591, 139.9999999999999716 ) ) ;
#199029=CARTESIAN_POINT ( 'NONE',  ( 23.27014359241642438, -11.64952062020058499, 165.7333947824558891 ) ) ;
#199085=CARTESIAN_POINT ( 'NONE',  ( 8.898068258721473001, -27.38543819252872069, 142.5843446569000150 ) ) ;
#199109=CARTESIAN_POINT ( 'NONE',  ( -17.14385361876520619, 23.59649016807275856, 144.5750000027312012 ) ) ;
#199141=EDGE_CURVE ( 'NONE', #155416, #116956, #52924, .T. ) ;
#199161=ORIENTED_EDGE ( 'NONE', *, *, #164239, .F. ) ;
#199274=DIRECTION ( 'NONE',  ( -1.000000000000000000, 0.000000000000000000, 0.000000000000000000 ) ) ;
#199275=CARTESIAN_POINT ( 'NONE',  ( 27.73933785331498925, -9.013057229001033122, 143.7750000027311614 ) ) ;
#199358=CARTESIAN_POINT ( 'NONE',  ( -16.25332922912272693, -23.18555326879971190, 140.0000000000000284 ) ) ;
#199400=CARTESIAN_POINT ( 'NONE',  ( 25.76143648877207681, 7.343476467569183264, 174.8772314887149264 ) ) ;
#199415=CARTESIAN_POINT ( 'NONE',  ( 17.81289503416611453, -24.51734667627695785, 144.6999999999999886 ) ) ;
#199466=DIRECTION ( 'NONE',  ( -1.000000000000000000, 0.000000000000000000, 0.000000000000000000 ) ) ;
#199513=CARTESIAN_POINT ( 'NONE',  ( -21.84611564451295962, -8.148379233835273183, 169.4346228884814707 ) ) ;
#199519=VERTEX_POINT ( 'NONE', #177844 ) ;
#199576=B_SPLINE_CURVE_WITH_KNOTS ( 'NONE', 3,
 ( #19732, #4536, #78405, #66229, #35888, #188600, #16757, #96554 ),
 .UNSPECIFIED., .F., .F.,
 ( 4, 2, 2, 4 ),
 ( 0.03534151991400943243, 0.03926041079282514140, 0.04121985623223303058, 0.04317930167164092670 ),
 .UNSPECIFIED. ) ;
#199592=CARTESIAN_POINT ( 'NONE',  ( 28.79475375365586132, 2.781246896534039337E-14, 148.9843446568999923 ) ) ;
#199605=CARTESIAN_POINT ( 'NONE',  ( 22.94331271462294097, 3.784814030245898575, 190.0000000000000000 ) ) ;
#199681=CARTESIAN_POINT ( 'NONE',  ( 22.06725540229016502, -16.90544345524162395, 140.0000000000001421 ) ) ;
#199705=EDGE_CURVE ( 'NONE', #144934, #93307, #192011, .T. ) ;
#199761=CARTESIAN_POINT ( 'NONE',  ( 17.14385361876520264, -23.59649016807271238, 144.0750000027311444 ) ) ;
#199765=CARTESIAN_POINT ( 'NONE',  ( 27.73933785331498214, 9.013057229001095294, 148.4750000027311785 ) ) ;
#199802=CARTESIAN_POINT ( 'NONE',  ( -25.47140278216090081, -9.703455644540127878, 170.7619267275368600 ) ) ;
#200004=CARTESIAN_POINT ( 'NONE',  ( -21.16427095311448880, 10.71512246325695372, 170.2843762835011319 ) ) ;
#200042=CARTESIAN_POINT ( 'NONE',  ( -21.56952297831560372, 5.557039098534931831, 173.4609804364286276 ) ) ;
#200103=CARTESIAN_POINT ( 'NONE',  ( 22.44159573604009594, -16.30477369853687364, 147.6750000027311671 ) ) ;
#200166=VECTOR ( 'NONE', #47631, 1000.000000000000000 ) ;
#200191=CARTESIAN_POINT ( 'NONE',  ( -26.47570757000579533, -8.223507928023325420, 167.6031463996532977 ) ) ;
ENDSEC;
END-ISO-10303-21;
